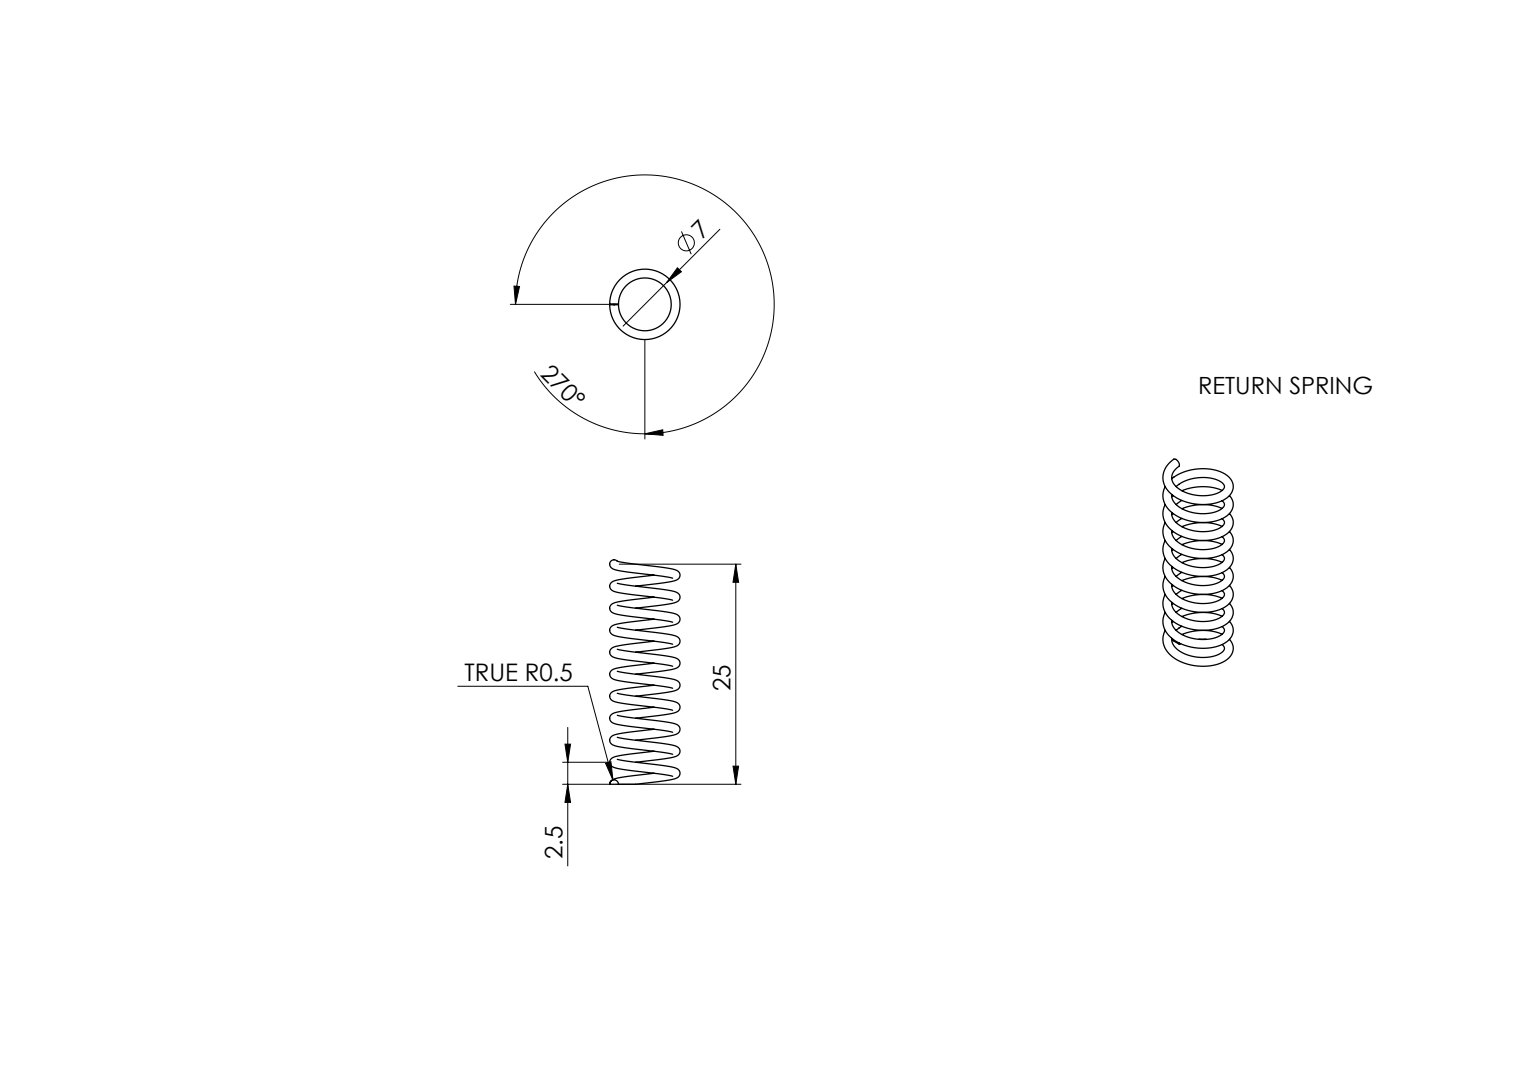
ISO-10303-21;
HEADER;
FILE_DESCRIPTION (('STEP AP214'),
    '1' );
FILE_NAME ('Return Spring.step',
    '2026-10-25T16:39:07',
    ( '' ),
    ( '' ),
    'SwSTEP 2.0',
    'SolidWorks 2026',
    '' );
FILE_SCHEMA (( 'AUTOMOTIVE_DESIGN' ));
ENDSEC;

DATA;
#1=CARTESIAN_POINT ( 'NONE',  ( 1.444289557195957086, 32.75319992234354061, -4.262301884875733471 ) ) ;
#6=CARTESIAN_POINT ( 'NONE',  ( 3.518350579753631191, 24.37180007765648071, 1.080741659609802285 ) ) ;
#9=CARTESIAN_POINT ( 'NONE',  ( -1.336863392178478716, 22.49680007765647360, 4.297206761780677731 ) ) ;
#14=CARTESIAN_POINT ( 'NONE',  ( -2.115076519116362519, 25.12180007765647360, 3.012182706137107147 ) ) ;
#21=CARTESIAN_POINT ( 'NONE',  ( 3.518350579753605434, 18.12819992234353705, -1.080741659609877114 ) ) ;
#23=CARTESIAN_POINT ( 'NONE',  ( -2.798362969681365886, 35.24680007765648071, 2.102939460078824929 ) ) ;
#24=CARTESIAN_POINT ( 'NONE',  ( 0.05938372350920109732, 27.62819992234353705, -3.680117784833935701 ) ) ;
#39=CARTESIAN_POINT ( 'NONE',  ( -2.518350579753611207, 21.87819992234354416, 0.7558219633769609480 ) ) ;
#47=CARTESIAN_POINT ( 'NONE',  ( 0.05938372350927906274, 32.37180007765647360, 3.680117784833935701 ) ) ;
#58=CARTESIAN_POINT ( 'NONE',  ( 2.055738996568313048, 21.99680007765648426, 1.423772053676023441 ) ) ;
#65=CARTESIAN_POINT ( 'NONE',  ( 0.8262555684460829442, 37.75319992234354771, -2.360188852285421302 ) ) ;
#69=CARTESIAN_POINT ( 'NONE',  ( 4.518350579753633411, 31.87180007765647716, 1.405661355842698468 ) ) ;
#87=CARTESIAN_POINT ( 'NONE',  ( 4.499999999999999112, 18.25319992234354771, 0.05647727720528474687 ) ) ;
#88=CARTESIAN_POINT ( 'NONE',  ( -2.115076519116425580, 27.37819992234354771, -3.012182706137063182 ) ) ;
#90=CARTESIAN_POINT ( 'NONE',  ( -1.593127413382998459, 35.87180007765648071, -2.091722143975139669 ) ) ;
#92=CARTESIAN_POINT ( 'NONE',  ( 2.733110507866328920, 36.12819992234354771, 3.862833514489095510 ) ) ;
#96=CARTESIAN_POINT ( 'NONE',  ( 2.798362969681366330, 18.99680007765648071, -2.102939460078824929 ) ) ;
#99=CARTESIAN_POINT ( 'NONE',  ( 4.518350579753633411, 21.87180007765647360, 1.405661355842698468 ) ) ;
#106=CARTESIAN_POINT ( 'NONE',  ( -3.500000000000000444, 22.99680007765647716, 0.05647727720536892260 ) ) ;
#111=CARTESIAN_POINT ( 'NONE',  ( -3.481649420246394122, 22.12819992234353705, -1.193696214020467883 ) ) ;
#113=CARTESIAN_POINT ( 'NONE',  ( 2.211161402132902243, 37.12180007765645939, 2.942372952327172442 ) ) ;
#114=CARTESIAN_POINT ( 'NONE',  ( 1.027846397803612311, 36.25319992234354771, 3.346150245485499219 ) ) ;
#126=CARTESIAN_POINT ( 'NONE',  ( -0.05938372350921170689, 21.37819992234354416, 2.628655560595669183 ) ) ;
#134=CARTESIAN_POINT ( 'NONE',  ( -0.05938372350927861171, 36.12180007765648782, -3.680117784833935701 ) ) ;
#147=CARTESIAN_POINT ( 'NONE',  ( 1.593127413382998903, 24.62180007765647716, 2.091722143975139669 ) ) ;
#149=CARTESIAN_POINT ( 'NONE',  ( 2.115076519116362963, 23.87180007765647360, -3.012182706137107591 ) ) ;
#154=CARTESIAN_POINT ( 'NONE',  ( -0.05938372350921170689, 33.87819992234354061, 2.628655560595669183 ) ) ;
#158=CARTESIAN_POINT ( 'NONE',  ( -3.607379964056306676, 35.24680007765647360, 2.690724712371306282 ) ) ;
#173=CARTESIAN_POINT ( 'NONE',  ( 2.733110507866328920, 21.12819992234354416, 3.862833514489095510 ) ) ;
#174=CARTESIAN_POINT ( 'NONE',  ( -2.211161402132838738, 26.62819992234354416, 2.942372952327218183 ) ) ;
#176=CARTESIAN_POINT ( 'NONE',  ( -1.989345975306426206, 40.24680007765648071, 1.515154207786343799 ) ) ;
#178=CARTESIAN_POINT ( 'NONE',  ( 0.05938372350919016857, 32.62819992234354771, -4.731580009072201776 ) ) ;
#182=CARTESIAN_POINT ( 'NONE',  ( -2.798362969681365886, 30.24680007765648071, 2.102939460078824929 ) ) ;
#187=CARTESIAN_POINT ( 'NONE',  ( 4.518350579753633411, 34.37180007765647360, 1.405661355842698468 ) ) ;
#191=CARTESIAN_POINT ( 'NONE',  ( -2.115076519116362519, 27.62180007765648071, 3.012182706137107147 ) ) ;
#197=CARTESIAN_POINT ( 'NONE',  ( 2.115076519116426024, 21.12819992234353705, 3.012182706137062294 ) ) ;
#200=CARTESIAN_POINT ( 'NONE',  ( -3.481649420246369697, 37.87180007765648071, 1.193696214020542490 ) ) ;
#202=CARTESIAN_POINT ( 'NONE',  ( -0.05938372350920063936, 31.37819992234354416, 3.680117784833935701 ) ) ;
#216=CARTESIAN_POINT ( 'NONE',  ( -1.086818808809129289, 15.00000000000000533, -3.240250934315705322 ) ) ;
#219=CARTESIAN_POINT ( 'NONE',  ( 0.8262555684460829442, 20.25319992234354771, -2.360188852285421302 ) ) ;
#222=CARTESIAN_POINT ( 'NONE',  ( -1.444289557196047014, 18.49680007765647360, -4.262301884875704161 ) ) ;
#229=CARTESIAN_POINT ( 'NONE',  ( -0.05938372350927861171, 31.12180007765647005, -3.680117784833935701 ) ) ;
#239=PLANE ( 'NONE',  #7419 ) ;
#242=CARTESIAN_POINT ( 'NONE',  ( 2.518350579753628971, 21.87180007765647360, 0.7558219633769073242 ) ) ;
#245=CARTESIAN_POINT ( 'NONE',  ( 0.05938372350927906967, 19.87180007765648071, 3.680117784833935701 ) ) ;
#249=CARTESIAN_POINT ( 'NONE',  ( 0.7188294034286553114, 33.75319992234354771, 2.395093729190349130 ) ) ;
#252=CARTESIAN_POINT ( 'NONE',  ( -2.733110507866247652, 32.62180007765647360, 3.862833514489154574 ) ) ;
#272=( NAMED_UNIT ( * ) SI_UNIT ( $, .STERADIAN. ) SOLID_ANGLE_UNIT ( ) );
#274=CARTESIAN_POINT ( 'NONE',  ( 3.607379964056363075, 18.50319992234354416, 2.690724712371229010 ) ) ;
#275=CARTESIAN_POINT ( 'NONE',  ( -2.864755990943222308, 26.75319992234354771, 2.011557305968548093 ) ) ;
#277=CARTESIAN_POINT ( 'NONE',  ( 2.518350579753628971, 34.37180007765647360, 0.7558219633769073242 ) ) ;
#279=CARTESIAN_POINT ( 'NONE',  ( 2.829195390882724759, 35.37819992234354061, -3.793023760679264278 ) ) ;
#284=CARTESIAN_POINT ( 'NONE',  ( 2.864755990943265829, 31.99680007765647716, 2.011557305968487697 ) ) ;
#289=CARTESIAN_POINT ( 'NONE',  ( -2.733110507866247652, 27.62180007765647716, 3.862833514489154574 ) ) ;
#293=CARTESIAN_POINT ( 'NONE',  ( 3.518350579753631191, 24.37180007765648071, 1.080741659609802285 ) ) ;
#298=CARTESIAN_POINT ( 'NONE',  ( -1.027846397803611866, 20.00319992234354416, -3.346150245485499219 ) ) ;
#301=CARTESIAN_POINT ( 'NONE',  ( 2.055738996568313048, 16.99680007765648071, 1.423772053676023441 ) ) ;
#303=CARTESIAN_POINT ( 'NONE',  ( 2.115076519116426024, 36.12819992234355482, 3.012182706137062294 ) ) ;
#318=CARTESIAN_POINT ( 'NONE',  ( 0.8262555684460829442, 17.75319992234354061, -2.360188852285421302 ) ) ;
#322=CARTESIAN_POINT ( 'NONE',  ( -1.336863392178478716, 17.49680007765647716, 4.297206761780677731 ) ) ;
#328=CARTESIAN_POINT ( 'NONE',  ( -2.864755990943265829, 38.24680007765647360, -2.011557305968488141 ) ) ;
#341=CARTESIAN_POINT ( 'NONE',  ( 0.7188294034286049072, 26.24680007765647716, -2.395093729190366005 ) ) ;
#344=CARTESIAN_POINT ( 'NONE',  ( 3.518350579753631191, 19.37180007765648071, 1.080741659609802729 ) ) ;
#348=CARTESIAN_POINT ( 'NONE',  ( -2.864755990943222308, 16.75319992234354416, 2.011557305968548093 ) ) ;
#351=CARTESIAN_POINT ( 'NONE',  ( -1.336863392178478716, 32.49680007765647360, 4.297206761780677731 ) ) ;
#360=ORIENTED_EDGE ( 'NONE', *, *, #444, .T. ) ;
#368=CARTESIAN_POINT ( 'NONE',  ( -3.607379964056363075, 24.75319992234354416, -2.690724712371229899 ) ) ;
#369=CARTESIAN_POINT ( 'NONE',  ( 2.798362969681409851, 26.00319992234354771, 2.102939460078764977 ) ) ;
#370=CARTESIAN_POINT ( 'NONE',  ( -2.518350579753611207, 19.37819992234354771, 0.7558219633769609480 ) ) ;
#372=CARTESIAN_POINT ( 'NONE',  ( -1.444289557195956863, 31.50319992234354416, 4.262301884875733471 ) ) ;
#379=EDGE_CURVE ( 'NONE', #12310, #9517, #6444, .T. ) ;
#380=CARTESIAN_POINT ( 'NONE',  ( 3.518350579753631191, 31.87180007765647716, 1.080741659609802285 ) ) ;
#384=CARTESIAN_POINT ( 'NONE',  ( 1.444289557196047680, 32.24680007765647360, 4.262301884875704161 ) ) ;
#388=CARTESIAN_POINT ( 'NONE',  ( 3.500000000000000444, 31.74680007765647716, -0.05647727720536935281 ) ) ;
#395=CARTESIAN_POINT ( 'NONE',  ( -2.211161402132839182, 26.62819992234353705, 2.942372952327218627 ) ) ;
#398=CARTESIAN_POINT ( 'NONE',  ( 3.481649420246369697, 36.62180007765648071, -1.193696214020541824 ) ) ;
#399=CARTESIAN_POINT ( 'NONE',  ( 3.518350579753605434, 33.12819992234354771, -1.080741659609877114 ) ) ;
#415=CARTESIAN_POINT ( 'NONE',  ( -0.05938372350921170689, 23.87819992234354416, 2.628655560595669183 ) ) ;
#417=CARTESIAN_POINT ( 'NONE',  ( 3.481649420246369697, 16.62180007765648071, -1.193696214020541824 ) ) ;
#422=CARTESIAN_POINT ( 'NONE',  ( 1.027846397803542144, 38.74680007765647360, -3.346150245485522312 ) ) ;
#424=DIRECTION ( 'NONE',  ( 1.027440012549754468E-14, -0.1129545544106655003, 0.9936001553129347741 ) ) ;
#431=CARTESIAN_POINT ( 'NONE',  ( -1.593127413382998459, 25.87180007765647716, -2.091722143975139669 ) ) ;
#433=CARTESIAN_POINT ( 'NONE',  ( 2.211161402132902243, 24.62180007765647716, 2.942372952327172442 ) ) ;
#437=CARTESIAN_POINT ( 'NONE',  ( -1.027846397803611866, 22.50319992234354416, -3.346150245485499219 ) ) ;
#441=CARTESIAN_POINT ( 'NONE',  ( -3.518350579753630747, 18.12180007765648071, -1.080741659609802729 ) ) ;
#444=EDGE_CURVE ( 'NONE', #6995, #13000, #16882, .T. ) ;
#460=CARTESIAN_POINT ( 'NONE',  ( -0.05938372350918959958, 28.87819992234354416, 4.731580009072201776 ) ) ;
#461=CARTESIAN_POINT ( 'NONE',  ( -2.115076519116425580, 24.87819992234354416, -3.012182706137063182 ) ) ;
#462=CARTESIAN_POINT ( 'NONE',  ( -2.500000000000001332, 22.00319992234354771, -0.05647727720530596601 ) ) ;
#464=CARTESIAN_POINT ( 'NONE',  ( -4.481649420246366589, 17.87180007765647360, 1.518615910253458878 ) ) ;
#468=CARTESIAN_POINT ( 'NONE',  ( 2.798362969681366330, 26.49680007765648071, -2.102939460078824929 ) ) ;
#471=CARTESIAN_POINT ( 'NONE',  ( -1.336863392178478716, 32.49680007765647360, 4.297206761780677731 ) ) ;
#475=CARTESIAN_POINT ( 'NONE',  ( 2.115076519116362963, 28.87180007765647716, -3.012182706137107147 ) ) ;
#480=( NAMED_UNIT ( * ) PLANE_ANGLE_UNIT ( ) SI_UNIT ( $, .RADIAN. ) );
#482=CARTESIAN_POINT ( 'NONE',  ( 0.05938372350920109732, 30.12819992234354416, -3.680117784833935701 ) ) ;
#486=CARTESIAN_POINT ( 'NONE',  ( 1.497042530366477164, 18.87180007765648071, -2.161531897785062384 ) ) ;
#487=CARTESIAN_POINT ( 'NONE',  ( 3.673772985318163098, 18.00319992234354416, -2.599342558261029001 ) ) ;
#504=CARTESIAN_POINT ( 'NONE',  ( -2.518350579753611207, 26.87819992234354416, 0.7558219633769609480 ) ) ;
#509=CARTESIAN_POINT ( 'NONE',  ( -2.798362969681365886, 20.24680007765647716, 2.102939460078824929 ) ) ;
#525=CARTESIAN_POINT ( 'NONE',  ( 1.497042530366477164, 33.87180007765647360, -2.161531897785062384 ) ) ;
#527=CARTESIAN_POINT ( 'NONE',  ( -2.115076519116362519, 25.12180007765647005, 3.012182706137108035 ) ) ;
#532=CARTESIAN_POINT ( 'NONE',  ( 1.027846397803612311, 18.75319992234354771, 3.346150245485499219 ) ) ;
#535=CARTESIAN_POINT ( 'NONE',  ( -2.864755990943265829, 18.24680007765648071, -2.011557305968488141 ) ) ;
#539=CLOSED_SHELL ( 'NONE', ( #14555, #17882, #8237, #2719, #9820 ) ) ;
#558=CARTESIAN_POINT ( 'NONE',  ( 4.499999999999999112, 23.25319992234354416, 0.05647727720528474687 ) ) ;
#559=CARTESIAN_POINT ( 'NONE',  ( -2.115076519116425580, 37.37819992234353350, -3.012182706137063182 ) ) ;
#561=CARTESIAN_POINT ( 'NONE',  ( -2.481649420246391902, 19.62819992234354416, -0.8687765177875723666 ) ) ;
#564=CARTESIAN_POINT ( 'NONE',  ( 3.673772985318219053, 19.49680007765647005, 2.599342558260951730 ) ) ;
#569=CARTESIAN_POINT ( 'NONE',  ( -3.481649420246369697, 32.87180007765645939, 1.193696214020542490 ) ) ;
#572=CARTESIAN_POINT ( 'NONE',  ( 4.518350579753633411, 29.37180007765647716, 1.405661355842698468 ) ) ;
#582=CARTESIAN_POINT ( 'NONE',  ( -3.500000000000000444, 24.50319992234354416, -0.05647727720529563400 ) ) ;
#585=CARTESIAN_POINT ( 'NONE',  ( 2.500000000000001332, 24.24680007765647716, -0.05647727720535888202 ) ) ;
#586=CARTESIAN_POINT ( 'NONE',  ( -3.673772985318163098, 16.75319992234354416, 2.599342558261029001 ) ) ;
#602=CARTESIAN_POINT ( 'NONE',  ( -1.497042530366522461, 27.37819992234355126, -2.161531897785030409 ) ) ;
#605=CARTESIAN_POINT ( 'NONE',  ( 0.05938372350927906274, 24.87180007765647005, 3.680117784833935701 ) ) ;
#622=CARTESIAN_POINT ( 'NONE',  ( -2.518350579753628526, 28.12180007765647716, -0.7558219633769075463 ) ) ;
#624=CARTESIAN_POINT ( 'NONE',  ( 2.211161402132902243, 27.12180007765647716, 2.942372952327172442 ) ) ;
#629=CARTESIAN_POINT ( 'NONE',  ( 3.481649420246394122, 20.87819992234354416, 1.193696214020467439 ) ) ;
#633=CARTESIAN_POINT ( 'NONE',  ( 3.500000000000000444, 16.74680007765647716, -0.05647727720536935281 ) ) ;
#650=CARTESIAN_POINT ( 'NONE',  ( -4.499999999999999112, 29.50319992234354061, -0.05647727720528529505 ) ) ;
#651=CARTESIAN_POINT ( 'NONE',  ( -2.115076519116425580, 32.37819992234354771, -3.012182706137063182 ) ) ;
#652=CARTESIAN_POINT ( 'NONE',  ( -0.05938372350921170689, 23.87819992234354416, 2.628655560595669183 ) ) ;
#655=CARTESIAN_POINT ( 'NONE',  ( -1.444289557196047014, 15.99680007765647716, -4.262301884875704161 ) ) ;
#659=CARTESIAN_POINT ( 'NONE',  ( 3.518350579753631191, 36.87180007765645939, 1.080741659609802285 ) ) ;
#672=CARTESIAN_POINT ( 'NONE',  ( -1.027846397803611866, 30.00319992234354416, -3.346150245485499219 ) ) ;
#675=CARTESIAN_POINT ( 'NONE',  ( 2.481649420246374138, 19.12180007765648071, -0.8687765177876252132 ) ) ;
#677=CARTESIAN_POINT ( 'NONE',  ( -2.829195390882724315, 21.62819992234354416, 3.793023760679264722 ) ) ;
#683=CARTESIAN_POINT ( 'NONE',  ( -4.499999999999999112, 37.99680007765646650, 0.05647727720537927543 ) ) ;
#696=CARTESIAN_POINT ( 'NONE',  ( 0.7188294034286553114, 26.25319992234354416, 2.395093729190349130 ) ) ;
#698=CARTESIAN_POINT ( 'NONE',  ( 1.135272562821090458, 19.74680007765648071, 3.311245368580554072 ) ) ;
#711=CARTESIAN_POINT ( 'NONE',  ( 1.497042530366477164, 28.87180007765648426, -2.161531897785062384 ) ) ;
#713=CARTESIAN_POINT ( 'NONE',  ( 1.027846397803542144, 31.24680007765647716, -3.346150245485522312 ) ) ;
#722=CARTESIAN_POINT ( 'NONE',  ( -1.336863392178478716, 39.99680007765647360, 4.297206761780677731 ) ) ;
#743=CARTESIAN_POINT ( 'NONE',  ( 3.673772985318163098, 25.50319992234354416, -2.599342558261029001 ) ) ;
#744=CARTESIAN_POINT ( 'NONE',  ( -2.211161402132838738, 39.12819992234354771, 2.942372952327218183 ) ) ;
#745=CARTESIAN_POINT ( 'NONE',  ( 1.593127413382953383, 17.87819992234354416, -2.091722143975172532 ) ) ;
#747=CARTESIAN_POINT ( 'NONE',  ( 1.444289557195957086, 37.75319992234354771, -4.262301884875733471 ) ) ;
#751=CARTESIAN_POINT ( 'NONE',  ( 3.518350579753631191, 34.37180007765648071, 1.080741659609802285 ) ) ;
#763=CARTESIAN_POINT ( 'NONE',  ( -1.027846397803611866, 25.00319992234354416, -3.346150245485499219 ) ) ;
#766=CARTESIAN_POINT ( 'NONE',  ( -2.518350579753628526, 25.62180007765648426, -0.7558219633769075463 ) ) ;
#767=CARTESIAN_POINT ( 'NONE',  ( 4.499999999999999112, 15.75319992234354416, 0.05647727720528474687 ) ) ;
#771=CARTESIAN_POINT ( 'NONE',  ( 1.027846397803542144, 16.24680007765647716, -3.346150245485522312 ) ) ;
#782=CARTESIAN_POINT ( 'NONE',  ( -2.481649420246391902, 29.62819992234354416, -0.8687765177875723666 ) ) ;
#784=CARTESIAN_POINT ( 'NONE',  ( -2.864755990943265829, 25.74680007765647716, -2.011557305968488141 ) ) ;
#791=DIRECTION ( 'NONE',  ( -1.028113302204112171E-14, 0.1129545544106649313, -0.9936001553129349961 ) ) ;
#799=CARTESIAN_POINT ( 'NONE',  ( -1.593127413382998459, 28.37180007765648426, -2.091722143975139669 ) ) ;
#801=CARTESIAN_POINT ( 'NONE',  ( 3.481649420246370141, 26.62180007765648071, -1.193696214020541602 ) ) ;
#805=CARTESIAN_POINT ( 'NONE',  ( -3.500000000000000444, 40.00000000000000711, 3.664603343001004987E-14 ) ) ;
#808=CARTESIAN_POINT ( 'NONE',  ( -3.518350579753630747, 25.62180007765648071, -1.080741659609802729 ) ) ;
#818=EDGE_CURVE ( 'NONE', #6875, #12310, #1742, .T. ) ;
#823=CARTESIAN_POINT ( 'NONE',  ( 3.500000000000000444, 34.24680007765648071, -0.05647727720536935281 ) ) ;
#829=CARTESIAN_POINT ( 'NONE',  ( 2.733110507866328920, 33.62819992234354771, 3.862833514489095510 ) ) ;
#830=CARTESIAN_POINT ( 'NONE',  ( 3.481649420246395010, 35.87819992234354061, 1.193696214020467439 ) ) ;
#831=CARTESIAN_POINT ( 'NONE',  ( 2.055738996568281518, 25.50319992234354416, -1.423772053676066518 ) ) ;
#833=CARTESIAN_POINT ( 'NONE',  ( 1.336863392178479160, 21.24680007765647716, -4.297206761780677731 ) ) ;
#839=CARTESIAN_POINT ( 'NONE',  ( 3.500000000000000444, 36.74680007765648071, -0.05647727720536935281 ) ) ;
#852=CARTESIAN_POINT ( 'NONE',  ( -2.798362969681409851, 34.75319992234354771, -2.102939460078765421 ) ) ;
#855=CARTESIAN_POINT ( 'NONE',  ( -2.518350579753628526, 18.12180007765648071, -0.7558219633769075463 ) ) ;
#856=CARTESIAN_POINT ( 'NONE',  ( -4.481649420246396787, 17.12819992234354416, -1.518615910253363399 ) ) ;
#860=CARTESIAN_POINT ( 'NONE',  ( 1.444289557196047680, 37.24680007765646650, 4.262301884875704161 ) ) ;
#868=CARTESIAN_POINT ( 'NONE',  ( 3.500000000000000444, 19.24680007765648071, -0.05647727720536935281 ) ) ;
#873=CARTESIAN_POINT ( 'NONE',  ( 0.8262555684460829442, 25.25319992234354771, -2.360188852285421302 ) ) ;
#876=CARTESIAN_POINT ( 'NONE',  ( 2.211161402132902243, 27.12180007765647360, 2.942372952327172442 ) ) ;
#884=CARTESIAN_POINT ( 'NONE',  ( -4.499999999999999112, 22.99680007765647716, 0.05647727720537927543 ) ) ;
#893=CARTESIAN_POINT ( 'NONE',  ( 2.518350579753628971, 29.37180007765648426, 0.7558219633769073242 ) ) ;
#895=CARTESIAN_POINT ( 'NONE',  ( 2.115076519116362963, 33.87180007765648071, -3.012182706137107591 ) ) ;
#900=ORIENTED_EDGE ( 'NONE', *, *, #12146, .T. ) ;
#902=CARTESIAN_POINT ( 'NONE',  ( -2.864755990943265829, 25.74680007765647716, -2.011557305968488141 ) ) ;
#915=CARTESIAN_POINT ( 'NONE',  ( -1.027846397803541700, 29.99680007765648071, 3.346150245485522312 ) ) ;
#920=CARTESIAN_POINT ( 'NONE',  ( 4.518350579753602325, 33.12819992234354771, -1.405661355842793725 ) ) ;
#921=CARTESIAN_POINT ( 'NONE',  ( -3.500000000000000444, 37.00319992234354061, -0.05647727720529563400 ) ) ;
#922=CARTESIAN_POINT ( 'NONE',  ( -1.989345975306457071, 29.75319992234354771, -1.515154207786300944 ) ) ;
#924=CARTESIAN_POINT ( 'NONE',  ( 4.481649420246366589, 21.62180007765647716, -1.518615910253458212 ) ) ;
#929=CARTESIAN_POINT ( 'NONE',  ( -3.518350579753630747, 35.62180007765648782, -1.080741659609802729 ) ) ;
#936=PRODUCT_DEFINITION_CONTEXT ( 'detailed design', #5355, 'design' ) ;
#941=CARTESIAN_POINT ( 'NONE',  ( 3.481649420246394122, 35.87819992234353350, 1.193696214020467439 ) ) ;
#944=CARTESIAN_POINT ( 'NONE',  ( -0.8262555684461330152, 30.99680007765647716, -2.360188852285403982 ) ) ;
#946=CARTESIAN_POINT ( 'NONE',  ( -1.336863392178569088, 27.50319992234354771, -4.297206761780648421 ) ) ;
#954=CARTESIAN_POINT ( 'NONE',  ( 2.733110507866247652, 36.37180007765647360, -3.862833514489153686 ) ) ;
#963=CARTESIAN_POINT ( 'NONE',  ( -1.135272562821090014, 18.49680007765648071, -3.311245368580554072 ) ) ;
#970=CARTESIAN_POINT ( 'NONE',  ( -1.027846397803611866, 15.00319992234354594, -3.346150245485499219 ) ) ;
#972=CARTESIAN_POINT ( 'NONE',  ( 2.115076519116362963, 31.37180007765647716, -3.012182706137107147 ) ) ;
#973=CARTESIAN_POINT ( 'NONE',  ( 3.500000000000000444, 20.75319992234354416, 0.05647727720529520379 ) ) ;
#974=CARTESIAN_POINT ( 'NONE',  ( 2.798362969681409851, 18.50319992234354771, 2.102939460078764977 ) ) ;
#980=CARTESIAN_POINT ( 'NONE',  ( -2.829195390882805139, 23.37180007765647716, -3.793023760679206102 ) ) ;
#987=CARTESIAN_POINT ( 'NONE',  ( -1.989345975306426206, 40.24680007765648071, 1.515154207786343799 ) ) ;
#989=CARTESIAN_POINT ( 'NONE',  ( -2.798362969681365886, 27.74680007765648071, 2.102939460078824929 ) ) ;
#997=CARTESIAN_POINT ( 'NONE',  ( -2.798362969681365886, 27.74680007765648071, 2.102939460078824929 ) ) ;
#1009=CARTESIAN_POINT ( 'NONE',  ( -1.027846397803541700, 34.99680007765648071, 3.346150245485522312 ) ) ;
#1013=CARTESIAN_POINT ( 'NONE',  ( 2.829195390882724759, 30.37819992234354061, -3.793023760679264278 ) ) ;
#1015=CARTESIAN_POINT ( 'NONE',  ( 2.500000000000001332, 25.75319992234354771, 0.05647727720530566764 ) ) ;
#1018=CARTESIAN_POINT ( 'NONE',  ( -1.444289557196047014, 23.49680007765647716, -4.262301884875704161 ) ) ;
#1023=CARTESIAN_POINT ( 'NONE',  ( 2.864755990943265829, 34.49680007765648071, 2.011557305968487697 ) ) ;
#1033=CARTESIAN_POINT ( 'NONE',  ( -0.05938372350920063936, 33.87819992234354771, 3.680117784833935701 ) ) ;
#1034=CARTESIAN_POINT ( 'NONE',  ( -0.05938372350920064630, 21.37819992234354061, 3.680117784833935701 ) ) ;
#1036=CARTESIAN_POINT ( 'NONE',  ( 1.989345975306426206, 31.49680007765648071, -1.515154207786343799 ) ) ;
#1037=CARTESIAN_POINT ( 'NONE',  ( 4.499999999999999112, 23.25319992234354416, 0.05647727720528474687 ) ) ;
#1043=CARTESIAN_POINT ( 'NONE',  ( -4.481649420246366589, 35.37180007765647360, 1.518615910253458878 ) ) ;
#1059=CARTESIAN_POINT ( 'NONE',  ( 1.593127413382953383, 32.87819992234354771, -2.091722143975172532 ) ) ;
#1061=CARTESIAN_POINT ( 'NONE',  ( -2.798362969681365886, 32.74680007765648071, 2.102939460078824929 ) ) ;
#1062=CARTESIAN_POINT ( 'NONE',  ( -3.518350579753605434, 24.37819992234353705, 1.080741659609877781 ) ) ;
#1067=CARTESIAN_POINT ( 'NONE',  ( -3.500000000000000444, 15.00000000000001243, 3.664603343001004987E-14 ) ) ;
#1068=CARTESIAN_POINT ( 'NONE',  ( -4.481649420246366589, 22.87180007765647360, 1.518615910253458878 ) ) ;
#1076=CARTESIAN_POINT ( 'NONE',  ( -2.481649420246391902, 14.62819992234354594, -0.8687765177875723666 ) ) ;
#1085=CARTESIAN_POINT ( 'NONE',  ( -3.481649420246369697, 27.87180007765647360, 1.193696214020542490 ) ) ;
#1096=CARTESIAN_POINT ( 'NONE',  ( 2.518350579753628971, 16.87180007765648071, 0.7558219633769073242 ) ) ;
#1100=CARTESIAN_POINT ( 'NONE',  ( -2.829195390882724315, 36.62819992234354771, 3.793023760679264722 ) ) ;
#1103=CARTESIAN_POINT ( 'NONE',  ( 0.05938372350921204690, 27.62819992234354416, -2.628655560595669183 ) ) ;
#1106=CARTESIAN_POINT ( 'NONE',  ( 4.499999999999999112, 24.24680007765647716, -0.05647727720537982360 ) ) ;
#1123=CARTESIAN_POINT ( 'NONE',  ( -2.115076519116362519, 17.62180007765647716, 3.012182706137108035 ) ) ;
#1126=CARTESIAN_POINT ( 'NONE',  ( -3.518350579753605434, 34.37819992234354771, 1.080741659609877781 ) ) ;
#1127=CARTESIAN_POINT ( 'NONE',  ( -1.135272562821019626, 24.00319992234354416, 3.311245368580577164 ) ) ;
#1129=CARTESIAN_POINT ( 'NONE',  ( -0.7188294034286043521, 32.49680007765648782, 2.395093729190366005 ) ) ;
#1130=CARTESIAN_POINT ( 'NONE',  ( 4.481649420246397675, 28.37819992234355126, 1.518615910253363177 ) ) ;
#1135=CARTESIAN_POINT ( 'NONE',  ( -2.211161402132902243, 25.87180007765647360, -2.942372952327172886 ) ) ;
#1144=CARTESIAN_POINT ( 'NONE',  ( 2.798362969681366330, 16.49680007765647716, -2.102939460078824929 ) ) ;
#1148=CARTESIAN_POINT ( 'NONE',  ( 1.593127413382953383, 37.87819992234354771, -2.091722143975172532 ) ) ;
#1150=CARTESIAN_POINT ( 'NONE',  ( 2.798362969681366330, 28.99680007765647716, -2.102939460078824929 ) ) ;
#1152=CARTESIAN_POINT ( 'NONE',  ( 1.027846397803612311, 28.75319992234354416, 3.346150245485499219 ) ) ;
#1161=DIRECTION ( 'NONE',  ( 0.000000000000000000, 0.9936001553129348851, 0.1129545544106647231 ) ) ;
#1167=CARTESIAN_POINT ( 'NONE',  ( -0.7188294034286043521, 39.99680007765647360, 2.395093729190366005 ) ) ;
#1169=CARTESIAN_POINT ( 'NONE',  ( 2.115076519116362963, 36.37180007765648071, -3.012182706137107591 ) ) ;
#1171=CARTESIAN_POINT ( 'NONE',  ( -1.244399073187948845, 15.00000000000001243, -3.410710356087081063 ) ) ;
#1175=CARTESIAN_POINT ( 'NONE',  ( 2.864755990943265829, 24.49680007765647716, 2.011557305968487697 ) ) ;
#1191=CARTESIAN_POINT ( 'NONE',  ( 1.027846397803542144, 38.74680007765647360, -3.346150245485522312 ) ) ;
#1196=CARTESIAN_POINT ( 'NONE',  ( -2.733110507866328476, 32.37819992234353350, -3.862833514489096398 ) ) ;
#1199=CARTESIAN_POINT ( 'NONE',  ( -2.518350579753611207, 31.87819992234354416, 0.7558219633769609480 ) ) ;
#1202=CARTESIAN_POINT ( 'NONE',  ( -4.499999999999999112, 27.99680007765647716, 0.05647727720537927543 ) ) ;
#1218=CARTESIAN_POINT ( 'NONE',  ( 3.518350579753605434, 38.12819992234354061, -1.080741659609877114 ) ) ;
#1219=CARTESIAN_POINT ( 'NONE',  ( 2.798362969681409851, 21.00319992234354416, 2.102939460078764977 ) ) ;
#1221=CARTESIAN_POINT ( 'NONE',  ( 1.989345975306426206, 33.99680007765647360, -1.515154207786343799 ) ) ;
#1223=CARTESIAN_POINT ( 'NONE',  ( 0.05938372350919016857, 27.62819992234354416, -4.731580009072201776 ) ) ;
#1229=CARTESIAN_POINT ( 'NONE',  ( 3.481649420246369697, 21.62180007765647360, -1.193696214020541824 ) ) ;
#1238=CARTESIAN_POINT ( 'NONE',  ( 2.211161402132902243, 17.12180007765648071, 2.942372952327172442 ) ) ;
#1243=CARTESIAN_POINT ( 'NONE',  ( -0.8262555684460826111, 36.50319992234354061, 2.360188852285421302 ) ) ;
#1245=CARTESIAN_POINT ( 'NONE',  ( -3.481649420246369697, 30.37180007765647005, 1.193696214020542490 ) ) ;
#1246=CARTESIAN_POINT ( 'NONE',  ( -3.481649420246394122, 24.62819992234354061, -1.193696214020467883 ) ) ;
#1261=CARTESIAN_POINT ( 'NONE',  ( 2.055738996568281518, 15.50319992234354949, -1.423772053676066518 ) ) ;
#1263=CARTESIAN_POINT ( 'NONE',  ( -1.027846397803541700, 39.99680007765648071, 3.346150245485522312 ) ) ;
#1265=CARTESIAN_POINT ( 'NONE',  ( -1.089585269739795192, 15.00000000000000533, -3.377979775708401355 ) ) ;
#1269=CARTESIAN_POINT ( 'NONE',  ( -3.481649420246369697, 35.37180007765648071, 1.193696214020542490 ) ) ;
#1283=CARTESIAN_POINT ( 'NONE',  ( -3.518350579753630747, 38.12180007765648071, -1.080741659609802729 ) ) ;
#1288=CARTESIAN_POINT ( 'NONE',  ( 1.336863392178479160, 16.24680007765647716, -4.297206761780677731 ) ) ;
#1290=CARTESIAN_POINT ( 'NONE',  ( -2.518350579753611207, 39.37819992234354771, 0.7558219633769609480 ) ) ;
#1294=CARTESIAN_POINT ( 'NONE',  ( -4.499999999999999112, 22.99680007765647716, 0.05647727720537927543 ) ) ;
#1309=FILL_AREA_STYLE_COLOUR ( '', #16948 ) ;
#1310=CARTESIAN_POINT ( 'NONE',  ( 2.733110507866328920, 18.62819992234354771, 3.862833514489095510 ) ) ;
#1311=CARTESIAN_POINT ( 'NONE',  ( -2.115076519116425580, 22.37819992234354061, -3.012182706137063182 ) ) ;
#1313=CARTESIAN_POINT ( 'NONE',  ( -0.8262555684461330152, 28.49680007765648071, -2.360188852285403982 ) ) ;
#1314=CARTESIAN_POINT ( 'NONE',  ( -4.499999999999999112, 27.00319992234355126, -0.05647727720528529505 ) ) ;
#1318=CARTESIAN_POINT ( 'NONE',  ( -3.518350579753630747, 23.12180007765647716, -1.080741659609802729 ) ) ;
#1328=CARTESIAN_POINT ( 'NONE',  ( -3.481649420246369697, 22.87180007765647360, 1.193696214020542490 ) ) ;
#1333=CARTESIAN_POINT ( 'NONE',  ( 0.05938372350921204690, 37.62819992234354771, -2.628655560595669183 ) ) ;
#1335=CARTESIAN_POINT ( 'NONE',  ( 2.115076519116362963, 28.87180007765647716, -3.012182706137107147 ) ) ;
#1336=CARTESIAN_POINT ( 'NONE',  ( -3.518350579753605434, 26.87819992234354416, 1.080741659609877781 ) ) ;
#1344=CARTESIAN_POINT ( 'NONE',  ( -2.013855872281842707, 15.00000000000000533, -2.423565815785008404 ) ) ;
#1347=CARTESIAN_POINT ( 'NONE',  ( 1.593127413382953383, 15.37819992234354594, -2.091722143975172532 ) ) ;
#1350=CARTESIAN_POINT ( 'NONE',  ( -3.481649420246370141, 37.87180007765647360, 1.193696214020542268 ) ) ;
#1355=CARTESIAN_POINT ( 'NONE',  ( -1.135272562821090014, 33.49680007765648071, -3.311245368580554072 ) ) ;
#1367=CARTESIAN_POINT ( 'NONE',  ( 1.135272562821090458, 39.74680007765648071, 3.311245368580554072 ) ) ;
#1371=CARTESIAN_POINT ( 'NONE',  ( -0.05938372350928957516, 16.12180007765647716, -4.731580009072201776 ) ) ;
#1374=CARTESIAN_POINT ( 'NONE',  ( -2.518350579753611207, 36.87819992234354061, 0.7558219633769609480 ) ) ;
#1378=CARTESIAN_POINT ( 'NONE',  ( 4.499999999999999112, 34.24680007765646650, -0.05647727720537982360 ) ) ;
#1396=CARTESIAN_POINT ( 'NONE',  ( 4.518350579753602325, 15.62819992234354238, -1.405661355842793725 ) ) ;
#1397=CARTESIAN_POINT ( 'NONE',  ( -2.211161402132838738, 16.62819992234354416, 2.942372952327218183 ) ) ;
#1399=CARTESIAN_POINT ( 'NONE',  ( -1.497042530366477164, 35.12180007765647360, 2.161531897785062384 ) ) ;
#1400=CARTESIAN_POINT ( 'NONE',  ( -3.607379964056363075, 37.25319992234354061, -2.690724712371229899 ) ) ;
#1408=CARTESIAN_POINT ( 'NONE',  ( 3.518350579753631191, 21.87180007765647360, 1.080741659609802285 ) ) ;
#1411=CARTESIAN_POINT ( 'NONE',  ( -4.518350579753632523, 25.62180007765648426, -1.405661355842698468 ) ) ;
#1417=CARTESIAN_POINT ( 'NONE',  ( 3.500000000000000444, 21.74680007765647716, -0.05647727720536935281 ) ) ;
#1424=CARTESIAN_POINT ( 'NONE',  ( 0.05938372350920109732, 17.62819992234354771, -3.680117784833935701 ) ) ;
#1427=CARTESIAN_POINT ( 'NONE',  ( -2.518350579753628526, 15.62180007765648071, -0.7558219633769075463 ) ) ;
#1428=CARTESIAN_POINT ( 'NONE',  ( 2.115076519116426024, 23.62819992234354416, 3.012182706137062294 ) ) ;
#1438=CARTESIAN_POINT ( 'NONE',  ( -1.074071013978619593, 15.00000000000066258, -3.257214625843751321 ) ) ;
#1440=CARTESIAN_POINT ( 'NONE',  ( -2.518350579753611207, 19.37819992234354771, 0.7558219633769609480 ) ) ;
#1442=CARTESIAN_POINT ( 'NONE',  ( -0.05938372350927861865, 36.12180007765648071, -3.680117784833935701 ) ) ;
#1448=CARTESIAN_POINT ( 'NONE',  ( -2.115076519116362519, 30.12180007765647360, 3.012182706137107147 ) ) ;
#1461=CARTESIAN_POINT ( 'NONE',  ( -3.500000000000000444, 40.49680007765648071, 0.05647727720536892260 ) ) ;
#1467=CARTESIAN_POINT ( 'NONE',  ( -2.055738996568281518, 34.25319992234354061, 1.423772053676066962 ) ) ;
#1471=CARTESIAN_POINT ( 'NONE',  ( -2.733110507866247652, 30.12180007765647716, 3.862833514489154574 ) ) ;
#1484=CARTESIAN_POINT ( 'NONE',  ( -1.444289557195956863, 21.50319992234354771, 4.262301884875733471 ) ) ;
#1485=CARTESIAN_POINT ( 'NONE',  ( -2.864755990943222308, 29.25319992234354416, 2.011557305968548093 ) ) ;
#1487=CARTESIAN_POINT ( 'NONE',  ( -2.055738996568313048, 38.24680007765647360, -1.423772053676023441 ) ) ;
#1488=CARTESIAN_POINT ( 'NONE',  ( 0.05938372350919016857, 35.12819992234354771, -4.731580009072201776 ) ) ;
#1493=CARTESIAN_POINT ( 'NONE',  ( -3.518350579753630747, 20.62180007765646650, -1.080741659609802729 ) ) ;
#1496=CARTESIAN_POINT ( 'NONE',  ( 4.518350579753633411, 24.37180007765647005, 1.405661355842698468 ) ) ;
#1501=CARTESIAN_POINT ( 'NONE',  ( -3.500000000000000444, 25.49680007765647716, 0.05647727720536892260 ) ) ;
#1508=CARTESIAN_POINT ( 'NONE',  ( 3.481649420246394122, 20.87819992234354416, 1.193696214020467439 ) ) ;
#1511=CARTESIAN_POINT ( 'NONE',  ( -0.7188294034286043521, 17.49680007765647716, 2.395093729190366005 ) ) ;
#1513=CARTESIAN_POINT ( 'NONE',  ( -2.115076519116425580, 32.37819992234354771, -3.012182706137062738 ) ) ;
#1528=CARTESIAN_POINT ( 'NONE',  ( -0.8262555684460826111, 16.50319992234354416, 2.360188852285421302 ) ) ;
#1530=CARTESIAN_POINT ( 'NONE',  ( 2.115076519116362963, 18.87180007765648071, -3.012182706137107147 ) ) ;
#1536=CARTESIAN_POINT ( 'NONE',  ( 1.135272562821090458, 29.74680007765647716, 3.311245368580554072 ) ) ;
#1541=( GEOMETRIC_REPRESENTATION_CONTEXT ( 3 ) GLOBAL_UNCERTAINTY_ASSIGNED_CONTEXT ( ( #5473 ) ) GLOBAL_UNIT_ASSIGNED_CONTEXT ( ( #13339, #1764, #272 ) ) REPRESENTATION_CONTEXT ( 'NONE', 'WORKASPACE' ) );
#1547=CARTESIAN_POINT ( 'NONE',  ( -1.593127413382998459, 20.87180007765648426, -2.091722143975139669 ) ) ;
#1549=CARTESIAN_POINT ( 'NONE',  ( 3.500000000000000444, 21.74680007765647716, -0.05647727720536935281 ) ) ;
#1552=CARTESIAN_POINT ( 'NONE',  ( 0.8262555684460829442, 32.75319992234354061, -2.360188852285421302 ) ) ;
#1557=CARTESIAN_POINT ( 'NONE',  ( -2.829195390882805139, 30.87180007765647716, -3.793023760679206102 ) ) ;
#1568=CARTESIAN_POINT ( 'NONE',  ( -4.518350579753602325, 16.87819992234354416, 1.405661355842794391 ) ) ;
#1574=CARTESIAN_POINT ( 'NONE',  ( -4.499999999999999112, 19.50319992234354416, -0.05647727720528529505 ) ) ;
#1575=CARTESIAN_POINT ( 'NONE',  ( 2.798362969681409851, 28.50319992234354416, 2.102939460078764977 ) ) ;
#1577=CARTESIAN_POINT ( 'NONE',  ( -0.8262555684461330152, 35.99680007765648071, -2.360188852285403982 ) ) ;
#1580=CARTESIAN_POINT ( 'NONE',  ( 4.481649420246397675, 35.87819992234354771, 1.518615910253363177 ) ) ;
#1585=CARTESIAN_POINT ( 'NONE',  ( 2.115076519116362963, 26.37180007765648071, -3.012182706137107147 ) ) ;
#1589=CARTESIAN_POINT ( 'NONE',  ( -0.05938372350928957516, 33.62180007765647360, -4.731580009072201776 ) ) ;
#1593=CARTESIAN_POINT ( 'NONE',  ( 1.135272562821090458, 27.24680007765648071, 3.311245368580554072 ) ) ;
#1598=CARTESIAN_POINT ( 'NONE',  ( -2.115076519116425580, 19.87819992234354416, -3.012182706137062738 ) ) ;
#1600=CARTESIAN_POINT ( 'NONE',  ( -2.211161402132902243, 38.37180007765648071, -2.942372952327172886 ) ) ;
#1601=CARTESIAN_POINT ( 'NONE',  ( -2.211161402132839182, 31.62819992234354416, 2.942372952327218627 ) ) ;
#1616=CARTESIAN_POINT ( 'NONE',  ( 1.989345975306457071, 18.50319992234354416, 1.515154207786300500 ) ) ;
#1623=CARTESIAN_POINT ( 'NONE',  ( 2.115076519116362963, 36.37180007765648782, -3.012182706137107147 ) ) ;
#1635=CARTESIAN_POINT ( 'NONE',  ( 0.05938372350926800214, 19.87180007765648426, 2.628655560595669183 ) ) ;
#1637=CARTESIAN_POINT ( 'NONE',  ( -2.864755990943265829, 25.74680007765647716, -2.011557305968488141 ) ) ;
#1641=CARTESIAN_POINT ( 'NONE',  ( -1.593127413382952939, 34.12819992234354771, 2.091722143975172532 ) ) ;
#1645=CARTESIAN_POINT ( 'NONE',  ( 3.607379964056306676, 36.49680007765646650, -2.690724712371305838 ) ) ;
#1663=CARTESIAN_POINT ( 'NONE',  ( -4.499999999999999112, 14.50319992234354594, -0.05647727720528529505 ) ) ;
#1664=CARTESIAN_POINT ( 'NONE',  ( 3.500000000000000444, 25.75319992234354771, 0.05647727720529520379 ) ) ;
#1666=CARTESIAN_POINT ( 'NONE',  ( -2.500000000000001332, 14.50319992234354771, -0.05647727720530596601 ) ) ;
#1668=CARTESIAN_POINT ( 'NONE',  ( 3.673772985318163098, 35.50319992234354771, -2.599342558261029001 ) ) ;
#1674=CARTESIAN_POINT ( 'NONE',  ( -1.135272562821090014, 33.49680007765648071, -3.311245368580554072 ) ) ;
#1679=CARTESIAN_POINT ( 'NONE',  ( -4.481649420246366589, 30.37180007765647716, 1.518615910253458878 ) ) ;
#1683=CARTESIAN_POINT ( 'NONE',  ( 2.864755990943265829, 21.99680007765647716, 2.011557305968487697 ) ) ;
#1689=CARTESIAN_POINT ( 'NONE',  ( 2.864755990943222308, 18.00319992234354771, -2.011557305968548093 ) ) ;
#1692=CARTESIAN_POINT ( 'NONE',  ( 1.593127413382998903, 17.12180007765648426, 2.091722143975139669 ) ) ;
#1694=CARTESIAN_POINT ( 'NONE',  ( 2.115076519116426024, 33.62819992234353350, 3.012182706137062294 ) ) ;
#1711=CARTESIAN_POINT ( 'NONE',  ( -2.055738996568281518, 16.75319992234354416, 1.423772053676066962 ) ) ;
#1714=CARTESIAN_POINT ( 'NONE',  ( -4.518350579753632523, 15.62180007765647360, -1.405661355842698468 ) ) ;
#1719=CARTESIAN_POINT ( 'NONE',  ( 3.500000000000000444, 36.74680007765648071, -0.05647727720536935281 ) ) ;
#1732=CARTESIAN_POINT ( 'NONE',  ( 0.7188294034286049072, 21.24680007765648426, -2.395093729190366005 ) ) ;
#1735=CARTESIAN_POINT ( 'NONE',  ( 3.481649420246370141, 19.12180007765648071, -1.193696214020541602 ) ) ;
#1739=CARTESIAN_POINT ( 'NONE',  ( -2.798362969681409851, 17.25319992234354416, -2.102939460078765421 ) ) ;
#1742=B_SPLINE_CURVE_WITH_KNOTS ( 'NONE', 3,
 ( #7246, #5865, #17304, #1438, #216, #12735, #11513, #4476, #11331, #14401, #10119, #1344, #15801, #17024, #2913, #8546, #6976, #14221, #12638, #16933 ),
 .UNSPECIFIED., .F., .F.,
 ( 4, 2, 2, 2, 2, 2, 2, 2, 2, 4 ),
 ( 0.004985757390083797244, 0.005047933101378701548, 0.005110108812673605852, 0.005234460235263413592, 0.005483163080443029073, 0.005980568770802258301, 0.006975380151520719357, 0.007970191532239179547, 0.008467597222598410509, 0.008965002912957639736 ),
 .UNSPECIFIED. ) ;
#1745=CARTESIAN_POINT ( 'NONE',  ( -4.499999999999999112, 32.99680007765648071, 0.05647727720537927543 ) ) ;
#1764=( NAMED_UNIT ( * ) PLANE_ANGLE_UNIT ( ) SI_UNIT ( $, .RADIAN. ) );
#1766=CARTESIAN_POINT ( 'NONE',  ( -2.733110507866328476, 29.87819992234354416, -3.862833514489096398 ) ) ;
#1767=CARTESIAN_POINT ( 'NONE',  ( 3.481649420246395010, 30.87819992234354061, 1.193696214020467439 ) ) ;
#1769=CARTESIAN_POINT ( 'NONE',  ( 2.055738996568313048, 39.49680007765648071, 1.423772053676023441 ) ) ;
#1771=CARTESIAN_POINT ( 'NONE',  ( 0.05938372350919016857, 37.62819992234354771, -4.731580009072201776 ) ) ;
#1776=CARTESIAN_POINT ( 'NONE',  ( -0.05938372350927861171, 26.12180007765647005, -3.680117784833935701 ) ) ;
#1780=CARTESIAN_POINT ( 'NONE',  ( 2.733110507866247652, 31.37180007765647716, -3.862833514489153686 ) ) ;
#1783=CARTESIAN_POINT ( 'NONE',  ( 1.027846397803542144, 31.24680007765647716, -3.346150245485522312 ) ) ;
#1788=CARTESIAN_POINT ( 'NONE',  ( 2.115076519116426024, 16.12819992234354416, 3.012182706137062294 ) ) ;
#1791=CARTESIAN_POINT ( 'NONE',  ( -1.593127413382998459, 15.87180007765648071, -2.091722143975139669 ) ) ;
#1792=CARTESIAN_POINT ( 'NONE',  ( 3.481649420246394122, 35.87819992234353350, 1.193696214020467439 ) ) ;
#1807=CARTESIAN_POINT ( 'NONE',  ( -0.05938372350921170689, 18.87819992234354416, 2.628655560595669183 ) ) ;
#1815=CARTESIAN_POINT ( 'NONE',  ( 2.864755990943265829, 36.99680007765648071, 2.011557305968487697 ) ) ;
#1826=CARTESIAN_POINT ( 'NONE',  ( 1.497042530366477164, 21.37180007765648071, -2.161531897785062384 ) ) ;
#1828=CARTESIAN_POINT ( 'NONE',  ( -3.518350579753630303, 23.12180007765647716, -1.080741659609802952 ) ) ;
#1833=CARTESIAN_POINT ( 'NONE',  ( -2.798362969681409851, 22.25319992234354416, -2.102939460078765421 ) ) ;
#1836=CARTESIAN_POINT ( 'NONE',  ( 4.481649420246366589, 39.12180007765647360, -1.518615910253458212 ) ) ;
#1860=CARTESIAN_POINT ( 'NONE',  ( 4.518350579753602325, 28.12819992234354416, -1.405661355842793725 ) ) ;
#1861=CARTESIAN_POINT ( 'NONE',  ( 3.500000000000000444, 28.25319992234354416, 0.05647727720529520379 ) ) ;
#1862=CARTESIAN_POINT ( 'NONE',  ( -0.05938372350921170689, 21.37819992234354416, 2.628655560595669183 ) ) ;
#1865=CARTESIAN_POINT ( 'NONE',  ( -0.05938372350928957516, 18.62180007765647716, -4.731580009072201776 ) ) ;
#1871=CARTESIAN_POINT ( 'NONE',  ( 1.135272562821090458, 29.74680007765647716, 3.311245368580554072 ) ) ;
#1875=CARTESIAN_POINT ( 'NONE',  ( -4.518350579753632523, 33.12180007765647360, -1.405661355842698468 ) ) ;
#1878=CARTESIAN_POINT ( 'NONE',  ( 0.05938372350927906274, 29.87180007765648071, 3.680117784833935701 ) ) ;
#1886=CARTESIAN_POINT ( 'NONE',  ( 2.798362969681409851, 28.50319992234354416, 2.102939460078764977 ) ) ;
#1889=CARTESIAN_POINT ( 'NONE',  ( -1.989345975306426206, 20.24680007765648071, 1.515154207786343799 ) ) ;
#1890=CARTESIAN_POINT ( 'NONE',  ( -1.027846397803611866, 32.50319992234354771, -3.346150245485499219 ) ) ;
#1907=CARTESIAN_POINT ( 'NONE',  ( -2.518350579753611207, 29.37819992234355126, 0.7558219633769609480 ) ) ;
#1909=CARTESIAN_POINT ( 'NONE',  ( -3.500000000000000444, 17.99680007765647716, 0.05647727720536892260 ) ) ;
#1915=CARTESIAN_POINT ( 'NONE',  ( 2.798362969681366330, 36.49680007765648071, -2.102939460078824929 ) ) ;
#1929=CARTESIAN_POINT ( 'NONE',  ( 2.481649420246374138, 34.12180007765647360, -0.8687765177876252132 ) ) ;
#1931=CARTESIAN_POINT ( 'NONE',  ( 0.05938372350927906967, 24.87180007765647360, 3.680117784833935701 ) ) ;
#1936=CARTESIAN_POINT ( 'NONE',  ( 3.518350579753605434, 15.62819992234354416, -1.080741659609877114 ) ) ;
#1939=CARTESIAN_POINT ( 'NONE',  ( -3.481649420246369697, 20.37180007765647716, 1.193696214020542490 ) ) ;
#1956=CARTESIAN_POINT ( 'NONE',  ( 3.673772985318163098, 23.00319992234354416, -2.599342558261029001 ) ) ;
#1957=CARTESIAN_POINT ( 'NONE',  ( 2.798362969681409851, 36.00319992234354771, 2.102939460078764977 ) ) ;
#1958=CARTESIAN_POINT ( 'NONE',  ( 2.518350579753611207, 18.12819992234354416, -0.7558219633769606149 ) ) ;
#1960=CARTESIAN_POINT ( 'NONE',  ( -2.733110507866247652, 17.62180007765648071, 3.862833514489154574 ) ) ;
#1965=CARTESIAN_POINT ( 'NONE',  ( 2.115076519116362963, 31.37180007765647716, -3.012182706137107147 ) ) ;
#1969=CARTESIAN_POINT ( 'NONE',  ( 1.336863392178479160, 33.74680007765647360, -4.297206761780677731 ) ) ;
#1973=CARTESIAN_POINT ( 'NONE',  ( -0.05938372350927861171, 33.62180007765648071, -3.680117784833935701 ) ) ;
#1977=CARTESIAN_POINT ( 'NONE',  ( 1.135272562821020070, 25.25319992234354416, -3.311245368580577164 ) ) ;
#1980=CARTESIAN_POINT ( 'NONE',  ( 1.989345975306426206, 21.49680007765648071, -1.515154207786343799 ) ) ;
#1982=CARTESIAN_POINT ( 'NONE',  ( -4.518350579753602325, 19.37819992234354061, 1.405661355842794391 ) ) ;
#1997=CARTESIAN_POINT ( 'NONE',  ( -1.989345975306457071, 24.75319992234354416, -1.515154207786300944 ) ) ;
#2001=CARTESIAN_POINT ( 'NONE',  ( 3.518350579753631191, 24.37180007765648071, 1.080741659609802285 ) ) ;
#2016=CARTESIAN_POINT ( 'NONE',  ( -2.518350579753628526, 30.62180007765647716, -0.7558219633769075463 ) ) ;
#2018=CARTESIAN_POINT ( 'NONE',  ( -2.864755990943265829, 30.74680007765647716, -2.011557305968488141 ) ) ;
#2024=CARTESIAN_POINT ( 'NONE',  ( 1.135272562821020070, 20.25319992234354416, -3.311245368580577164 ) ) ;
#2028=CARTESIAN_POINT ( 'NONE',  ( 0.05938372350929014415, 39.87180007765647360, 4.731580009072201776 ) ) ;
#2046=CARTESIAN_POINT ( 'NONE',  ( 3.673772985318163098, 28.00319992234354771, -2.599342558261029001 ) ) ;
#2048=CARTESIAN_POINT ( 'NONE',  ( -2.055738996568281518, 21.75319992234354416, 1.423772053676066962 ) ) ;
#2051=CARTESIAN_POINT ( 'NONE',  ( 4.518350579753602325, 38.12819992234354061, -1.405661355842793725 ) ) ;
#2057=CARTESIAN_POINT ( 'NONE',  ( -3.500000000000000444, 37.99680007765647360, 0.05647727720536892260 ) ) ;
#2061=PRODUCT_DEFINITION_SHAPE ( 'NONE', 'NONE',  #6725 ) ;
#2070=CARTESIAN_POINT ( 'NONE',  ( 3.481649420246394122, 25.87819992234354771, 1.193696214020467439 ) ) ;
#2073=CARTESIAN_POINT ( 'NONE',  ( 1.989345975306426206, 23.99680007765648071, -1.515154207786343799 ) ) ;
#2074=CARTESIAN_POINT ( 'NONE',  ( -0.05938372350918959958, 21.37819992234354416, 4.731580009072201776 ) ) ;
#2079=CARTESIAN_POINT ( 'NONE',  ( -1.336863392178478716, 37.49680007765647360, 4.297206761780677731 ) ) ;
#2092=CARTESIAN_POINT ( 'NONE',  ( -2.500000000000001332, 29.50319992234354771, -0.05647727720530596601 ) ) ;
#2094=CARTESIAN_POINT ( 'NONE',  ( -1.135272562821090014, 20.99680007765647716, -3.311245368580554072 ) ) ;
#2111=CARTESIAN_POINT ( 'NONE',  ( -0.05938372350926768989, 28.62180007765647716, -2.628655560595669183 ) ) ;
#2113=CARTESIAN_POINT ( 'NONE',  ( 3.518350579753631191, 29.37180007765647360, 1.080741659609802729 ) ) ;
#2118=CARTESIAN_POINT ( 'NONE',  ( -0.05938372350920063936, 21.37819992234353705, 3.680117784833935701 ) ) ;
#2121=CARTESIAN_POINT ( 'NONE',  ( 0.05938372350927906274, 19.87180007765648426, 3.680117784833935701 ) ) ;
#2138=CARTESIAN_POINT ( 'NONE',  ( -4.481649420246396787, 27.12819992234355126, -1.518615910253363399 ) ) ;
#2139=CARTESIAN_POINT ( 'NONE',  ( -2.864755990943222308, 39.25319992234354771, 2.011557305968548093 ) ) ;
#2140=CARTESIAN_POINT ( 'NONE',  ( -0.05938372350921170689, 18.87819992234354416, 2.628655560595669183 ) ) ;
#2143=CARTESIAN_POINT ( 'NONE',  ( -4.518350579753632523, 20.62180007765647716, -1.405661355842698468 ) ) ;
#2147=CARTESIAN_POINT ( 'NONE',  ( 2.115076519116362963, 38.87180007765645939, -3.012182706137107147 ) ) ;
#2162=CARTESIAN_POINT ( 'NONE',  ( 3.481649420246394122, 30.87819992234353350, 1.193696214020467439 ) ) ;
#2165=CARTESIAN_POINT ( 'NONE',  ( -2.055738996568313048, 20.74680007765648071, -1.423772053676023441 ) ) ;
#2167=CARTESIAN_POINT ( 'NONE',  ( -1.336863392178569088, 20.00319992234354416, -4.297206761780648421 ) ) ;
#2172=CARTESIAN_POINT ( 'NONE',  ( 1.135272562821090458, 17.24680007765647716, 3.311245368580554072 ) ) ;
#2185=CARTESIAN_POINT ( 'NONE',  ( -2.481649420246391902, 32.12819992234354771, -0.8687765177875723666 ) ) ;
#2188=CARTESIAN_POINT ( 'NONE',  ( -3.481649420246369697, 25.37180007765648071, 1.193696214020542490 ) ) ;
#2203=CARTESIAN_POINT ( 'NONE',  ( -1.989345975306426206, 27.74680007765648071, 1.515154207786343799 ) ) ;
#2205=CARTESIAN_POINT ( 'NONE',  ( 2.211161402132902243, 29.62180007765647716, 2.942372952327172442 ) ) ;
#2213=CARTESIAN_POINT ( 'NONE',  ( -3.518350579753630747, 15.62180007765647538, -1.080741659609802729 ) ) ;
#2230=CARTESIAN_POINT ( 'NONE',  ( 2.829195390882724759, 32.87819992234354771, -3.793023760679264278 ) ) ;
#2231=CARTESIAN_POINT ( 'NONE',  ( -2.115076519116425580, 34.87819992234354771, -3.012182706137063182 ) ) ;
#2232=CARTESIAN_POINT ( 'NONE',  ( 0.7188294034286553114, 18.75319992234354416, 2.395093729190349130 ) ) ;
#2234=CARTESIAN_POINT ( 'NONE',  ( 3.673772985318163098, 38.00319992234354061, -2.599342558261029001 ) ) ;
#2239=CARTESIAN_POINT ( 'NONE',  ( -3.481649420246369697, 35.37180007765648071, 1.193696214020542490 ) ) ;
#2253=CARTESIAN_POINT ( 'NONE',  ( -3.500000000000000444, 32.00319992234354771, -0.05647727720529563400 ) ) ;
#2256=CARTESIAN_POINT ( 'NONE',  ( -2.518350579753628526, 20.62180007765647716, -0.7558219633769075463 ) ) ;
#2257=CARTESIAN_POINT ( 'NONE',  ( -1.336863392178569088, 17.50319992234354771, -4.297206761780648421 ) ) ;
#2263=CARTESIAN_POINT ( 'NONE',  ( -3.673772985318219053, 38.24680007765647360, -2.599342558260952174 ) ) ;
#2273=CARTESIAN_POINT ( 'NONE',  ( 2.481649420246391902, 28.37819992234355126, 0.8687765177875720335 ) ) ;
#2275=CARTESIAN_POINT ( 'NONE',  ( -2.798362969681365886, 22.74680007765648071, 2.102939460078824929 ) ) ;
#2282=CARTESIAN_POINT ( 'NONE',  ( -2.733110507866247652, 20.12180007765647716, 3.862833514489154574 ) ) ;
#2290=CARTESIAN_POINT ( 'NONE',  ( 0.7188294034286049072, 31.24680007765648071, -2.395093729190366005 ) ) ;
#2292=CARTESIAN_POINT ( 'NONE',  ( 2.115076519116362963, 26.37180007765648071, -3.012182706137107591 ) ) ;
#2297=CARTESIAN_POINT ( 'NONE',  ( 2.798362969681366330, 23.99680007765647716, -2.102939460078824929 ) ) ;
#2311=CARTESIAN_POINT ( 'NONE',  ( -3.500000000000000444, 32.99680007765648071, 0.05647727720536892260 ) ) ;
#2318=CARTESIAN_POINT ( 'NONE',  ( 4.481649420246397675, 30.87819992234354061, 1.518615910253363177 ) ) ;
#2319=CARTESIAN_POINT ( 'NONE',  ( 0.05938372350920110426, 35.12819992234354771, -3.680117784833935701 ) ) ;
#2320=CARTESIAN_POINT ( 'NONE',  ( -1.593127413382952939, 29.12819992234354416, 2.091722143975172532 ) ) ;
#2323=CARTESIAN_POINT ( 'NONE',  ( -3.673772985318219053, 28.24680007765647360, -2.599342558260952174 ) ) ;
#2344=CARTESIAN_POINT ( 'NONE',  ( 2.115076519116426024, 33.62819992234353350, 3.012182706137062294 ) ) ;
#2348=CARTESIAN_POINT ( 'NONE',  ( -0.05938372350926768989, 28.62180007765647716, -2.628655560595669183 ) ) ;
#2349=CARTESIAN_POINT ( 'NONE',  ( -4.481649420246396787, 19.62819992234354416, -1.518615910253363399 ) ) ;
#2354=CARTESIAN_POINT ( 'NONE',  ( -1.027846397803541700, 17.49680007765647716, 3.346150245485522312 ) ) ;
#2361=CARTESIAN_POINT ( 'NONE',  ( -3.481649420246369697, 17.87180007765648071, 1.193696214020542490 ) ) ;
#2365=CARTESIAN_POINT ( 'NONE',  ( -3.481649420246394122, 14.62819992234354061, -1.193696214020467883 ) ) ;
#2366=( NAMED_UNIT ( * ) PLANE_ANGLE_UNIT ( ) SI_UNIT ( $, .RADIAN. ) );
#2368=CARTESIAN_POINT ( 'NONE',  ( -2.211161402132902243, 28.37180007765647716, -2.942372952327172886 ) ) ;
#2376=CARTESIAN_POINT ( 'NONE',  ( 2.829195390882805583, 24.62180007765647716, 3.793023760679204770 ) ) ;
#2382=CARTESIAN_POINT ( 'NONE',  ( -1.593127413382998459, 35.87180007765648071, -2.091722143975139669 ) ) ;
#2385=CARTESIAN_POINT ( 'NONE',  ( 1.135272562821090458, 32.24680007765648071, 3.311245368580554072 ) ) ;
#2392=CARTESIAN_POINT ( 'NONE',  ( 1.135272562821090458, 24.74680007765647716, 3.311245368580554072 ) ) ;
#2404=CARTESIAN_POINT ( 'NONE',  ( -3.481649420246369697, 35.37180007765648071, 1.193696214020542490 ) ) ;
#2409=CARTESIAN_POINT ( 'NONE',  ( 0.05938372350919016857, 32.62819992234354771, -4.731580009072201776 ) ) ;
#2411=CARTESIAN_POINT ( 'NONE',  ( 0.7188294034286553114, 26.25319992234354416, 2.395093729190349130 ) ) ;
#2413=CARTESIAN_POINT ( 'NONE',  ( 4.481649420246366589, 29.12180007765647005, -1.518615910253458212 ) ) ;
#2429=CARTESIAN_POINT ( 'NONE',  ( 0.05938372350927906967, 17.37180007765647360, 3.680117784833935701 ) ) ;
#2433=CARTESIAN_POINT ( 'NONE',  ( 2.211161402132839626, 35.37819992234353350, -2.942372952327218183 ) ) ;
#2434=CARTESIAN_POINT ( 'NONE',  ( 1.027846397803612311, 18.75319992234354771, 3.346150245485499219 ) ) ;
#2436=CARTESIAN_POINT ( 'NONE',  ( -0.7188294034286043521, 27.49680007765648071, 2.395093729190366005 ) ) ;
#2437=CARTESIAN_POINT ( 'NONE',  ( -1.444289557195956863, 29.00319992234354771, 4.262301884875733471 ) ) ;
#2442=CARTESIAN_POINT ( 'NONE',  ( 3.673772985318219053, 39.49680007765648071, 2.599342558260951730 ) ) ;
#2451=CARTESIAN_POINT ( 'NONE',  ( 2.115076519116362963, 18.87180007765648071, -3.012182706137107147 ) ) ;
#2457=CARTESIAN_POINT ( 'NONE',  ( 1.989345975306457071, 33.50319992234354061, 1.515154207786300500 ) ) ;
#2459=CARTESIAN_POINT ( 'NONE',  ( 0.05938372350927906274, 27.37180007765647716, 3.680117784833935701 ) ) ;
#2462=CARTESIAN_POINT ( 'NONE',  ( -2.864755990943222308, 26.75319992234354771, 2.011557305968548093 ) ) ;
#2468=CARTESIAN_POINT ( 'NONE',  ( 4.518350579753633411, 19.37180007765647716, 1.405661355842698468 ) ) ;
#2475=CARTESIAN_POINT ( 'NONE',  ( 0.7188294034286049072, 36.24680007765647360, -2.395093729190366005 ) ) ;
#2477=CARTESIAN_POINT ( 'NONE',  ( -3.518350579753630303, 35.62180007765648071, -1.080741659609802952 ) ) ;
#2480=CARTESIAN_POINT ( 'NONE',  ( -2.590630740757541073, 15.00000000000000888, -2.889634409359581380 ) ) ;
#2484=CARTESIAN_POINT ( 'NONE',  ( 3.500000000000000444, 26.74680007765648071, -0.05647727720536935281 ) ) ;
#2497=CARTESIAN_POINT ( 'NONE',  ( -1.027846397803541700, 37.49680007765647360, 3.346150245485522312 ) ) ;
#2501=CARTESIAN_POINT ( 'NONE',  ( -1.444289557195956863, 36.50319992234354061, 4.262301884875733471 ) ) ;
#2504=CARTESIAN_POINT ( 'NONE',  ( 2.518350579753611207, 30.62819992234355126, -0.7558219633769606149 ) ) ;
#2508=CARTESIAN_POINT ( 'NONE',  ( 1.444289557196047680, 24.74680007765647716, 4.262301884875704161 ) ) ;
#2523=CARTESIAN_POINT ( 'NONE',  ( -2.798362969681409851, 37.25319992234354061, -2.102939460078765421 ) ) ;
#2524=CARTESIAN_POINT ( 'NONE',  ( 1.027846397803612311, 23.75319992234354416, 3.346150245485499219 ) ) ;
#2526=CARTESIAN_POINT ( 'NONE',  ( 2.500000000000001332, 26.74680007765648071, -0.05647727720535888202 ) ) ;
#2528=CARTESIAN_POINT ( 'NONE',  ( -2.733110507866328476, 24.87819992234354771, -3.862833514489096398 ) ) ;
#2532=CARTESIAN_POINT ( 'NONE',  ( 3.481649420246369697, 24.12180007765648071, -1.193696214020541824 ) ) ;
#2540=CARTESIAN_POINT ( 'NONE',  ( -3.500000000000000444, 17.99680007765647716, 0.05647727720536892260 ) ) ;
#2546=CARTESIAN_POINT ( 'NONE',  ( 1.593127413382953383, 35.37819992234354061, -2.091722143975172532 ) ) ;
#2547=EDGE_CURVE ( 'NONE', #13037, #6995, #5736, .T. ) ;
#2549=CARTESIAN_POINT ( 'NONE',  ( 1.135272562821090458, 29.74680007765647716, 3.311245368580554072 ) ) ;
#2551=CARTESIAN_POINT ( 'NONE',  ( 3.518350579753605434, 25.62819992234353705, -1.080741659609877114 ) ) ;
#2556=CARTESIAN_POINT ( 'NONE',  ( -3.607379964056306676, 25.24680007765648071, 2.690724712371306282 ) ) ;
#2564=CARTESIAN_POINT ( 'NONE',  ( 0.05938372350926800214, 37.37180007765647360, 2.628655560595669183 ) ) ;
#2567=CARTESIAN_POINT ( 'NONE',  ( -1.135272562821090014, 35.99680007765648071, -3.311245368580554072 ) ) ;
#2570=CARTESIAN_POINT ( 'NONE',  ( -1.557381532822000203, 15.00000000000000888, -3.376484385459055826 ) ) ;
#2573=CARTESIAN_POINT ( 'NONE',  ( -2.211161402132902243, 28.37180007765647716, -2.942372952327172886 ) ) ;
#2584=CARTESIAN_POINT ( 'NONE',  ( -2.055738996568313048, 15.74680007765648071, -1.423772053676023441 ) ) ;
#2588=CARTESIAN_POINT ( 'NONE',  ( -1.444289557195956863, 31.50319992234354416, 4.262301884875733471 ) ) ;
#2591=CARTESIAN_POINT ( 'NONE',  ( -1.593127413382952939, 26.62819992234354416, 2.091722143975172532 ) ) ;
#2595=CARTESIAN_POINT ( 'NONE',  ( -1.336863392178478716, 27.49680007765647360, 4.297206761780677731 ) ) ;
#2611=CARTESIAN_POINT ( 'NONE',  ( 2.864755990943222308, 38.00319992234354061, -2.011557305968548093 ) ) ;
#2612=CARTESIAN_POINT ( 'NONE',  ( 2.115076519116425580, 18.62819992234354771, 3.012182706137062294 ) ) ;
#2615=CARTESIAN_POINT ( 'NONE',  ( 1.497042530366477164, 33.87180007765647360, -2.161531897785062384 ) ) ;
#2616=CARTESIAN_POINT ( 'NONE',  ( 3.607379964056363075, 26.00319992234354771, 2.690724712371229010 ) ) ;
#2621=CARTESIAN_POINT ( 'NONE',  ( -1.135272562821090014, 18.49680007765648071, -3.311245368580554072 ) ) ;
#2635=CARTESIAN_POINT ( 'NONE',  ( 2.500000000000001332, 35.75319992234354061, 0.05647727720530566764 ) ) ;
#2637=CARTESIAN_POINT ( 'NONE',  ( 2.211161402132902243, 34.62180007765648071, 2.942372952327172442 ) ) ;
#2638=CARTESIAN_POINT ( 'NONE',  ( -2.115076519116425580, 29.87819992234353350, -3.012182706137062738 ) ) ;
#2654=CARTESIAN_POINT ( 'NONE',  ( -1.497042530366522461, 14.87819992234354594, -2.161531897785030409 ) ) ;
#2657=CARTESIAN_POINT ( 'NONE',  ( 1.135272562821090458, 39.74680007765648071, 3.311245368580554072 ) ) ;
#2660=CARTESIAN_POINT ( 'NONE',  ( -1.139492713648220912, 15.00000000000000533, -3.396762047727180267 ) ) ;
#2664=CARTESIAN_POINT ( 'NONE',  ( -3.518350579753630747, 23.12180007765647716, -1.080741659609802729 ) ) ;
#2676=CARTESIAN_POINT ( 'NONE',  ( 3.481649420246369697, 36.62180007765648071, -1.193696214020541824 ) ) ;
#2677=ORIENTED_EDGE ( 'NONE', *, *, #5186, .T. ) ;
#2681=CARTESIAN_POINT ( 'NONE',  ( 3.673772985318219053, 16.99680007765647716, 2.599342558260951730 ) ) ;
#2684=CARTESIAN_POINT ( 'NONE',  ( 1.497042530366522461, 33.62819992234354771, 2.161531897785029965 ) ) ;
#2687=CARTESIAN_POINT ( 'NONE',  ( -1.444289557196047014, 28.49680007765648071, -4.262301884875704161 ) ) ;
#2704=CARTESIAN_POINT ( 'NONE',  ( -4.481649420246396787, 17.12819992234354416, -1.518615910253363399 ) ) ;
#2705=CARTESIAN_POINT ( 'NONE',  ( -0.05938372350920064630, 18.87819992234354771, 3.680117784833935701 ) ) ;
#2707=CARTESIAN_POINT ( 'NONE',  ( -2.481649420246374138, 30.37180007765648426, 0.8687765177876256573 ) ) ;
#2709=CARTESIAN_POINT ( 'NONE',  ( -3.607379964056363075, 24.75319992234354416, -2.690724712371229899 ) ) ;
#2714=CARTESIAN_POINT ( 'NONE',  ( 3.500000000000000444, 21.74680007765647716, -0.05647727720536935281 ) ) ;
#2719=ADVANCED_FACE ( 'NONE', ( #4664 ), #12725, .T. ) ;
#2724=CARTESIAN_POINT ( 'NONE',  ( 3.500000000000000444, 24.24680007765647716, -0.05647727720536935281 ) ) ;
#2729=CARTESIAN_POINT ( 'NONE',  ( 1.497042530366522461, 36.12819992234354771, 2.161531897785029965 ) ) ;
#2731=CARTESIAN_POINT ( 'NONE',  ( -3.500000000000000444, 30.49680007765647716, 0.05647727720536892260 ) ) ;
#2732=CARTESIAN_POINT ( 'NONE',  ( -2.864755990943222308, 29.25319992234354416, 2.011557305968548093 ) ) ;
#2743=CARTESIAN_POINT ( 'NONE',  ( -0.05938372350921170689, 16.37819992234354416, 2.628655560595669183 ) ) ;
#2753=CARTESIAN_POINT ( 'NONE',  ( 0.05938372350927906274, 29.87180007765648071, 3.680117784833935701 ) ) ;
#2766=CARTESIAN_POINT ( 'NONE',  ( 0.8262555684461332373, 17.24680007765648071, 2.360188852285403982 ) ) ;
#2771=CARTESIAN_POINT ( 'NONE',  ( -2.829195390882724315, 39.12819992234354771, 3.793023760679264722 ) ) ;
#2774=CARTESIAN_POINT ( 'NONE',  ( 0.05938372350921204690, 32.62819992234354771, -2.628655560595669183 ) ) ;
#2777=CARTESIAN_POINT ( 'NONE',  ( 2.733110507866247652, 36.37180007765647360, -3.862833514489153686 ) ) ;
#2791=CARTESIAN_POINT ( 'NONE',  ( 3.673772985318163098, 18.00319992234354416, -2.599342558261029001 ) ) ;
#2792=CARTESIAN_POINT ( 'NONE',  ( -2.115076519116425580, 17.37819992234354416, -3.012182706137063182 ) ) ;
#2794=CARTESIAN_POINT ( 'NONE',  ( 0.05938372350926800214, 37.37180007765647360, 2.628655560595669183 ) ) ;
#2795=CARTESIAN_POINT ( 'NONE',  ( -4.481649420246396787, 27.12819992234355126, -1.518615910253363399 ) ) ;
#2800=CARTESIAN_POINT ( 'NONE',  ( 2.115076519116362963, 23.87180007765647005, -3.012182706137107147 ) ) ;
#2808=CARTESIAN_POINT ( 'NONE',  ( 3.481649420246369697, 26.62180007765648071, -1.193696214020541824 ) ) ;
#2814=CARTESIAN_POINT ( 'NONE',  ( 3.500000000000000444, 20.75319992234354416, 0.05647727720529520379 ) ) ;
#2816=CARTESIAN_POINT ( 'NONE',  ( -2.115076519116362519, 37.62180007765648071, 3.012182706137107147 ) ) ;
#2818=CARTESIAN_POINT ( 'NONE',  ( 3.481649420246394122, 28.37819992234354416, 1.193696214020467439 ) ) ;
#2829=CARTESIAN_POINT ( 'NONE',  ( -0.8262555684460826111, 19.00319992234354771, 2.360188852285421302 ) ) ;
#2837=CARTESIAN_POINT ( 'NONE',  ( -2.798362969681365886, 30.24680007765648071, 2.102939460078824929 ) ) ;
#2847=CARTESIAN_POINT ( 'NONE',  ( -2.864755990943265829, 38.24680007765647360, -2.011557305968488141 ) ) ;
#2851=CARTESIAN_POINT ( 'NONE',  ( -0.7188294034286550893, 35.00319992234354771, -2.395093729190349130 ) ) ;
#2854=CARTESIAN_POINT ( 'NONE',  ( 4.481649420246366589, 36.62180007765647360, -1.518615910253458212 ) ) ;
#2874=CARTESIAN_POINT ( 'NONE',  ( -4.481649420246396787, 22.12819992234354416, -1.518615910253363399 ) ) ;
#2875=CARTESIAN_POINT ( 'NONE',  ( -2.798362969681409851, 24.75319992234354416, -2.102939460078765421 ) ) ;
#2877=CARTESIAN_POINT ( 'NONE',  ( 2.500000000000001332, 15.75319992234354594, 0.05647727720530566764 ) ) ;
#2878=CARTESIAN_POINT ( 'NONE',  ( 1.336863392178569754, 33.75319992234354771, 4.297206761780648421 ) ) ;
#2884=CARTESIAN_POINT ( 'NONE',  ( -3.481649420246369697, 20.37180007765647716, 1.193696214020542490 ) ) ;
#2887=CARTESIAN_POINT ( 'NONE',  ( -1.336863392178478716, 19.99680007765647716, 4.297206761780677731 ) ) ;
#2892=CARTESIAN_POINT ( 'NONE',  ( -2.211161402132902243, 23.37180007765647716, -2.942372952327172886 ) ) ;
#2898=CARTESIAN_POINT ( 'NONE',  ( -0.05938372350920063936, 16.37819992234354416, 3.680117784833935701 ) ) ;
#2901=CARTESIAN_POINT ( 'NONE',  ( 1.027846397803542144, 38.74680007765647360, -3.346150245485522312 ) ) ;
#2902=CARTESIAN_POINT ( 'NONE',  ( -2.798362969681409851, 34.75319992234354771, -2.102939460078765421 ) ) ;
#2913=CARTESIAN_POINT ( 'NONE',  ( -2.754179286501430735, 15.00000000000001954, -1.305413474713025490 ) ) ;
#2916=CARTESIAN_POINT ( 'NONE',  ( -1.497042530366522461, 22.37819992234354416, -2.161531897785030409 ) ) ;
#2918=CARTESIAN_POINT ( 'NONE',  ( -1.135272562821090014, 18.49680007765648071, -3.311245368580554072 ) ) ;
#2924=CARTESIAN_POINT ( 'NONE',  ( 2.211161402132902243, 34.62180007765648071, 2.942372952327172442 ) ) ;
#2928=CARTESIAN_POINT ( 'NONE',  ( 0.000000000000000000, 15.00000000000000355, 0.000000000000000000 ) ) ;
#2936=CARTESIAN_POINT ( 'NONE',  ( 1.989345975306426206, 21.49680007765648071, -1.515154207786343799 ) ) ;
#2938=CARTESIAN_POINT ( 'NONE',  ( -3.500000000000000444, 20.49680007765647716, 0.05647727720536892260 ) ) ;
#2943=CARTESIAN_POINT ( 'NONE',  ( -0.8262555684460826111, 39.00319992234355482, 2.360188852285421302 ) ) ;
#2947=CARTESIAN_POINT ( 'NONE',  ( -3.673772985318219053, 30.74680007765647716, -2.599342558260952174 ) ) ;
#2962=CARTESIAN_POINT ( 'NONE',  ( 2.829195390882724759, 20.37819992234354416, -3.793023760679264278 ) ) ;
#2963=CARTESIAN_POINT ( 'NONE',  ( 2.864755990943222308, 25.50319992234354771, -2.011557305968548093 ) ) ;
#2964=CARTESIAN_POINT ( 'NONE',  ( -2.518350579753628526, 35.62180007765647360, -0.7558219633769075463 ) ) ;
#2968=CARTESIAN_POINT ( 'NONE',  ( -2.733110507866328476, 29.87819992234354416, -3.862833514489096398 ) ) ;
#2974=CARTESIAN_POINT ( 'NONE',  ( 3.518350579753631191, 29.37180007765647005, 1.080741659609802285 ) ) ;
#2977=CARTESIAN_POINT ( 'NONE',  ( 4.481649420246366589, 31.62180007765647716, -1.518615910253458212 ) ) ;
#2981=CARTESIAN_POINT ( 'NONE',  ( 1.027846397803542144, 21.24680007765647716, -3.346150245485522312 ) ) ;
#2985=( LENGTH_UNIT ( ) NAMED_UNIT ( * ) SI_UNIT ( .MILLI., .METRE. ) );
#2988=CARTESIAN_POINT ( 'NONE',  ( -1.135272562821019626, 19.00319992234354771, 3.311245368580577164 ) ) ;
#2990=CARTESIAN_POINT ( 'NONE',  ( -3.500000000000000444, 37.99680007765647360, 0.05647727720536892260 ) ) ;
#2992=CARTESIAN_POINT ( 'NONE',  ( 2.798362969681409851, 38.50319992234354061, 2.102939460078764977 ) ) ;
#3005=CARTESIAN_POINT ( 'NONE',  ( -2.055738996568281518, 19.25319992234354416, 1.423772053676066962 ) ) ;
#3007=CARTESIAN_POINT ( 'NONE',  ( 1.135272562821090458, 17.24680007765647716, 3.311245368580554072 ) ) ;
#3015=CARTESIAN_POINT ( 'NONE',  ( 1.027846397803542144, 36.24680007765648071, -3.346150245485522312 ) ) ;
#3024=DIRECTION ( 'NONE',  ( 0.000000000000000000, -0.9936001553129347741, -0.1129545544106647093 ) ) ;
#3026=CARTESIAN_POINT ( 'NONE',  ( -0.7188294034286043521, 19.99680007765648071, 2.395093729190366005 ) ) ;
#3028=CARTESIAN_POINT ( 'NONE',  ( -3.500000000000000444, 25.49680007765647716, 0.05647727720536892260 ) ) ;
#3035=CARTESIAN_POINT ( 'NONE',  ( -1.497042530366522461, 37.37819992234354771, -2.161531897785030409 ) ) ;
#3040=CARTESIAN_POINT ( 'NONE',  ( 0.05938372350929014415, 34.87180007765647360, 4.731580009072201776 ) ) ;
#3056=CARTESIAN_POINT ( 'NONE',  ( -3.673772985318163098, 19.25319992234354416, 2.599342558261029001 ) ) ;
#3057=CARTESIAN_POINT ( 'NONE',  ( 0.05938372350920110426, 27.62819992234354061, -3.680117784833935701 ) ) ;
#3058=CARTESIAN_POINT ( 'NONE',  ( 0.05938372350921204690, 15.12819992234354771, -2.628655560595669183 ) ) ;
#3060=CARTESIAN_POINT ( 'NONE',  ( -1.336863392178569088, 35.00319992234354771, -4.297206761780648421 ) ) ;
#3065=CARTESIAN_POINT ( 'NONE',  ( -3.500000000000000444, 32.99680007765648071, 0.05647727720536892260 ) ) ;
#3068=CARTESIAN_POINT ( 'NONE',  ( 2.829195390882805583, 32.12180007765646650, 3.793023760679204770 ) ) ;
#3072=CARTESIAN_POINT ( 'NONE',  ( 3.518350579753631191, 21.87180007765647360, 1.080741659609802285 ) ) ;
#3079=CARTESIAN_POINT ( 'NONE',  ( -3.518350579753605434, 21.87819992234354771, 1.080741659609877781 ) ) ;
#3082=CARTESIAN_POINT ( 'NONE',  ( 1.027846397803542144, 36.24680007765648071, -3.346150245485522312 ) ) ;
#3083=CARTESIAN_POINT ( 'NONE',  ( -2.211161402132839182, 34.12819992234355482, 2.942372952327218627 ) ) ;
#3099=CARTESIAN_POINT ( 'NONE',  ( -2.055738996568281518, 21.75319992234354416, 1.423772053676066962 ) ) ;
#3103=CARTESIAN_POINT ( 'NONE',  ( 3.607379964056306676, 16.49680007765647716, -2.690724712371305838 ) ) ;
#3109=CARTESIAN_POINT ( 'NONE',  ( -2.115076519116362519, 35.12180007765645939, 3.012182706137107147 ) ) ;
#3118=FACE_OUTER_BOUND ( 'NONE', #16048, .T. ) ;
#3120=CARTESIAN_POINT ( 'NONE',  ( 0.05938372350926800214, 24.87180007765647716, 2.628655560595669183 ) ) ;
#3122=CARTESIAN_POINT ( 'NONE',  ( 2.211161402132902243, 19.62180007765647716, 2.942372952327172442 ) ) ;
#3126=CARTESIAN_POINT ( 'NONE',  ( 3.481649420246394122, 18.37819992234354771, 1.193696214020467439 ) ) ;
#3129=CARTESIAN_POINT ( 'NONE',  ( 4.518350579753633411, 34.37180007765647360, 1.405661355842698468 ) ) ;
#3147=CARTESIAN_POINT ( 'NONE',  ( -2.829195390882724315, 29.12819992234354416, 3.793023760679264722 ) ) ;
#3149=CARTESIAN_POINT ( 'NONE',  ( -2.115076519116425580, 29.87819992234354061, -3.012182706137063182 ) ) ;
#3151=CARTESIAN_POINT ( 'NONE',  ( -2.481649420246374138, 35.37180007765647360, 0.8687765177876256573 ) ) ;
#3153=CARTESIAN_POINT ( 'NONE',  ( -2.829195390882724315, 31.62819992234354416, 3.793023760679264722 ) ) ;
#3157=CARTESIAN_POINT ( 'NONE',  ( -1.135272562821090014, 30.99680007765647716, -3.311245368580554072 ) ) ;
#3161=CARTESIAN_POINT ( 'NONE',  ( -1.336863392178478716, 29.99680007765647716, 4.297206761780677731 ) ) ;
#3166=CARTESIAN_POINT ( 'NONE',  ( 3.518350579753631191, 31.87180007765647716, 1.080741659609802285 ) ) ;
#3171=CARTESIAN_POINT ( 'NONE',  ( -1.135272562821019626, 21.50319992234354416, 3.311245368580577164 ) ) ;
#3174=CARTESIAN_POINT ( 'NONE',  ( -2.481649420246374138, 17.87180007765647716, 0.8687765177876256573 ) ) ;
#3175=CARTESIAN_POINT ( 'NONE',  ( -3.518350579753605434, 36.87819992234354771, 1.080741659609877781 ) ) ;
#3192=CARTESIAN_POINT ( 'NONE',  ( -2.500000000000001332, 22.00319992234354771, -0.05647727720530596601 ) ) ;
#3194=CARTESIAN_POINT ( 'NONE',  ( 3.500000000000000444, 16.74680007765647716, -0.05647727720536935281 ) ) ;
#3199=CARTESIAN_POINT ( 'NONE',  ( -2.798362969681365886, 40.24680007765648071, 2.102939460078824929 ) ) ;
#3214=CARTESIAN_POINT ( 'NONE',  ( -2.518350579753628526, 23.12180007765647005, -0.7558219633769075463 ) ) ;
#3218=CARTESIAN_POINT ( 'NONE',  ( -2.115076519116362519, 22.62180007765647716, 3.012182706137108035 ) ) ;
#3222=CARTESIAN_POINT ( 'NONE',  ( 0.05938372350920109732, 20.12819992234353705, -3.680117784833935701 ) ) ;
#3225=CARTESIAN_POINT ( 'NONE',  ( -2.733110507866247652, 40.12180007765647360, 3.862833514489154574 ) ) ;
#3244=CARTESIAN_POINT ( 'NONE',  ( -1.336863392178569088, 25.00319992234354771, -4.297206761780648421 ) ) ;
#3245=CARTESIAN_POINT ( 'NONE',  ( -3.481649420246394566, 24.62819992234354061, -1.193696214020467883 ) ) ;
#3246=CARTESIAN_POINT ( 'NONE',  ( 2.055738996568281518, 20.50319992234355126, -1.423772053676066518 ) ) ;
#3248=CARTESIAN_POINT ( 'NONE',  ( -3.607379964056306676, 17.74680007765647716, 2.690724712371306282 ) ) ;
#3252=CARTESIAN_POINT ( 'NONE',  ( -2.798362969681365886, 27.74680007765648071, 2.102939460078824929 ) ) ;
#3257=CARTESIAN_POINT ( 'NONE',  ( 4.499999999999999112, 29.24680007765647716, -0.05647727720537982360 ) ) ;
#3260=CARTESIAN_POINT ( 'NONE',  ( -0.05938372350927861171, 28.62180007765648071, -3.680117784833935701 ) ) ;
#3266=CARTESIAN_POINT ( 'NONE',  ( -0.05938372350920063936, 28.87819992234353705, 3.680117784833935701 ) ) ;
#3270=CARTESIAN_POINT ( 'NONE',  ( 1.497042530366477164, 23.87180007765647716, -2.161531897785062384 ) ) ;
#3273=CARTESIAN_POINT ( 'NONE',  ( 2.864755990943222308, 33.00319992234354771, -2.011557305968548093 ) ) ;
#3287=CARTESIAN_POINT ( 'NONE',  ( -1.497042530366522461, 24.87819992234354771, -2.161531897785030409 ) ) ;
#3294=CARTESIAN_POINT ( 'NONE',  ( 0.05938372350927906274, 37.37180007765645939, 3.680117784833935701 ) ) ;
#3304=CARTESIAN_POINT ( 'NONE',  ( 2.500000000000001332, 19.24680007765648071, -0.05647727720535888202 ) ) ;
#3306=CARTESIAN_POINT ( 'NONE',  ( 1.027846397803542144, 23.74680007765647716, -3.346150245485522312 ) ) ;
#3312=CARTESIAN_POINT ( 'NONE',  ( -2.115076519116425580, 14.87819992234354594, -3.012182706137062738 ) ) ;
#3315=CARTESIAN_POINT ( 'NONE',  ( 3.518350579753631191, 19.37180007765648071, 1.080741659609802285 ) ) ;
#3337=CARTESIAN_POINT ( 'NONE',  ( 3.607379964056363075, 28.50319992234354416, 2.690724712371229010 ) ) ;
#3338=CARTESIAN_POINT ( 'NONE',  ( 3.481649420246395010, 38.37819992234354061, 1.193696214020467439 ) ) ;
#3339=CARTESIAN_POINT ( 'NONE',  ( -0.05938372350921170689, 16.37819992234354416, 2.628655560595669183 ) ) ;
#3341=CARTESIAN_POINT ( 'NONE',  ( 3.607379964056306676, 16.49680007765647716, -2.690724712371305838 ) ) ;
#3347=CARTESIAN_POINT ( 'NONE',  ( -3.518350579753630747, 28.12180007765647360, -1.080741659609802729 ) ) ;
#3350=CARTESIAN_POINT ( 'NONE',  ( -1.444289557196047014, 28.49680007765648071, -4.262301884875704161 ) ) ;
#3353=CARTESIAN_POINT ( 'NONE',  ( -3.518350579753630747, 30.62180007765647716, -1.080741659609802729 ) ) ;
#3358=( NAMED_UNIT ( * ) SI_UNIT ( $, .STERADIAN. ) SOLID_ANGLE_UNIT ( ) );
#3361=CARTESIAN_POINT ( 'NONE',  ( 3.500000000000000444, 28.25319992234354416, 0.05647727720529520379 ) ) ;
#3364=CARTESIAN_POINT ( 'NONE',  ( -0.8262555684461330152, 18.49680007765647716, -2.360188852285403982 ) ) ;
#3366=CARTESIAN_POINT ( 'NONE',  ( 1.444289557195957086, 20.25319992234354416, -4.262301884875733471 ) ) ;
#3382=CARTESIAN_POINT ( 'NONE',  ( -2.500000000000001332, 27.00319992234355126, -0.05647727720530596601 ) ) ;
#3385=CARTESIAN_POINT ( 'NONE',  ( 2.864755990943265829, 21.99680007765647716, 2.011557305968487697 ) ) ;
#3399=CARTESIAN_POINT ( 'NONE',  ( -1.497042530366477164, 30.12180007765648426, 2.161531897785062384 ) ) ;
#3402=CARTESIAN_POINT ( 'NONE',  ( 3.500000000000000444, 31.74680007765647716, -0.05647727720536935281 ) ) ;
#3407=CARTESIAN_POINT ( 'NONE',  ( 3.500000000000000444, 15.75319992234354416, 0.05647727720529520379 ) ) ;
#3410=CARTESIAN_POINT ( 'NONE',  ( -4.499999999999999112, 37.99680007765646650, 0.05647727720537927543 ) ) ;
#3429=CARTESIAN_POINT ( 'NONE',  ( -1.336863392178569088, 27.50319992234354771, -4.297206761780648421 ) ) ;
#3430=CARTESIAN_POINT ( 'NONE',  ( -1.027846397803611866, 32.50319992234354771, -3.346150245485499219 ) ) ;
#3431=CARTESIAN_POINT ( 'NONE',  ( -2.481649420246391902, 17.12819992234354416, -0.8687765177875723666 ) ) ;
#3433=CARTESIAN_POINT ( 'NONE',  ( -0.05938372350918959958, 38.87819992234354771, 4.731580009072201776 ) ) ;
#3450=CARTESIAN_POINT ( 'NONE',  ( 2.115076519116426024, 26.12819992234354771, 3.012182706137062294 ) ) ;
#3451=CARTESIAN_POINT ( 'NONE',  ( -1.055605843668875110, 15.00000000000000888, -3.337496964141338562 ) ) ;
#3453=CARTESIAN_POINT ( 'NONE',  ( 0.05938372350926800214, 22.37180007765647716, 2.628655560595669183 ) ) ;
#3455=CARTESIAN_POINT ( 'NONE',  ( 2.733110507866328920, 18.62819992234354771, 3.862833514489095510 ) ) ;
#3471=CARTESIAN_POINT ( 'NONE',  ( -2.518350579753611207, 31.87819992234354416, 0.7558219633769609480 ) ) ;
#3474=CARTESIAN_POINT ( 'NONE',  ( 1.027846397803542144, 21.24680007765647716, -3.346150245485522312 ) ) ;
#3485=CARTESIAN_POINT ( 'NONE',  ( -3.500000000000000444, 40.00000000000000711, 3.664603343001004987E-14 ) ) ;
#3486=CARTESIAN_POINT ( 'NONE',  ( 0.05938372350926800214, 27.37180007765647716, 2.628655560595669183 ) ) ;
#3488=CARTESIAN_POINT ( 'NONE',  ( 2.115076519116362963, 28.87180007765647716, -3.012182706137107591 ) ) ;
#3494=CARTESIAN_POINT ( 'NONE',  ( -3.500000000000000444, 22.00319992234354416, -0.05647727720529563400 ) ) ;
#3498=CARTESIAN_POINT ( 'NONE',  ( -4.499999999999999112, 40.49680007765648071, 0.05647727720537927543 ) ) ;
#3517=CARTESIAN_POINT ( 'NONE',  ( -3.673772985318163098, 24.25319992234354061, 2.599342558261029001 ) ) ;
#3518=CARTESIAN_POINT ( 'NONE',  ( 1.135272562821020070, 35.25319992234354771, -3.311245368580577164 ) ) ;
#3519=CARTESIAN_POINT ( 'NONE',  ( 0.8262555684460829442, 22.75319992234354771, -2.360188852285421302 ) ) ;
#3522=CARTESIAN_POINT ( 'NONE',  ( -4.499999999999999112, 15.49680007765647538, 0.05647727720537927543 ) ) ;
#3527=CARTESIAN_POINT ( 'NONE',  ( -1.135272562821090014, 38.49680007765647360, -3.311245368580554072 ) ) ;
#3542=CARTESIAN_POINT ( 'NONE',  ( 1.027846397803612311, 31.25319992234354416, 3.346150245485499219 ) ) ;
#3545=CARTESIAN_POINT ( 'NONE',  ( 2.518350579753628971, 19.37180007765648071, 0.7558219633769073242 ) ) ;
#3546=CARTESIAN_POINT ( 'NONE',  ( 1.336863392178569754, 16.25319992234354416, 4.297206761780648421 ) ) ;
#3552=CARTESIAN_POINT ( 'NONE',  ( 3.500000000000000444, 16.74680007765647716, -0.05647727720536935281 ) ) ;
#3564=CARTESIAN_POINT ( 'NONE',  ( -2.500000000000001332, 24.50319992234354771, -0.05647727720530596601 ) ) ;
#3567=CARTESIAN_POINT ( 'NONE',  ( -2.864755990943265829, 23.24680007765647716, -2.011557305968488141 ) ) ;
#3577=CARTESIAN_POINT ( 'NONE',  ( -2.481649420246374138, 27.87180007765648426, 0.8687765177876256573 ) ) ;
#3579=CARTESIAN_POINT ( 'NONE',  ( 1.027846397803542144, 26.24680007765648071, -3.346150245485522312 ) ) ;
#3586=CARTESIAN_POINT ( 'NONE',  ( 2.115076519116362963, 16.37180007765647716, -3.012182706137107147 ) ) ;
#3602=CARTESIAN_POINT ( 'NONE',  ( 4.481649420246397675, 33.37819992234354771, 1.518615910253363177 ) ) ;
#3604=CARTESIAN_POINT ( 'NONE',  ( 2.115076519116425580, 33.62819992234354061, 3.012182706137062294 ) ) ;
#3606=CARTESIAN_POINT ( 'NONE',  ( -2.055738996568281518, 19.25319992234354416, 1.423772053676066962 ) ) ;
#3609=CARTESIAN_POINT ( 'NONE',  ( 4.518350579753633411, 16.87180007765647716, 1.405661355842698468 ) ) ;
#3619=PRODUCT_DEFINITION_FORMATION_WITH_SPECIFIED_SOURCE ( 'ANY', '', #4859, .NOT_KNOWN. ) ;
#3620=CARTESIAN_POINT ( 'NONE',  ( -3.500000000000000444, 39.50319992234354061, -0.05647727720529600870 ) ) ;
#3628=CARTESIAN_POINT ( 'NONE',  ( -1.027846397803611866, 27.50319992234354771, -3.346150245485499219 ) ) ;
#3632=CARTESIAN_POINT ( 'NONE',  ( -0.8262555684461330152, 25.99680007765648071, -2.360188852285403982 ) ) ;
#3634=CARTESIAN_POINT ( 'NONE',  ( -3.500000000000000444, 39.50319992234354771, -0.05647727720529563400 ) ) ;
#3640=CARTESIAN_POINT ( 'NONE',  ( -1.135272562821090014, 15.99680007765647716, -3.311245368580554072 ) ) ;
#3650=CARTESIAN_POINT ( 'NONE',  ( 2.500000000000001332, 25.75319992234354771, 0.05647727720530566764 ) ) ;
#3652=CARTESIAN_POINT ( 'NONE',  ( -3.500000000000000444, 25.49680007765647716, 0.05647727720536892260 ) ) ;
#3662=CARTESIAN_POINT ( 'NONE',  ( 2.829195390882805583, 19.62180007765647716, 3.793023760679204770 ) ) ;
#3671=CARTESIAN_POINT ( 'NONE',  ( 2.055738996568313048, 29.49680007765648426, 1.423772053676023441 ) ) ;
#3673=CARTESIAN_POINT ( 'NONE',  ( -2.211161402132901799, 33.37180007765648071, -2.942372952327172886 ) ) ;
#3675=SHAPE_DEFINITION_REPRESENTATION ( #2061, #5199 ) ;
#3679=CARTESIAN_POINT ( 'NONE',  ( -1.135272562821090014, 23.49680007765647716, -3.311245368580554072 ) ) ;
#3690=CARTESIAN_POINT ( 'NONE',  ( 2.864755990943265829, 34.49680007765648071, 2.011557305968487697 ) ) ;
#3694=CARTESIAN_POINT ( 'NONE',  ( -3.673772985318163098, 36.75319992234353350, 2.599342558261029001 ) ) ;
#3695=CARTESIAN_POINT ( 'NONE',  ( 2.864755990943222308, 33.00319992234354771, -2.011557305968548093 ) ) ;
#3696=CARTESIAN_POINT ( 'NONE',  ( -1.989345975306457071, 27.25319992234354771, -1.515154207786300944 ) ) ;
#3698=CARTESIAN_POINT ( 'NONE',  ( 3.607379964056306676, 23.99680007765647716, -2.690724712371305838 ) ) ;
#3702=CARTESIAN_POINT ( 'NONE',  ( -2.211161402132902243, 35.87180007765648782, -2.942372952327172886 ) ) ;
#3713=CARTESIAN_POINT ( 'NONE',  ( -1.135272562821019626, 39.00319992234354061, 3.311245368580577164 ) ) ;
#3716=CARTESIAN_POINT ( 'NONE',  ( -2.500000000000001332, 30.49680007765648071, 0.05647727720535858364 ) ) ;
#3717=CARTESIAN_POINT ( 'NONE',  ( -1.336863392178569088, 15.00319992234354594, -4.297206761780648421 ) ) ;
#3722=CARTESIAN_POINT ( 'NONE',  ( -2.829195390882805139, 35.87180007765647360, -3.793023760679206102 ) ) ;
#3730=CARTESIAN_POINT ( 'NONE',  ( 2.211161402132902243, 19.62180007765647360, 2.942372952327172442 ) ) ;
#3734=CARTESIAN_POINT ( 'NONE',  ( -2.481649420246391902, 37.12819992234354771, -0.8687765177875723666 ) ) ;
#3736=CARTESIAN_POINT ( 'NONE',  ( 2.211161402132902243, 22.12180007765648071, 2.942372952327172442 ) ) ;
#3743=CARTESIAN_POINT ( 'NONE',  ( 4.499999999999999112, 26.74680007765647360, -0.05647727720537982360 ) ) ;
#3752=CARTESIAN_POINT ( 'NONE',  ( 1.989345975306426206, 33.99680007765647360, -1.515154207786343799 ) ) ;
#3754=CARTESIAN_POINT ( 'NONE',  ( -0.05938372350927861865, 26.12180007765647716, -3.680117784833935701 ) ) ;
#3762=CARTESIAN_POINT ( 'NONE',  ( -1.027846397803541700, 27.49680007765648071, 3.346150245485522312 ) ) ;
#3773=CARTESIAN_POINT ( 'NONE',  ( 1.135272562821090458, 34.74680007765648071, 3.311245368580554072 ) ) ;
#3779=CARTESIAN_POINT ( 'NONE',  ( 2.829195390882724759, 35.37819992234354061, -3.793023760679264278 ) ) ;
#3782=CARTESIAN_POINT ( 'NONE',  ( -0.8262555684460826111, 26.50319992234354771, 2.360188852285421302 ) ) ;
#3784=CARTESIAN_POINT ( 'NONE',  ( -2.733110507866247652, 25.12180007765648071, 3.862833514489154574 ) ) ;
#3796=CARTESIAN_POINT ( 'NONE',  ( -2.211161402132901799, 15.87180007765647716, -2.942372952327172886 ) ) ;
#3801=CARTESIAN_POINT ( 'NONE',  ( -0.05938372350920063936, 31.37819992234354416, 3.680117784833935701 ) ) ;
#3802=CARTESIAN_POINT ( 'NONE',  ( 2.115076519116425580, 21.12819992234354061, 3.012182706137062294 ) ) ;
#3804=CARTESIAN_POINT ( 'NONE',  ( 1.593127413382998903, 29.62180007765647716, 2.091722143975139669 ) ) ;
#3805=CARTESIAN_POINT ( 'NONE',  ( -0.05938372350918959958, 23.87819992234354416, 4.731580009072201776 ) ) ;
#3810=CARTESIAN_POINT ( 'NONE',  ( 1.336863392178479160, 36.24680007765647360, -4.297206761780677731 ) ) ;
#3820=CARTESIAN_POINT ( 'NONE',  ( 2.864755990943265829, 16.99680007765647716, 2.011557305968487697 ) ) ;
#3826=CARTESIAN_POINT ( 'NONE',  ( -1.989345975306457071, 34.75319992234354771, -1.515154207786300944 ) ) ;
#3828=CARTESIAN_POINT ( 'NONE',  ( 1.135272562821090458, 32.24680007765648071, 3.311245368580554072 ) ) ;
#3831=CARTESIAN_POINT ( 'NONE',  ( 2.864755990943222308, 23.00319992234354416, -2.011557305968548093 ) ) ;
#3839=CARTESIAN_POINT ( 'NONE',  ( -4.481649420246366589, 20.37180007765648071, 1.518615910253458878 ) ) ;
#3848=CARTESIAN_POINT ( 'NONE',  ( -0.7188294034286043521, 34.99680007765648071, 2.395093729190366005 ) ) ;
#3850=CARTESIAN_POINT ( 'NONE',  ( 3.481649420246370141, 34.12180007765648071, -1.193696214020541602 ) ) ;
#3856=CARTESIAN_POINT ( 'NONE',  ( -3.481649420246369697, 25.37180007765648071, 1.193696214020542490 ) ) ;
#3857=ORIENTED_EDGE ( 'NONE', *, *, #5186, .F. ) ;
#3869=CARTESIAN_POINT ( 'NONE',  ( -0.8262555684461330152, 18.49680007765647716, -2.360188852285403982 ) ) ;
#3874=CARTESIAN_POINT ( 'NONE',  ( -3.673772985318163098, 34.25319992234354061, 2.599342558261029001 ) ) ;
#3876=CARTESIAN_POINT ( 'NONE',  ( 1.989345975306457071, 28.50319992234355126, 1.515154207786300500 ) ) ;
#3879=CARTESIAN_POINT ( 'NONE',  ( 4.518350579753633411, 24.37180007765647005, 1.405661355842698468 ) ) ;
#3894=CARTESIAN_POINT ( 'NONE',  ( -3.500000000000000444, 15.49680007765647893, 0.05647727720536901974 ) ) ;
#3898=CARTESIAN_POINT ( 'NONE',  ( -3.481649420246394122, 37.12819992234354771, -1.193696214020467883 ) ) ;
#3899=CARTESIAN_POINT ( 'NONE',  ( 0.05938372350920110426, 20.12819992234354061, -3.680117784833935701 ) ) ;
#3901=CARTESIAN_POINT ( 'NONE',  ( -2.500000000000001332, 27.99680007765648426, 0.05647727720535858364 ) ) ;
#3902=CARTESIAN_POINT ( 'NONE',  ( 4.499999999999999112, 28.25319992234354416, 0.05647727720528474687 ) ) ;
#3906=CARTESIAN_POINT ( 'NONE',  ( 2.733110507866247652, 38.87180007765646650, -3.862833514489153686 ) ) ;
#3914=CARTESIAN_POINT ( 'NONE',  ( 3.500000000000000444, 16.74680007765647716, -0.05647727720536935281 ) ) ;
#3920=CARTESIAN_POINT ( 'NONE',  ( -0.05938372350921170689, 33.87819992234354061, 2.628655560595669183 ) ) ;
#3922=CARTESIAN_POINT ( 'NONE',  ( 2.115076519116362963, 33.87180007765648071, -3.012182706137107147 ) ) ;
#3924=CARTESIAN_POINT ( 'NONE',  ( -1.135272562821019626, 24.00319992234354416, 3.311245368580577164 ) ) ;
#3931=CARTESIAN_POINT ( 'NONE',  ( 1.336863392178479160, 23.74680007765647716, -4.297206761780677731 ) ) ;
#3938=CARTESIAN_POINT ( 'NONE',  ( 2.481649420246374138, 39.12180007765647360, -0.8687765177876252132 ) ) ;
#3940=CARTESIAN_POINT ( 'NONE',  ( 1.135272562821090458, 37.24680007765648071, 3.311245368580554072 ) ) ;
#3945=CARTESIAN_POINT ( 'NONE',  ( -2.054657775866485014, 15.00000000000001243, -3.211012929026491047 ) ) ;
#3948=CARTESIAN_POINT ( 'NONE',  ( -3.518350579753630747, 20.62180007765646650, -1.080741659609802729 ) ) ;
#3959=CARTESIAN_POINT ( 'NONE',  ( 0.7188294034286049072, 16.24680007765648071, -2.395093729190366005 ) ) ;
#3963=CARTESIAN_POINT ( 'NONE',  ( -4.481649420246396787, 34.62819992234354771, -1.518615910253363399 ) ) ;
#3965=CARTESIAN_POINT ( 'NONE',  ( 2.500000000000001332, 30.75319992234354416, 0.05647727720530566764 ) ) ;
#3969=CARTESIAN_POINT ( 'NONE',  ( -2.733110507866247652, 22.62180007765647360, 3.862833514489154574 ) ) ;
#3985=CARTESIAN_POINT ( 'NONE',  ( -2.115076519116425580, 34.87819992234354771, -3.012182706137062738 ) ) ;
#3986=CARTESIAN_POINT ( 'NONE',  ( -3.518350579753606322, 16.87819992234354061, 1.080741659609877781 ) ) ;
#3988=CARTESIAN_POINT ( 'NONE',  ( 2.500000000000001332, 31.74680007765648782, -0.05647727720535888202 ) ) ;
#3991=CARTESIAN_POINT ( 'NONE',  ( -2.829195390882724315, 24.12819992234354771, 3.793023760679264722 ) ) ;
#3997=CARTESIAN_POINT ( 'NONE',  ( -1.135272562821090014, 25.99680007765648071, -3.311245368580554072 ) ) ;
#4007=CARTESIAN_POINT ( 'NONE',  ( 1.027846397803542144, 16.24680007765647716, -3.346150245485522312 ) ) ;
#4013=CARTESIAN_POINT ( 'NONE',  ( -2.055738996568281518, 36.75319992234354771, 1.423772053676066962 ) ) ;
#4015=CARTESIAN_POINT ( 'NONE',  ( 3.500000000000000444, 34.24680007765648071, -0.05647727720536935281 ) ) ;
#4016=CARTESIAN_POINT ( 'NONE',  ( -2.211161402132839182, 29.12819992234354771, 2.942372952327218627 ) ) ;
#4027=CARTESIAN_POINT ( 'NONE',  ( 1.497042530366477164, 36.37180007765648071, -2.161531897785062384 ) ) ;
#4029=CARTESIAN_POINT ( 'NONE',  ( -2.798362969681365886, 35.24680007765648071, 2.102939460078824929 ) ) ;
#4034=CARTESIAN_POINT ( 'NONE',  ( -0.05938372350927861171, 21.12180007765648071, -3.680117784833935701 ) ) ;
#4042=CARTESIAN_POINT ( 'NONE',  ( -2.864755990943265829, 35.74680007765648071, -2.011557305968488141 ) ) ;
#4043=ORIENTED_EDGE ( 'NONE', *, *, #379, .F. ) ;
#4047=CARTESIAN_POINT ( 'NONE',  ( 1.336863392178569754, 38.75319992234354061, 4.297206761780648421 ) ) ;
#4049=CARTESIAN_POINT ( 'NONE',  ( -1.497042530366522461, 27.37819992234355126, -2.161531897785030409 ) ) ;
#4052=CARTESIAN_POINT ( 'NONE',  ( -4.518350579753632523, 28.12180007765647716, -1.405661355842698468 ) ) ;
#4072=CARTESIAN_POINT ( 'NONE',  ( 1.135272562821020070, 35.25319992234354771, -3.311245368580577164 ) ) ;
#4073=CARTESIAN_POINT ( 'NONE',  ( -1.027846397803611866, 20.00319992234354416, -3.346150245485499219 ) ) ;
#4075=CARTESIAN_POINT ( 'NONE',  ( 2.481649420246374138, 31.62180007765648426, -0.8687765177876252132 ) ) ;
#4078=CARTESIAN_POINT ( 'NONE',  ( -0.05938372350918959958, 26.37819992234355126, 4.731580009072201776 ) ) ;
#4082=CARTESIAN_POINT ( 'NONE',  ( 2.211161402132902243, 19.62180007765647360, 2.942372952327172442 ) ) ;
#4094=CARTESIAN_POINT ( 'NONE',  ( -2.798362969681365886, 25.24680007765647716, 2.102939460078824929 ) ) ;
#4100=CARTESIAN_POINT ( 'NONE',  ( -2.500000000000001332, 34.50319992234354771, -0.05647727720530596601 ) ) ;
#4102=CARTESIAN_POINT ( 'NONE',  ( 2.211161402132902243, 32.12180007765647360, 2.942372952327172442 ) ) ;
#4103=CARTESIAN_POINT ( 'NONE',  ( -2.115076519116425580, 24.87819992234354771, -3.012182706137062738 ) ) ;
#4121=CARTESIAN_POINT ( 'NONE',  ( -0.8262555684461330152, 35.99680007765648071, -2.360188852285403982 ) ) ;
#4124=CARTESIAN_POINT ( 'NONE',  ( 2.864755990943265829, 36.99680007765648071, 2.011557305968487697 ) ) ;
#4130=CARTESIAN_POINT ( 'NONE',  ( 3.481649420246369697, 34.12180007765648071, -1.193696214020541824 ) ) ;
#4141=CARTESIAN_POINT ( 'NONE',  ( 2.481649420246374138, 16.62180007765648071, -0.8687765177876252132 ) ) ;
#4147=CARTESIAN_POINT ( 'NONE',  ( -3.607379964056306676, 17.74680007765647716, 2.690724712371306282 ) ) ;
#4149=CARTESIAN_POINT ( 'NONE',  ( -3.500000000000000444, 14.50319992234354416, -0.05647727720529563400 ) ) ;
#4152=CARTESIAN_POINT ( 'NONE',  ( 2.829195390882805583, 34.62180007765646650, 3.793023760679204770 ) ) ;
#4170=CARTESIAN_POINT ( 'NONE',  ( -1.336863392178569088, 17.50319992234354771, -4.297206761780648421 ) ) ;
#4171=CARTESIAN_POINT ( 'NONE',  ( -1.135272562821019626, 19.00319992234354771, 3.311245368580577164 ) ) ;
#4173=CARTESIAN_POINT ( 'NONE',  ( 1.593127413382998903, 34.62180007765648071, 2.091722143975139669 ) ) ;
#4175=CARTESIAN_POINT ( 'NONE',  ( 4.518350579753602325, 23.12819992234354416, -1.405661355842793725 ) ) ;
#4179=CARTESIAN_POINT ( 'NONE',  ( -2.211161402132902243, 23.37180007765647716, -2.942372952327172886 ) ) ;
#4188=CARTESIAN_POINT ( 'NONE',  ( -1.135272562821090014, 20.99680007765647716, -3.311245368580554072 ) ) ;
#4194=CARTESIAN_POINT ( 'NONE',  ( 3.518350579753605434, 15.62819992234354416, -1.080741659609877114 ) ) ;
#4196=CARTESIAN_POINT ( 'NONE',  ( -2.864755990943265829, 33.24680007765648071, -2.011557305968488141 ) ) ;
#4197=CARTESIAN_POINT ( 'NONE',  ( -0.05938372350920063936, 26.37819992234354061, 3.680117784833935701 ) ) ;
#4210=CARTESIAN_POINT ( 'NONE',  ( 2.500000000000001332, 39.24680007765647360, -0.05647727720535888202 ) ) ;
#4212=CARTESIAN_POINT ( 'NONE',  ( 3.518350579753631191, 39.37180007765646650, 1.080741659609802729 ) ) ;
#4219=CARTESIAN_POINT ( 'NONE',  ( 1.135272562821090458, 34.74680007765648071, 3.311245368580554072 ) ) ;
#4235=CARTESIAN_POINT ( 'NONE',  ( 0.05938372350927906274, 39.87180007765648071, 3.680117784833935701 ) ) ;
#4240=CARTESIAN_POINT ( 'NONE',  ( -1.593127413382952939, 36.62819992234354771, 2.091722143975172532 ) ) ;
#4244=CARTESIAN_POINT ( 'NONE',  ( 2.829195390882805583, 32.12180007765646650, 3.793023760679204770 ) ) ;
#4259=CARTESIAN_POINT ( 'NONE',  ( 0.05938372350919016857, 15.12819992234354594, -4.731580009072201776 ) ) ;
#4260=CARTESIAN_POINT ( 'NONE',  ( -2.211161402132838738, 24.12819992234354416, 2.942372952327218183 ) ) ;
#4262=CARTESIAN_POINT ( 'NONE',  ( -2.481649420246391902, 14.62819992234354594, -0.8687765177875723666 ) ) ;
#4263=CARTESIAN_POINT ( 'NONE',  ( 4.481649420246397675, 30.87819992234354061, 1.518615910253363177 ) ) ;
#4268=CARTESIAN_POINT ( 'NONE',  ( -3.500000000000000444, 25.49680007765647716, 0.05647727720536892260 ) ) ;
#4271=CARTESIAN_POINT ( 'NONE',  ( 4.481649420246366589, 21.62180007765647716, -1.518615910253458212 ) ) ;
#4276=CARTESIAN_POINT ( 'NONE',  ( -1.027846397803541700, 22.49680007765648071, 3.346150245485522312 ) ) ;
#4282=CARTESIAN_POINT ( 'NONE',  ( -2.798362969681409851, 22.25319992234354416, -2.102939460078765421 ) ) ;
#4284=CARTESIAN_POINT ( 'NONE',  ( 0.05938372350927906274, 39.87180007765648071, 3.680117784833935701 ) ) ;
#4285=CARTESIAN_POINT ( 'NONE',  ( -0.05938372350920063936, 33.87819992234354771, 3.680117784833935701 ) ) ;
#4297=CARTESIAN_POINT ( 'NONE',  ( 0.8262555684460829442, 22.75319992234354771, -2.360188852285421302 ) ) ;
#4299=CARTESIAN_POINT ( 'NONE',  ( 0.05938372350927906274, 17.37180007765647005, 3.680117784833935701 ) ) ;
#4304=CARTESIAN_POINT ( 'NONE',  ( 3.518350579753631191, 34.37180007765648071, 1.080741659609802285 ) ) ;
#4315=CARTESIAN_POINT ( 'NONE',  ( 0.8262555684461332373, 19.74680007765648071, 2.360188852285403982 ) ) ;
#4321=CARTESIAN_POINT ( 'NONE',  ( 1.989345975306457071, 38.50319992234354771, 1.515154207786300500 ) ) ;
#4322=( BOUNDED_CURVE ( )  B_SPLINE_CURVE ( 2, ( #3451, #17836, #13361, #9364, #15040, #13630, #6586, #7700, #11969, #17661, #16249, #5381, #18205, #9457, #12420, #1397, #5469, #3986, #5557, #11114, #13911, #2792, #14085, #11205, #7025, #5648, #6762, #8154, #15130, #16894, #12510, #2612, #2434, #2705, #4171, #16803, #8060, #13723, #18014, #16713, #5286, #18111, #4073, #3899, #9635, #8337, #15224, #9725, #973, #10941, #1219, #3802, #9814, #1034, #11030, #15313, #15410, #8252, #18284, #6856, #13996, #1311, #12689, #15495, #8423, #11291, #6943, #6674, #12596, #12328, #16624, #9546, #2524, #13816, #1127, #4260, #4532, #9903, #6008, #3245, #2875, #461, #14365, #12779, #6102, #4438, #2963, #8688, #1664, #7300, #369, #14178, #12960, #8597, #14464, #174, #275, #15574, #7213, #14561, #5919, #88, #13150, #3057, #10174, #15948, #8883, #11663, #1861, #16983, #1575, #14272, #8505, #17355, #11564, #15757, #1485, #15851, #4618, #17259, #7119, #3149, #7492, #13058, #4343, #12867, #8783, #17068, #10078, #1767, #9990, #7398, #5741, #11381, #10268, #15665, #5825, #11470, #17164, #14750, #4990, #651, #3430, #11850, #10646, #6295, #3695, #6471, #16411, #9341, #10549, #3604, #17546, #9254, #9071, #10737, #16225, #16318, #14939, #12031, #13607, #2231, #12123, #2319, #3518, #11948, #7677, #15019, #17448, #830, #1957, #7950, #9165, #4716, #14846, #14657, #8984, #7583, #921, #6388, #17817, #559, #5078, #7857, #13241, #10367, #16046, #10463, #6201, #3338, #4815, #11754, #13430, #17642, #13514, #744, #2139, #17724, #7770 ),
 .UNSPECIFIED., .F., .F. ) 
 B_SPLINE_CURVE_WITH_KNOTS ( ( 3, 2, 2, 2, 2, 2, 2, 2, 2, 2, 2, 2, 2, 2, 2, 2, 2, 2, 2, 2, 2, 2, 2, 2, 2, 2, 2, 2, 2, 2, 2, 2, 2, 2, 2, 2, 2, 2, 2, 2, 2, 2, 2, 2, 2, 2, 2, 2, 2, 2, 2, 2, 2, 2, 2, 2, 2, 2, 2, 2, 2, 2, 2, 2, 2, 2, 2, 2, 2, 2, 2, 2, 2, 2, 2, 2, 2, 2, 2, 2, 2, 2, 2, 2, 2, 2, 2, 2, 2, 2, 2, 2, 2, 2, 2, 2, 2, 2, 2, 3 ),
 ( 0.01986568351594109050, 0.02000000000000000042, 0.02999999999999999889, 0.04000000000000000083, 0.05000000000000000278, 0.05999999999999999778, 0.07000000000000000666, 0.08000000000000000167, 0.08999999999999999667, 0.1000000000000000056, 0.1100000000000000006, 0.1199999999999999956, 0.1300000000000000044, 0.1400000000000000133, 0.1499999999999999944, 0.1600000000000000033, 0.1699999999999999845, 0.1799999999999999933, 0.1900000000000000022, 0.2000000000000000111, 0.2099999999999999922, 0.2200000000000000289, 0.2300000000000000100, 0.2399999999999999911, 0.2500000000000000000, 0.2600000000000000089, 0.2700000000000000178, 0.2800000000000000266, 0.2899999999999999800, 0.2999999999999999889, 0.3099999999999999978, 0.3200000000000000067, 0.3300000000000000155, 0.3400000000000000244, 0.3499999999999999778, 0.3599999999999999867, 0.3699999999999999956, 0.3800000000000000044, 0.3900000000000000133, 0.4000000000000000222, 0.4099999999999999756, 0.4199999999999999845, 0.4299999999999999933, 0.4400000000000000022, 0.4500000000000000111, 0.4600000000000000200, 0.4699999999999999734, 0.4799999999999999822, 0.4899999999999999911, 0.5000000000000000000, 0.5100000000000000089, 0.5200000000000000178, 0.5300000000000000266, 0.5400000000000000355, 0.5500000000000000444, 0.5600000000000000533, 0.5699999999999999512, 0.5799999999999999600, 0.5899999999999999689, 0.5999999999999999778, 0.6099999999999999867, 0.6199999999999999956, 0.6300000000000000044, 0.6400000000000000133, 0.6500000000000000222, 0.6600000000000000311, 0.6700000000000000400, 0.6800000000000000488, 0.6899999999999999467, 0.6999999999999999556, 0.7099999999999999645, 0.7199999999999999734, 0.7299999999999999822, 0.7399999999999999911, 0.7500000000000000000, 0.7600000000000000089, 0.7700000000000000178, 0.7800000000000000266, 0.7900000000000000355, 0.8000000000000000444, 0.8100000000000000533, 0.8199999999999999512, 0.8299999999999999600, 0.8399999999999999689, 0.8499999999999999778, 0.8599999999999999867, 0.8699999999999999956, 0.8800000000000000044, 0.8900000000000000133, 0.9000000000000000222, 0.9100000000000000311, 0.9200000000000000400, 0.9300000000000000488, 0.9399999999999999467, 0.9499999999999999556, 0.9599999999999999645, 0.9699999999999999734, 0.9799999999999999822, 0.9899999999999999911, 1.000000000000000000 ),
 .UNSPECIFIED. ) 
 CURVE ( )  GEOMETRIC_REPRESENTATION_ITEM ( )  RATIONAL_B_SPLINE_CURVE ( ( 0.9987028763776494289, 0.9993426083351170108, 1.000000000000000000, 0.9510565162951535312, 1.000000000000000000, 0.9510565162951535312, 1.000000000000000000, 0.9510565162951535312, 1.000000000000000000, 0.9510565162951535312, 1.000000000000000000, 0.9510565162951535312, 1.000000000000000000, 0.9510565162951535312, 1.000000000000000000, 0.9510565162951535312, 1.000000000000000000, 0.9510565162951535312, 1.000000000000000000, 0.9510565162951535312, 1.000000000000000000, 0.9510565162951535312, 1.000000000000000000, 0.9510565162951535312, 1.000000000000000000, 0.9510565162951535312, 1.000000000000000000, 0.9510565162951535312, 1.000000000000000000, 0.9510565162951535312, 1.000000000000000000, 0.9510565162951535312, 1.000000000000000000, 0.9510565162951535312, 1.000000000000000000, 0.9510565162951535312, 1.000000000000000000, 0.9510565162951535312, 1.000000000000000000, 0.9510565162951535312, 1.000000000000000000, 0.9510565162951535312, 1.000000000000000000, 0.9510565162951535312, 1.000000000000000000, 0.9510565162951535312, 1.000000000000000000, 0.9510565162951535312, 1.000000000000000000, 0.9510565162951535312, 1.000000000000000000, 0.9510565162951535312, 1.000000000000000000, 0.9510565162951535312, 1.000000000000000000, 0.9510565162951535312, 1.000000000000000000, 0.9510565162951535312, 1.000000000000000000, 0.9510565162951535312, 1.000000000000000000, 0.9510565162951535312, 1.000000000000000000, 0.9510565162951535312, 1.000000000000000000, 0.9510565162951535312, 1.000000000000000000, 0.9510565162951535312, 1.000000000000000000, 0.9510565162951535312, 1.000000000000000000, 0.9510565162951535312, 1.000000000000000000, 0.9510565162951535312, 1.000000000000000000, 0.9510565162951535312, 1.000000000000000000, 0.9510565162951535312, 1.000000000000000000, 0.9510565162951535312, 1.000000000000000000, 0.9510565162951535312, 1.000000000000000000, 0.9510565162951535312, 1.000000000000000000, 0.9510565162951535312, 1.000000000000000000, 0.9510565162951535312, 1.000000000000000000, 0.9510565162951535312, 1.000000000000000000, 0.9510565162951535312, 1.000000000000000000, 0.9510565162951535312, 1.000000000000000000, 0.9510565162951535312, 1.000000000000000000, 0.9510565162951535312, 1.000000000000000000, 0.9510565162951535312, 1.000000000000000000, 0.9510565162951535312, 1.000000000000000000, 0.9510565162951535312, 1.000000000000000000, 0.9510565162951535312, 1.000000000000000000, 0.9510565162951535312, 1.000000000000000000, 0.9510565162951535312, 1.000000000000000000, 0.9510565162951535312, 1.000000000000000000, 0.9510565162951535312, 1.000000000000000000, 0.9510565162951535312, 1.000000000000000000, 0.9510565162951535312, 1.000000000000000000, 0.9510565162951535312, 1.000000000000000000, 0.9510565162951535312, 1.000000000000000000, 0.9510565162951535312, 1.000000000000000000, 0.9510565162951535312, 1.000000000000000000, 0.9510565162951535312, 1.000000000000000000, 0.9510565162951535312, 1.000000000000000000, 0.9510565162951535312, 1.000000000000000000, 0.9510565162951535312, 1.000000000000000000, 0.9510565162951535312, 1.000000000000000000, 0.9510565162951535312, 1.000000000000000000, 0.9510565162951535312, 1.000000000000000000, 0.9510565162951535312, 1.000000000000000000, 0.9510565162951535312, 1.000000000000000000, 0.9510565162951535312, 1.000000000000000000, 0.9510565162951535312, 1.000000000000000000, 0.9510565162951535312, 1.000000000000000000, 0.9510565162951535312, 1.000000000000000000, 0.9510565162951535312, 1.000000000000000000, 0.9510565162951535312, 1.000000000000000000, 0.9510565162951535312, 1.000000000000000000, 0.9510565162951535312, 1.000000000000000000, 0.9510565162951535312, 1.000000000000000000, 0.9510565162951535312, 1.000000000000000000, 0.9510565162951535312, 1.000000000000000000, 0.9510565162951535312, 1.000000000000000000, 0.9510565162951535312, 1.000000000000000000, 0.9510565162951535312, 1.000000000000000000, 0.9510565162951535312, 1.000000000000000000, 0.9510565162951535312, 1.000000000000000000, 0.9510565162951535312, 1.000000000000000000, 0.9510565162951535312, 1.000000000000000000, 0.9510565162951535312, 1.000000000000000000, 0.9510565162951535312, 1.000000000000000000, 0.9510565162951535312, 1.000000000000000000, 0.9510565162951535312, 1.000000000000000000, 0.9510565162951535312, 1.000000000000000000, 0.9510565162951535312, 1.000000000000000000, 0.9510565162951535312, 1.000000000000000000, 0.9510565162951535312, 1.000000000000000000, 0.9510565162951535312, 1.000000000000000000 ) ) 
 REPRESENTATION_ITEM ( '' )  );
#4325=CARTESIAN_POINT ( 'NONE',  ( 2.733110507866247652, 33.87180007765647360, -3.862833514489153686 ) ) ;
#4341=FILL_AREA_STYLE ('',( #1309 ) ) ;
#4342=CARTESIAN_POINT ( 'NONE',  ( -3.607379964056363075, 19.75319992234354416, -2.690724712371229899 ) ) ;
#4343=CARTESIAN_POINT ( 'NONE',  ( 1.135272562821020070, 30.25319992234354416, -3.311245368580577164 ) ) ;
#4344=CARTESIAN_POINT ( 'NONE',  ( 1.593127413382998903, 37.12180007765648071, 2.091722143975139669 ) ) ;
#4346=CARTESIAN_POINT ( 'NONE',  ( 0.05938372350919016857, 30.12819992234354061, -4.731580009072201776 ) ) ;
#4351=CARTESIAN_POINT ( 'NONE',  ( 2.211161402132902243, 29.62180007765648071, 2.942372952327172442 ) ) ;
#4355=CARTESIAN_POINT ( 'NONE',  ( 4.499999999999999112, 34.24680007765646650, -0.05647727720537982360 ) ) ;
#4359=CARTESIAN_POINT ( 'NONE',  ( -3.518350579753630747, 25.62180007765648071, -1.080741659609802729 ) ) ;
#4364=CARTESIAN_POINT ( 'NONE',  ( -3.518350579753605434, 16.87819992234353705, 1.080741659609877781 ) ) ;
#4367=CARTESIAN_POINT ( 'NONE',  ( -3.500000000000000444, 40.49680007765648071, 0.05647727720536892260 ) ) ;
#4368=CARTESIAN_POINT ( 'NONE',  ( 1.135272562821020070, 37.75319992234354061, -3.311245368580577164 ) ) ;
#4386=CARTESIAN_POINT ( 'NONE',  ( 0.05938372350921204690, 22.62819992234354771, -2.628655560595669183 ) ) ;
#4389=CARTESIAN_POINT ( 'NONE',  ( 3.481649420246369697, 19.12180007765648071, -1.193696214020541824 ) ) ;
#4398=CARTESIAN_POINT ( 'NONE',  ( -1.027846397803541700, 34.99680007765648071, 3.346150245485522312 ) ) ;
#4409=CARTESIAN_POINT ( 'NONE',  ( 2.481649420246374138, 19.12180007765648071, -0.8687765177876252132 ) ) ;
#4411=CARTESIAN_POINT ( 'NONE',  ( -2.211161402132901799, 23.37180007765647716, -2.942372952327172886 ) ) ;
#4415=CARTESIAN_POINT ( 'NONE',  ( 1.593127413382953383, 35.37819992234354061, -2.091722143975172532 ) ) ;
#4419=CARTESIAN_POINT ( 'NONE',  ( -4.481649420246366589, 30.37180007765647716, 1.518615910253458878 ) ) ;
#4436=PRESENTATION_STYLE_ASSIGNMENT (( #16892 ) ) ;
#4437=CARTESIAN_POINT ( 'NONE',  ( 2.829195390882724759, 17.87819992234354416, -3.793023760679264278 ) ) ;
#4438=CARTESIAN_POINT ( 'NONE',  ( 2.211161402132839182, 25.37819992234354416, -2.942372952327217739 ) ) ;
#4439=CARTESIAN_POINT ( 'NONE',  ( -2.518350579753628526, 38.12180007765647360, -0.7558219633769075463 ) ) ;
#4441=CARTESIAN_POINT ( 'NONE',  ( -4.481649420246396787, 32.12819992234354771, -1.518615910253363399 ) ) ;
#4448=CARTESIAN_POINT ( 'NONE',  ( -2.115076519116362519, 27.62180007765648071, 3.012182706137107147 ) ) ;
#4452=CARTESIAN_POINT ( 'NONE',  ( -2.733110507866247652, 35.12180007765647360, 3.862833514489154574 ) ) ;
#4457=CARTESIAN_POINT ( 'NONE',  ( 3.481649420246369697, 21.62180007765647360, -1.193696214020541824 ) ) ;
#4462=CARTESIAN_POINT ( 'NONE',  ( 1.027846397803612311, 16.25319992234354416, 3.346150245485499219 ) ) ;
#4465=CARTESIAN_POINT ( 'NONE',  ( -1.135272562821090014, 35.99680007765648071, -3.311245368580554072 ) ) ;
#4466=CARTESIAN_POINT ( 'NONE',  ( 1.027846397803612311, 31.25319992234354416, 3.346150245485499219 ) ) ;
#4476=CARTESIAN_POINT ( 'NONE',  ( -1.252219993090138761, 15.00000000000000355, -3.080002712724053904 ) ) ;
#4480=CARTESIAN_POINT ( 'NONE',  ( 0.05938372350921204690, 20.12819992234354771, -2.628655560595669183 ) ) ;
#4483=CARTESIAN_POINT ( 'NONE',  ( 3.607379964056306676, 18.99680007765647716, -2.690724712371305838 ) ) ;
#4489=CARTESIAN_POINT ( 'NONE',  ( -2.211161402132902243, 33.37180007765648071, -2.942372952327172886 ) ) ;
#4502=CARTESIAN_POINT ( 'NONE',  ( 2.055738996568313048, 19.49680007765648071, 1.423772053676023441 ) ) ;
#4504=CARTESIAN_POINT ( 'NONE',  ( 2.211161402132902243, 22.12180007765648071, 2.942372952327172442 ) ) ;
#4509=CARTESIAN_POINT ( 'NONE',  ( -0.05938372350921170689, 38.87819992234354771, 2.628655560595669183 ) ) ;
#4512=CARTESIAN_POINT ( 'NONE',  ( 4.481649420246366589, 34.12180007765647360, -1.518615910253458212 ) ) ;
#4531=CARTESIAN_POINT ( 'NONE',  ( -1.336863392178569088, 15.00319992234354594, -4.297206761780648421 ) ) ;
#4532=CARTESIAN_POINT ( 'NONE',  ( -2.864755990943222308, 24.25319992234354416, 2.011557305968548093 ) ) ;
#4533=CARTESIAN_POINT ( 'NONE',  ( 2.500000000000001332, 36.74680007765648071, -0.05647727720535888202 ) ) ;
#4536=CARTESIAN_POINT ( 'NONE',  ( -4.518350579753602325, 34.37819992234354771, 1.405661355842794391 ) ) ;
#4541=CARTESIAN_POINT ( 'NONE',  ( 2.115076519116362963, 33.87180007765648071, -3.012182706137107147 ) ) ;
#4544=CARTESIAN_POINT ( 'NONE',  ( -4.499999999999999112, 27.99680007765647716, 0.05647727720537927543 ) ) ;
#4549=CARTESIAN_POINT ( 'NONE',  ( -2.115076519116362519, 30.12180007765647360, 3.012182706137107147 ) ) ;
#4554=CARTESIAN_POINT ( 'NONE',  ( 2.864755990943222308, 23.00319992234354416, -2.011557305968548093 ) ) ;
#4558=CARTESIAN_POINT ( 'NONE',  ( -2.798362969681365886, 40.24680007765648071, 2.102939460078824929 ) ) ;
#4560=CARTESIAN_POINT ( 'NONE',  ( 3.481649420246394122, 30.87819992234353350, 1.193696214020467439 ) ) ;
#4562=EDGE_CURVE ( 'NONE', #6875, #13000, #4322, .T. ) ;
#4573=CARTESIAN_POINT ( 'NONE',  ( -2.518350579753611207, 16.87819992234354416, 0.7558219633769609480 ) ) ;
#4579=CARTESIAN_POINT ( 'NONE',  ( 3.518350579753631191, 36.87180007765645939, 1.080741659609802285 ) ) ;
#4589=CARTESIAN_POINT ( 'NONE',  ( -2.500000000000001332, 22.99680007765648071, 0.05647727720535858364 ) ) ;
#4591=CARTESIAN_POINT ( 'NONE',  ( 3.481649420246370141, 21.62180007765647360, -1.193696214020541602 ) ) ;
#4595=CARTESIAN_POINT ( 'NONE',  ( 3.500000000000000444, 18.25319992234354771, 0.05647727720529520379 ) ) ;
#4598=CARTESIAN_POINT ( 'NONE',  ( 2.864755990943265829, 16.99680007765647716, 2.011557305968487697 ) ) ;
#4617=CARTESIAN_POINT ( 'NONE',  ( 0.05938372350919016857, 30.12819992234354061, -4.731580009072201776 ) ) ;
#4618=CARTESIAN_POINT ( 'NONE',  ( -3.500000000000000444, 29.50319992234354416, -0.05647727720529563400 ) ) ;
#4621=CARTESIAN_POINT ( 'NONE',  ( 0.05938372350921204690, 22.62819992234354771, -2.628655560595669183 ) ) ;
#4623=CARTESIAN_POINT ( 'NONE',  ( 3.607379964056363075, 31.00319992234354771, 2.690724712371229010 ) ) ;
#4628=CARTESIAN_POINT ( 'NONE',  ( -2.115076519116362519, 32.62180007765646650, 3.012182706137107147 ) ) ;
#4632=CARTESIAN_POINT ( 'NONE',  ( 1.444289557196047680, 27.24680007765647716, 4.262301884875704161 ) ) ;
#4635=CARTESIAN_POINT ( 'NONE',  ( 0.05938372350927906274, 32.37180007765647360, 3.680117784833935701 ) ) ;
#4640=CARTESIAN_POINT ( 'NONE',  ( 2.798362969681409851, 26.00319992234354771, 2.102939460078764977 ) ) ;
#4643=CARTESIAN_POINT ( 'NONE',  ( 1.135272562821090458, 39.74680007765648071, 3.311245368580554072 ) ) ;
#4644=CARTESIAN_POINT ( 'NONE',  ( 2.115076519116426024, 31.12819992234354061, 3.012182706137062294 ) ) ;
#4662=CARTESIAN_POINT ( 'NONE',  ( -2.055738996568281518, 29.25319992234355126, 1.423772053676066962 ) ) ;
#4664=FACE_OUTER_BOUND ( 'NONE', #17182, .T. ) ;
#4668=CARTESIAN_POINT ( 'NONE',  ( 3.518350579753631191, 39.37180007765646650, 1.080741659609802285 ) ) ;
#4683=CARTESIAN_POINT ( 'NONE',  ( -1.497042530366477164, 20.12180007765648071, 2.161531897785062384 ) ) ;
#4687=CARTESIAN_POINT ( 'NONE',  ( -3.518350579753630303, 18.12180007765647716, -1.080741659609802952 ) ) ;
#4691=CARTESIAN_POINT ( 'NONE',  ( 2.864755990943222308, 20.50319992234354416, -2.011557305968548093 ) ) ;
#4694=CARTESIAN_POINT ( 'NONE',  ( 2.115076519116362963, 18.87180007765648071, -3.012182706137107147 ) ) ;
#4715=CARTESIAN_POINT ( 'NONE',  ( -2.829195390882724315, 24.12819992234354771, 3.793023760679264722 ) ) ;
#4716=CARTESIAN_POINT ( 'NONE',  ( -0.05938372350920064630, 36.37819992234354771, 3.680117784833935701 ) ) ;
#4718=CARTESIAN_POINT ( 'NONE',  ( 1.593127413382953383, 22.87819992234354771, -2.091722143975172532 ) ) ;
#4720=CARTESIAN_POINT ( 'NONE',  ( 4.481649420246366589, 19.12180007765647360, -1.518615910253458212 ) ) ;
#4724=CARTESIAN_POINT ( 'NONE',  ( -2.115076519116362519, 30.12180007765647360, 3.012182706137107147 ) ) ;
#4730=CARTESIAN_POINT ( 'NONE',  ( -4.481649420246366589, 32.87180007765647360, 1.518615910253458878 ) ) ;
#4734=CARTESIAN_POINT ( 'NONE',  ( 1.027846397803542144, 33.74680007765648071, -3.346150245485522312 ) ) ;
#4740=CARTESIAN_POINT ( 'NONE',  ( -2.115076519116425580, 24.87819992234354771, -3.012182706137062738 ) ) ;
#4743=CARTESIAN_POINT ( 'NONE',  ( 0.7188294034286049072, 18.74680007765648071, -2.395093729190366005 ) ) ;
#4745=CARTESIAN_POINT ( 'NONE',  ( 4.481649420246397675, 18.37819992234354416, 1.518615910253363177 ) ) ;
#4760=CARTESIAN_POINT ( 'NONE',  ( 1.497042530366522461, 31.12819992234354416, 2.161531897785029965 ) ) ;
#4762=CARTESIAN_POINT ( 'NONE',  ( -1.135272562821090014, 23.49680007765647716, -3.311245368580554072 ) ) ;
#4766=CARTESIAN_POINT ( 'NONE',  ( 2.115076519116362963, 38.87180007765645939, -3.012182706137107147 ) ) ;
#4777=CARTESIAN_POINT ( 'NONE',  ( -2.055738996568313048, 28.24680007765648071, -1.423772053676023441 ) ) ;
#4779=CARTESIAN_POINT ( 'NONE',  ( -3.518350579753630303, 30.62180007765647716, -1.080741659609802952 ) ) ;
#4786=CARTESIAN_POINT ( 'NONE',  ( 0.05938372350920109732, 17.62819992234354771, -3.680117784833935701 ) ) ;
#4790=CARTESIAN_POINT ( 'NONE',  ( 1.135272562821090458, 17.24680007765647716, 3.311245368580554072 ) ) ;
#4814=CARTESIAN_POINT ( 'NONE',  ( -4.518350579753602325, 24.37819992234354416, 1.405661355842794391 ) ) ;
#4815=CARTESIAN_POINT ( 'NONE',  ( 2.798362969681409851, 38.50319992234354061, 2.102939460078764977 ) ) ;
#4816=CARTESIAN_POINT ( 'NONE',  ( -2.500000000000001332, 17.00319992234354416, -0.05647727720530596601 ) ) ;
#4818=CARTESIAN_POINT ( 'NONE',  ( -2.829195390882805139, 20.87180007765647716, -3.793023760679206102 ) ) ;
#4836=CARTESIAN_POINT ( 'NONE',  ( 2.115076519116426024, 28.62819992234353705, 3.012182706137062294 ) ) ;
#4839=CARTESIAN_POINT ( 'NONE',  ( 1.497042530366477164, 21.37180007765648071, -2.161531897785062384 ) ) ;
#4840=CARTESIAN_POINT ( 'NONE',  ( 3.673772985318163098, 20.50319992234354771, -2.599342558261029001 ) ) ;
#4854=CARTESIAN_POINT ( 'NONE',  ( -1.989345975306457071, 27.25319992234354771, -1.515154207786300944 ) ) ;
#4857=CARTESIAN_POINT ( 'NONE',  ( -1.135272562821090014, 25.99680007765648071, -3.311245368580554072 ) ) ;
#4859=PRODUCT ( 'Return Spring', 'Return Spring', '', ( #16294 ) ) ;
#4872=CARTESIAN_POINT ( 'NONE',  ( 2.481649420246374138, 29.12180007765648426, -0.8687765177876252132 ) ) ;
#4874=CARTESIAN_POINT ( 'NONE',  ( -3.481649420246370141, 32.87180007765647360, 1.193696214020542268 ) ) ;
#4877=CARTESIAN_POINT ( 'NONE',  ( 2.115076519116426024, 16.12819992234354416, 3.012182706137062294 ) ) ;
#4880=CARTESIAN_POINT ( 'NONE',  ( -1.027846397803541700, 17.49680007765647716, 3.346150245485522312 ) ) ;
#4898=CARTESIAN_POINT ( 'NONE',  ( -4.481649420246396787, 29.62819992234354416, -1.518615910253363399 ) ) ;
#4900=CARTESIAN_POINT ( 'NONE',  ( 1.497042530366522461, 21.12819992234354416, 2.161531897785029965 ) ) ;
#4903=CARTESIAN_POINT ( 'NONE',  ( -4.481649420246366589, 20.37180007765648071, 1.518615910253458878 ) ) ;
#4907=CARTESIAN_POINT ( 'NONE',  ( 2.864755990943265829, 39.49680007765647360, 2.011557305968487697 ) ) ;
#4922=CARTESIAN_POINT ( 'NONE',  ( 3.500000000000000444, 30.75319992234354416, 0.05647727720529520379 ) ) ;
#4925=CARTESIAN_POINT ( 'NONE',  ( -2.481649420246374138, 25.37180007765648426, 0.8687765177876256573 ) ) ;
#4926=CARTESIAN_POINT ( 'NONE',  ( 3.673772985318163098, 15.50319992234354416, -2.599342558261029001 ) ) ;
#4931=CARTESIAN_POINT ( 'NONE',  ( 1.444289557196047680, 39.74680007765648071, 4.262301884875704161 ) ) ;
#4941=CARTESIAN_POINT ( 'NONE',  ( 1.989345975306457071, 31.00319992234355126, 1.515154207786300500 ) ) ;
#4945=CARTESIAN_POINT ( 'NONE',  ( 1.027846397803542144, 23.74680007765647716, -3.346150245485522312 ) ) ;
#4960=CARTESIAN_POINT ( 'NONE',  ( -1.497042530366477164, 27.62180007765648426, 2.161531897785062384 ) ) ;
#4962=CARTESIAN_POINT ( 'NONE',  ( 2.864755990943265829, 26.99680007765648071, 2.011557305968487697 ) ) ;
#4969=CARTESIAN_POINT ( 'NONE',  ( -1.135272562821090014, 15.99680007765647716, -3.311245368580554072 ) ) ;
#4989=CARTESIAN_POINT ( 'NONE',  ( 2.733110507866328920, 36.12819992234354771, 3.862833514489095510 ) ) ;
#4990=CARTESIAN_POINT ( 'NONE',  ( -2.798362969681409851, 32.25319992234354771, -2.102939460078765421 ) ) ;
#4991=CARTESIAN_POINT ( 'NONE',  ( 2.518350579753611207, 20.62819992234354771, -0.7558219633769606149 ) ) ;
#4994=CARTESIAN_POINT ( 'NONE',  ( -3.673772985318163098, 39.25319992234354771, 2.599342558261029001 ) ) ;
#4999=CARTESIAN_POINT ( 'NONE',  ( -2.211161402132902243, 38.37180007765648071, -2.942372952327172886 ) ) ;
#5011=CARTESIAN_POINT ( 'NONE',  ( 0.05938372350920109732, 25.12819992234354416, -3.680117784833935701 ) ) ;
#5014=CARTESIAN_POINT ( 'NONE',  ( 1.593127413382998903, 22.12180007765648071, 2.091722143975139669 ) ) ;
#5016=CARTESIAN_POINT ( 'NONE',  ( 4.481649420246397675, 15.87819992234354061, 1.518615910253363177 ) ) ;
#5023=CARTESIAN_POINT ( 'NONE',  ( -2.115076519116362519, 17.62180007765647716, 3.012182706137107147 ) ) ;
#5035=CARTESIAN_POINT ( 'NONE',  ( -1.593127413382952939, 26.62819992234354416, 2.091722143975172532 ) ) ;
#5037=CARTESIAN_POINT ( 'NONE',  ( -0.05938372350927861171, 26.12180007765647005, -3.680117784833935701 ) ) ;
#5043=DIRECTION ( 'NONE',  ( 0.000000000000000000, 0.9936001553129348851, 0.1129545544106647231 ) ) ;
#5050=CARTESIAN_POINT ( 'NONE',  ( -2.500000000000001332, 32.99680007765648071, 0.05647727720535858364 ) ) ;
#5052=CARTESIAN_POINT ( 'NONE',  ( 3.518350579753631191, 31.87180007765647716, 1.080741659609802729 ) ) ;
#5057=DIRECTION ( 'NONE',  ( 1.028113302204111856E-14, -0.1129545544106654864, 0.9936001553129347741 ) ) ;
#5060=CARTESIAN_POINT ( 'NONE',  ( -3.500000000000000444, 20.49680007765647716, 0.05647727720536892260 ) ) ;
#5073=CARTESIAN_POINT ( 'NONE',  ( -2.115076519116362519, 35.12180007765645939, 3.012182706137107147 ) ) ;
#5077=CARTESIAN_POINT ( 'NONE',  ( -2.829195390882724315, 34.12819992234354771, 3.793023760679264722 ) ) ;
#5078=CARTESIAN_POINT ( 'NONE',  ( -1.027846397803611866, 37.50319992234354061, -3.346150245485499219 ) ) ;
#5079=CARTESIAN_POINT ( 'NONE',  ( 0.7188294034286553114, 28.75319992234354771, 2.395093729190349130 ) ) ;
#5081=CARTESIAN_POINT ( 'NONE',  ( 2.829195390882805583, 19.62180007765647716, 3.793023760679204770 ) ) ;
#5086=CARTESIAN_POINT ( 'NONE',  ( -2.115076519116362519, 37.62180007765648071, 3.012182706137107147 ) ) ;
#5099=CARTESIAN_POINT ( 'NONE',  ( 1.027846397803612311, 38.75319992234354061, 3.346150245485499219 ) ) ;
#5102=CARTESIAN_POINT ( 'NONE',  ( 0.05938372350926800214, 32.37180007765648782, 2.628655560595669183 ) ) ;
#5104=CARTESIAN_POINT ( 'NONE',  ( -0.05938372350920063936, 38.87819992234354771, 3.680117784833935701 ) ) ;
#5110=CARTESIAN_POINT ( 'NONE',  ( -3.607379964056306676, 40.24680007765648071, 2.690724712371306282 ) ) ;
#5118=ORIENTED_EDGE ( 'NONE', *, *, #444, .F. ) ;
#5119=CARTESIAN_POINT ( 'NONE',  ( -1.027846397803541700, 17.49680007765647716, 3.346150245485522312 ) ) ;
#5123=CARTESIAN_POINT ( 'NONE',  ( 2.518350579753611207, 35.62819992234354771, -0.7558219633769606149 ) ) ;
#5125=CARTESIAN_POINT ( 'NONE',  ( -2.115076519116362519, 22.62180007765647360, 3.012182706137107147 ) ) ;
#5133=CARTESIAN_POINT ( 'NONE',  ( 4.481649420246366589, 26.62180007765648426, -1.518615910253458212 ) ) ;
#5143=CARTESIAN_POINT ( 'NONE',  ( -0.05938372350926768989, 33.62180007765647360, -2.628655560595669183 ) ) ;
#5145=CARTESIAN_POINT ( 'NONE',  ( 1.135272562821090458, 29.74680007765647716, 3.311245368580554072 ) ) ;
#5152=CARTESIAN_POINT ( 'NONE',  ( 2.798362969681366330, 26.49680007765648071, -2.102939460078824929 ) ) ;
#5166=CARTESIAN_POINT ( 'NONE',  ( -2.211161402132902243, 33.37180007765648071, -2.942372952327172886 ) ) ;
#5170=CARTESIAN_POINT ( 'NONE',  ( 3.673772985318163098, 33.00319992234354771, -2.599342558261029001 ) ) ;
#5172=CARTESIAN_POINT ( 'NONE',  ( 1.593127413382953383, 30.37819992234354061, -2.091722143975172532 ) ) ;
#5174=CARTESIAN_POINT ( 'NONE',  ( 1.336863392178479160, 26.24680007765647716, -4.297206761780677731 ) ) ;
#5179=CARTESIAN_POINT ( 'NONE',  ( -2.115076519116362519, 40.12180007765648071, 3.012182706137107147 ) ) ;
#5186=EDGE_CURVE ( 'NONE', #13000, #6995, #14926, .T. ) ;
#5194=CARTESIAN_POINT ( 'NONE',  ( 2.115076519116426024, 36.12819992234355482, 3.012182706137062294 ) ) ;
#5198=CARTESIAN_POINT ( 'NONE',  ( -1.989345975306426206, 32.74680007765648071, 1.515154207786343799 ) ) ;
#5199=SHAPE_REPRESENTATION ( 'Return Spring', ( #16940 ), #6566 ) ;
#5200=CARTESIAN_POINT ( 'NONE',  ( 1.336863392178569754, 26.25319992234354416, 4.297206761780648421 ) ) ;
#5205=CARTESIAN_POINT ( 'NONE',  ( -3.607379964056306676, 37.74680007765647360, 2.690724712371306282 ) ) ;
#5213=CARTESIAN_POINT ( 'NONE',  ( 2.864755990943265829, 19.49680007765648071, 2.011557305968487697 ) ) ;
#5216=CARTESIAN_POINT ( 'NONE',  ( 0.05938372350920109732, 15.12819992234354238, -3.680117784833935701 ) ) ;
#5219=CARTESIAN_POINT ( 'NONE',  ( 2.798362969681366330, 31.49680007765647716, -2.102939460078824929 ) ) ;
#5220=CARTESIAN_POINT ( 'NONE',  ( 2.115076519116426024, 21.12819992234353705, 3.012182706137062294 ) ) ;
#5227=CARTESIAN_POINT ( 'NONE',  ( -0.05938372350928957516, 23.62180007765647005, -4.731580009072201776 ) ) ;
#5229=CIRCLE ( 'NONE', #8192, 0.4999999999999992784 ) ;
#5234=CARTESIAN_POINT ( 'NONE',  ( 1.593127413382998903, 34.62180007765648071, 2.091722143975139669 ) ) ;
#5236=CARTESIAN_POINT ( 'NONE',  ( -2.798362969681365886, 37.74680007765647360, 2.102939460078824929 ) ) ;
#5239=CARTESIAN_POINT ( 'NONE',  ( -2.908635224650709894, 15.00000000000001066, -2.619577396687581050 ) ) ;
#5243=CARTESIAN_POINT ( 'NONE',  ( 3.481649420246369697, 21.62180007765647360, -1.193696214020541824 ) ) ;
#5258=CARTESIAN_POINT ( 'NONE',  ( -0.7188294034286043521, 17.49680007765647716, 2.395093729190366005 ) ) ;
#5264=CARTESIAN_POINT ( 'NONE',  ( -3.607379964056363075, 37.25319992234354061, -2.690724712371229899 ) ) ;
#5266=CARTESIAN_POINT ( 'NONE',  ( -2.055738996568281518, 24.25319992234354061, 1.423772053676066962 ) ) ;
#5269=CARTESIAN_POINT ( 'NONE',  ( 4.518350579753633411, 26.87180007765647716, 1.405661355842698468 ) ) ;
#5285=CARTESIAN_POINT ( 'NONE',  ( 2.864755990943222308, 33.00319992234354771, -2.011557305968548093 ) ) ;
#5286=CARTESIAN_POINT ( 'NONE',  ( -2.798362969681409851, 19.75319992234354416, -2.102939460078765421 ) ) ;
#5290=CARTESIAN_POINT ( 'NONE',  ( 2.518350579753628971, 31.87180007765648426, 0.7558219633769073242 ) ) ;
#5291=CARTESIAN_POINT ( 'NONE',  ( 0.05938372350919016857, 25.12819992234354416, -4.731580009072201776 ) ) ;
#5296=CARTESIAN_POINT ( 'NONE',  ( -3.673772985318219053, 35.74680007765646650, -2.599342558260952174 ) ) ;
#5307=CARTESIAN_POINT ( 'NONE',  ( -2.211161402132902243, 15.87180007765647716, -2.942372952327172886 ) ) ;
#5312=CARTESIAN_POINT ( 'NONE',  ( 0.8262555684460829442, 37.75319992234354771, -2.360188852285421302 ) ) ;
#5315=CARTESIAN_POINT ( 'NONE',  ( 2.864755990943265829, 31.99680007765647716, 2.011557305968487697 ) ) ;
#5317=CARTESIAN_POINT ( 'NONE',  ( -2.864755990943222308, 24.25319992234354416, 2.011557305968548093 ) ) ;
#5322=EDGE_CURVE ( 'NONE', #9517, #6875, #13982, .T. ) ;
#5324=CARTESIAN_POINT ( 'NONE',  ( -4.518350579753632523, 23.12180007765647005, -1.405661355842698468 ) ) ;
#5332=CARTESIAN_POINT ( 'NONE',  ( -1.989345975306426206, 37.74680007765647360, 1.515154207786343799 ) ) ;
#5334=CARTESIAN_POINT ( 'NONE',  ( -1.027846397803541700, 34.99680007765648071, 3.346150245485522312 ) ) ;
#5336=CARTESIAN_POINT ( 'NONE',  ( -3.313999109161785306, 15.00000000000000888, -2.150837222270006066 ) ) ;
#5339=CARTESIAN_POINT ( 'NONE',  ( 2.211161402132902243, 27.12180007765647360, 2.942372952327172442 ) ) ;
#5351=CARTESIAN_POINT ( 'NONE',  ( -2.798362969681365886, 37.74680007765647360, 2.102939460078824929 ) ) ;
#5355=APPLICATION_CONTEXT ( 'automotive_design' ) ;
#5358=CARTESIAN_POINT ( 'NONE',  ( -4.481649420246396787, 37.12819992234354061, -1.518615910253363399 ) ) ;
#5360=CARTESIAN_POINT ( 'NONE',  ( -0.8262555684460826111, 31.50319992234354416, 2.360188852285421302 ) ) ;
#5364=CARTESIAN_POINT ( 'NONE',  ( 0.05938372350929014415, 22.37180007765647716, 4.731580009072201776 ) ) ;
#5377=CARTESIAN_POINT ( 'NONE',  ( -2.864755990943265829, 15.74680007765647716, -2.011557305968488141 ) ) ;
#5380=CARTESIAN_POINT ( 'NONE',  ( 3.481649420246394122, 33.37819992234353350, 1.193696214020467439 ) ) ;
#5381=CARTESIAN_POINT ( 'NONE',  ( 2.115076519116425580, 16.12819992234354416, 3.012182706137062294 ) ) ;
#5383=CARTESIAN_POINT ( 'NONE',  ( -0.8262555684461330152, 33.49680007765648071, -2.360188852285403982 ) ) ;
#5384=CARTESIAN_POINT ( 'NONE',  ( -2.829195390882724315, 26.62819992234354416, 3.793023760679264722 ) ) ;
#5389=CARTESIAN_POINT ( 'NONE',  ( -1.135272562821090014, 23.49680007765647716, -3.311245368580554072 ) ) ;
#5397=CARTESIAN_POINT ( 'NONE',  ( 3.518350579753631191, 16.87180007765648071, 1.080741659609802285 ) ) ;
#5404=CARTESIAN_POINT ( 'NONE',  ( -1.593127413382952939, 39.12819992234354771, 2.091722143975172532 ) ) ;
#5406=CARTESIAN_POINT ( 'NONE',  ( -2.211161402132902243, 33.37180007765648071, -2.942372952327172886 ) ) ;
#5408=CARTESIAN_POINT ( 'NONE',  ( 1.027846397803612311, 26.25319992234354771, 3.346150245485499219 ) ) ;
#5421=CARTESIAN_POINT ( 'NONE',  ( 2.055738996568313048, 36.99680007765647360, 1.423772053676023441 ) ) ;
#5424=CARTESIAN_POINT ( 'NONE',  ( 2.798362969681366330, 33.99680007765648071, -2.102939460078824929 ) ) ;
#5431=CARTESIAN_POINT ( 'NONE',  ( -2.864755990943265829, 20.74680007765647716, -2.011557305968488141 ) ) ;
#5441=CARTESIAN_POINT ( 'NONE',  ( 1.989345975306426206, 16.49680007765648071, -1.515154207786343799 ) ) ;
#5445=CARTESIAN_POINT ( 'NONE',  ( -4.518350579753632523, 18.12180007765647716, -1.405661355842698468 ) ) ;
#5447=CARTESIAN_POINT ( 'NONE',  ( 1.593127413382953383, 27.87819992234355126, -2.091722143975172532 ) ) ;
#5450=CARTESIAN_POINT ( 'NONE',  ( 4.481649420246366589, 26.62180007765648426, -1.518615910253458212 ) ) ;
#5465=CARTESIAN_POINT ( 'NONE',  ( 3.481649420246370141, 16.62180007765647716, -1.193696214020541602 ) ) ;
#5468=CARTESIAN_POINT ( 'NONE',  ( 1.027846397803612311, 33.75319992234354771, 3.346150245485499219 ) ) ;
#5469=CARTESIAN_POINT ( 'NONE',  ( -2.864755990943222308, 16.75319992234354416, 2.011557305968548093 ) ) ;
#5471=CARTESIAN_POINT ( 'NONE',  ( -1.593127413382998459, 28.37180007765648426, -2.091722143975139669 ) ) ;
#5472=CARTESIAN_POINT ( 'NONE',  ( 1.336863392178569754, 28.75319992234354771, 4.297206761780648421 ) ) ;
#5473=UNCERTAINTY_MEASURE_WITH_UNIT (LENGTH_MEASURE( 1.000000000000000082E-05 ), #13339, 'distance_accuracy_value', 'NONE');
#5480=CARTESIAN_POINT ( 'NONE',  ( -3.481649420246369697, 22.87180007765647360, 1.193696214020542490 ) ) ;
#5493=CARTESIAN_POINT ( 'NONE',  ( -0.8262555684460826111, 39.00319992234355482, 2.360188852285421302 ) ) ;
#5495=CARTESIAN_POINT ( 'NONE',  ( 3.481649420246369697, 29.12180007765647005, -1.193696214020541824 ) ) ;
#5496=CARTESIAN_POINT ( 'NONE',  ( 3.500000000000000444, 25.75319992234354771, 0.05647727720529520379 ) ) ;
#5507=CARTESIAN_POINT ( 'NONE',  ( 2.481649420246391902, 15.87819992234354771, 0.8687765177875720335 ) ) ;
#5510=CARTESIAN_POINT ( 'NONE',  ( -3.481649420246370141, 35.37180007765648071, 1.193696214020542268 ) ) ;
#5516=CARTESIAN_POINT ( 'NONE',  ( 3.481649420246369697, 29.12180007765647005, -1.193696214020541824 ) ) ;
#5529=CARTESIAN_POINT ( 'NONE',  ( 1.497042530366477164, 16.37180007765648426, -2.161531897785062384 ) ) ;
#5532=CARTESIAN_POINT ( 'NONE',  ( 4.518350579753633411, 16.87180007765647716, 1.405661355842698468 ) ) ;
#5535=CARTESIAN_POINT ( 'NONE',  ( -2.500000000000001332, 39.50319992234355482, -0.05647727720530596601 ) ) ;
#5538=CARTESIAN_POINT ( 'NONE',  ( -0.05938372350928957516, 26.12180007765648426, -4.731580009072201776 ) ) ;
#5555=SURFACE_STYLE_FILL_AREA ( #4341 ) ;
#5556=CARTESIAN_POINT ( 'NONE',  ( -2.733110507866328476, 14.87819992234354238, -3.862833514489096398 ) ) ;
#5557=CARTESIAN_POINT ( 'NONE',  ( -3.500000000000000444, 17.00319992234354416, -0.05647727720529563400 ) ) ;
#5559=CARTESIAN_POINT ( 'NONE',  ( -1.989345975306426206, 35.24680007765648071, 1.515154207786343799 ) ) ;
#5561=CARTESIAN_POINT ( 'NONE',  ( -1.444289557195956863, 26.50319992234354771, 4.262301884875733471 ) ) ;
#5566=CARTESIAN_POINT ( 'NONE',  ( 2.798362969681366330, 21.49680007765647716, -2.102939460078824929 ) ) ;
#5575=CARTESIAN_POINT ( 'NONE',  ( 2.798362969681366330, 26.49680007765648071, -2.102939460078824929 ) ) ;
#5583=CARTESIAN_POINT ( 'NONE',  ( 2.864755990943222308, 15.50319992234354416, -2.011557305968548093 ) ) ;
#5586=CARTESIAN_POINT ( 'NONE',  ( 3.518350579753631191, 34.37180007765648071, 1.080741659609802285 ) ) ;
#5588=CARTESIAN_POINT ( 'NONE',  ( 2.864755990943222308, 25.50319992234354771, -2.011557305968548093 ) ) ;
#5604=CARTESIAN_POINT ( 'NONE',  ( 0.05938372350926800214, 34.87180007765648071, 2.628655560595669183 ) ) ;
#5606=CARTESIAN_POINT ( 'NONE',  ( -3.500000000000000444, 40.49680007765648071, 0.05647727720536853402 ) ) ;
#5610=CARTESIAN_POINT ( 'NONE',  ( -3.481649420246369697, 30.37180007765647005, 1.193696214020542490 ) ) ;
#5615=FACE_OUTER_BOUND ( 'NONE', #14074, .T. ) ;
#5623=CARTESIAN_POINT ( 'NONE',  ( 2.864755990943265829, 36.99680007765648071, 2.011557305968487697 ) ) ;
#5630=CARTESIAN_POINT ( 'NONE',  ( -0.05938372350921170689, 36.37819992234354771, 2.628655560595669183 ) ) ;
#5634=CARTESIAN_POINT ( 'NONE',  ( -4.481649420246366589, 32.87180007765647360, 1.518615910253458878 ) ) ;
#5647=CARTESIAN_POINT ( 'NONE',  ( 1.336863392178569754, 16.25319992234354416, 4.297206761780648421 ) ) ;
#5648=CARTESIAN_POINT ( 'NONE',  ( 2.211161402132839182, 17.87819992234354771, -2.942372952327217739 ) ) ;
#5651=CARTESIAN_POINT ( 'NONE',  ( -0.7188294034286043521, 39.99680007765647360, 2.395093729190366005 ) ) ;
#5652=CARTESIAN_POINT ( 'NONE',  ( 4.499999999999999112, 33.25319992234354771, 0.05647727720528474687 ) ) ;
#5657=CARTESIAN_POINT ( 'NONE',  ( 2.864755990943265829, 24.49680007765647716, 2.011557305968487697 ) ) ;
#5660=CARTESIAN_POINT ( 'NONE',  ( -3.673772985318219053, 25.74680007765648426, -2.599342558260952174 ) ) ;
#5666=CARTESIAN_POINT ( 'NONE',  ( 1.135272562821090458, 24.74680007765647716, 3.311245368580554072 ) ) ;
#5672=CARTESIAN_POINT ( 'NONE',  ( 2.798362969681409851, 21.00319992234354416, 2.102939460078764977 ) ) ;
#5674=CARTESIAN_POINT ( 'NONE',  ( 0.7188294034286049072, 16.24680007765648071, -2.395093729190366005 ) ) ;
#5675=CARTESIAN_POINT ( 'NONE',  ( 3.518350579753605434, 38.12819992234354061, -1.080741659609877114 ) ) ;
#5693=CARTESIAN_POINT ( 'NONE',  ( -2.481649420246391902, 22.12819992234354771, -0.8687765177875723666 ) ) ;
#5701=CARTESIAN_POINT ( 'NONE',  ( -3.481649420246369697, 32.87180007765645939, 1.193696214020542490 ) ) ;
#5716=CARTESIAN_POINT ( 'NONE',  ( 0.05938372350926800214, 22.37180007765647716, 2.628655560595669183 ) ) ;
#5720=CARTESIAN_POINT ( 'NONE',  ( 2.518350579753611207, 38.12819992234354771, -0.7558219633769606149 ) ) ;
#5723=CARTESIAN_POINT ( 'NONE',  ( 1.336863392178479160, 36.24680007765647360, -4.297206761780677731 ) ) ;
#5736=( BOUNDED_CURVE ( )  B_SPLINE_CURVE ( 2, ( #3894, #8247, #5377, #3796, #13908, #9543, #12231, #6581, #11026, #5465, #13718, #16800, #13532, #17919, #9453, #2429, #8150, #1123, #12416, #16707, #17419, #4687, #15730, #11821, #7368, #5799, #17517, #15826, #14339, #1735, #13028, #344, #11725, #3122, #10240, #245, #5981, #6071, #8756, #12845, #2938, #15917, #11634, #8573, #17328, #14430, #14246, #8851, #10335, #4591, #1549, #7187, #11443, #4504, #17135, #15406, #13210, #3218, #14531, #16014, #10147, #1828, #6173, #4411, #7465, #9719, #3306, #149, #5890, #12930, #13124, #11539, #8948, #433, #14629, #1931, #7555, #527, #17231, #10053, #3028, #8662, #1637, #7274, #14815, #3754, #3579, #2292, #9229, #801, #9044, #16111, #4962, #624, #9136, #6537, #13669, #10525, #989, #16197, #9403, #13311, #7743, #13487, #6361, #16384, #17612, #3488, #12189, #12003, #17876, #2113, #17792, #2205, #5145, #7921, #17698, #16473, #12096, #13401, #14720, #4779, #2018, #15081, #7646, #6633, #713, #10803, #10431, #7831, #3402, #5052, #6263, #10708, #2385, #10618, #12278, #6448, #11915, #4874, #16292, #8016, #14911, #3673, #9318, #14991, #13578, #895, #5424, #3850, #13861, #6982, #16846, #9676, #18240, #8292, #5334, #14130, #4029, #5510, #16939, #2477, #11156, #15173, #2567, #1442, #8198, #1169, #16755, #6809, #7072, #18333, #4124, #12459, #3940, #10985, #17967, #15358, #5236, #1350, #16664, #9496, #10891, #18154, #13766, #9591, #12643, #8462, #15269, #16570, #11072, #4212, #12367, #8107, #2657, #13950, #1263, #9772, #18061, #6895, #5606 ),
 .UNSPECIFIED., .F., .T. ) 
 B_SPLINE_CURVE_WITH_KNOTS ( ( 3, 2, 2, 2, 2, 2, 2, 2, 2, 2, 2, 2, 2, 2, 2, 2, 2, 2, 2, 2, 2, 2, 2, 2, 2, 2, 2, 2, 2, 2, 2, 2, 2, 2, 2, 2, 2, 2, 2, 2, 2, 2, 2, 2, 2, 2, 2, 2, 2, 2, 2, 2, 2, 2, 2, 2, 2, 2, 2, 2, 2, 2, 2, 2, 2, 2, 2, 2, 2, 2, 2, 2, 2, 2, 2, 2, 2, 2, 2, 2, 2, 2, 2, 2, 2, 2, 2, 2, 2, 2, 2, 2, 2, 2, 2, 2, 2, 2, 2, 2, 3 ),
 ( 0.000000000000000000, 0.01000000000000000021, 0.02000000000000000042, 0.02999999999999999889, 0.04000000000000000083, 0.05000000000000000278, 0.05999999999999999778, 0.07000000000000000666, 0.08000000000000000167, 0.08999999999999999667, 0.1000000000000000056, 0.1100000000000000006, 0.1199999999999999956, 0.1300000000000000044, 0.1400000000000000133, 0.1499999999999999944, 0.1600000000000000033, 0.1700000000000000122, 0.1799999999999999933, 0.1900000000000000022, 0.2000000000000000111, 0.2099999999999999922, 0.2200000000000000011, 0.2300000000000000100, 0.2399999999999999911, 0.2500000000000000000, 0.2600000000000000089, 0.2700000000000000178, 0.2800000000000000266, 0.2899999999999999800, 0.2999999999999999889, 0.3099999999999999978, 0.3200000000000000067, 0.3300000000000000155, 0.3400000000000000244, 0.3499999999999999778, 0.3599999999999999867, 0.3699999999999999956, 0.3800000000000000044, 0.3900000000000000133, 0.4000000000000000222, 0.4099999999999999756, 0.4199999999999999845, 0.4299999999999999933, 0.4400000000000000022, 0.4500000000000000111, 0.4600000000000000200, 0.4699999999999999734, 0.4799999999999999822, 0.4899999999999999911, 0.5000000000000000000, 0.5100000000000000089, 0.5200000000000000178, 0.5300000000000000266, 0.5400000000000000355, 0.5500000000000000444, 0.5600000000000000533, 0.5699999999999999512, 0.5799999999999999600, 0.5899999999999999689, 0.5999999999999999778, 0.6099999999999999867, 0.6199999999999999956, 0.6300000000000000044, 0.6400000000000000133, 0.6500000000000000222, 0.6600000000000000311, 0.6700000000000000400, 0.6800000000000000488, 0.6899999999999999467, 0.6999999999999999556, 0.7099999999999999645, 0.7199999999999999734, 0.7299999999999999822, 0.7399999999999999911, 0.7500000000000000000, 0.7600000000000000089, 0.7700000000000000178, 0.7800000000000000266, 0.7900000000000000355, 0.8000000000000000444, 0.8100000000000000533, 0.8199999999999999512, 0.8299999999999999600, 0.8399999999999999689, 0.8499999999999999778, 0.8599999999999999867, 0.8699999999999999956, 0.8800000000000000044, 0.8900000000000000133, 0.9000000000000000222, 0.9100000000000000311, 0.9200000000000000400, 0.9300000000000000488, 0.9399999999999999467, 0.9499999999999999556, 0.9599999999999999645, 0.9699999999999999734, 0.9799999999999999822, 0.9899999999999999911, 1.000000000000000000 ),
 .UNSPECIFIED. ) 
 CURVE ( )  GEOMETRIC_REPRESENTATION_ITEM ( )  RATIONAL_B_SPLINE_CURVE ( ( 1.000000000000000000, 0.9510565162951535312, 1.000000000000000000, 0.9510565162951535312, 1.000000000000000000, 0.9510565162951535312, 1.000000000000000000, 0.9510565162951535312, 1.000000000000000000, 0.9510565162951535312, 1.000000000000000000, 0.9510565162951535312, 1.000000000000000000, 0.9510565162951535312, 1.000000000000000000, 0.9510565162951535312, 1.000000000000000000, 0.9510565162951535312, 1.000000000000000000, 0.9510565162951535312, 1.000000000000000000, 0.9510565162951535312, 1.000000000000000000, 0.9510565162951535312, 1.000000000000000000, 0.9510565162951535312, 1.000000000000000000, 0.9510565162951535312, 1.000000000000000000, 0.9510565162951535312, 1.000000000000000000, 0.9510565162951535312, 1.000000000000000000, 0.9510565162951535312, 1.000000000000000000, 0.9510565162951535312, 1.000000000000000000, 0.9510565162951535312, 1.000000000000000000, 0.9510565162951535312, 1.000000000000000000, 0.9510565162951535312, 1.000000000000000000, 0.9510565162951535312, 1.000000000000000000, 0.9510565162951535312, 1.000000000000000000, 0.9510565162951535312, 1.000000000000000000, 0.9510565162951535312, 1.000000000000000000, 0.9510565162951535312, 1.000000000000000000, 0.9510565162951535312, 1.000000000000000000, 0.9510565162951535312, 1.000000000000000000, 0.9510565162951535312, 1.000000000000000000, 0.9510565162951535312, 1.000000000000000000, 0.9510565162951535312, 1.000000000000000000, 0.9510565162951535312, 1.000000000000000000, 0.9510565162951535312, 1.000000000000000000, 0.9510565162951535312, 1.000000000000000000, 0.9510565162951535312, 1.000000000000000000, 0.9510565162951535312, 1.000000000000000000, 0.9510565162951535312, 1.000000000000000000, 0.9510565162951535312, 1.000000000000000000, 0.9510565162951535312, 1.000000000000000000, 0.9510565162951535312, 1.000000000000000000, 0.9510565162951535312, 1.000000000000000000, 0.9510565162951535312, 1.000000000000000000, 0.9510565162951535312, 1.000000000000000000, 0.9510565162951535312, 1.000000000000000000, 0.9510565162951535312, 1.000000000000000000, 0.9510565162951535312, 1.000000000000000000, 0.9510565162951535312, 1.000000000000000000, 0.9510565162951535312, 1.000000000000000000, 0.9510565162951535312, 1.000000000000000000, 0.9510565162951535312, 1.000000000000000000, 0.9510565162951535312, 1.000000000000000000, 0.9510565162951535312, 1.000000000000000000, 0.9510565162951535312, 1.000000000000000000, 0.9510565162951535312, 1.000000000000000000, 0.9510565162951535312, 1.000000000000000000, 0.9510565162951535312, 1.000000000000000000, 0.9510565162951535312, 1.000000000000000000, 0.9510565162951535312, 1.000000000000000000, 0.9510565162951535312, 1.000000000000000000, 0.9510565162951535312, 1.000000000000000000, 0.9510565162951535312, 1.000000000000000000, 0.9510565162951535312, 1.000000000000000000, 0.9510565162951535312, 1.000000000000000000, 0.9510565162951535312, 1.000000000000000000, 0.9510565162951535312, 1.000000000000000000, 0.9510565162951535312, 1.000000000000000000, 0.9510565162951535312, 1.000000000000000000, 0.9510565162951535312, 1.000000000000000000, 0.9510565162951535312, 1.000000000000000000, 0.9510565162951535312, 1.000000000000000000, 0.9510565162951535312, 1.000000000000000000, 0.9510565162951535312, 1.000000000000000000, 0.9510565162951535312, 1.000000000000000000, 0.9510565162951535312, 1.000000000000000000, 0.9510565162951535312, 1.000000000000000000, 0.9510565162951535312, 1.000000000000000000, 0.9510565162951535312, 1.000000000000000000, 0.9510565162951535312, 1.000000000000000000, 0.9510565162951535312, 1.000000000000000000, 0.9510565162951535312, 1.000000000000000000, 0.9510565162951535312, 1.000000000000000000, 0.9510565162951535312, 1.000000000000000000, 0.9510565162951535312, 1.000000000000000000, 0.9510565162951535312, 1.000000000000000000, 0.9510565162951535312, 1.000000000000000000, 0.9510565162951535312, 1.000000000000000000, 0.9510565162951535312, 1.000000000000000000, 0.9510565162951535312, 1.000000000000000000, 0.9510565162951535312, 1.000000000000000000, 0.9510565162951535312, 1.000000000000000000, 0.9510565162951535312, 1.000000000000000000, 0.9510565162951535312, 1.000000000000000000, 0.9510565162951535312, 1.000000000000000000, 0.9510565162951535312, 1.000000000000000000, 0.9510565162951535312, 1.000000000000000000, 0.9510565162951535312, 1.000000000000000000, 0.9510565162951535312, 1.000000000000000000, 0.9510565162951535312, 1.000000000000000000, 0.9510565162951535312, 1.000000000000000000, 0.9510565162951535312, 1.000000000000000000 ) ) 
 REPRESENTATION_ITEM ( '' )  );
#5740=CARTESIAN_POINT ( 'NONE',  ( -0.05938372350918959958, 18.87819992234354416, 4.731580009072201776 ) ) ;
#5741=CARTESIAN_POINT ( 'NONE',  ( 1.027846397803612311, 31.25319992234354416, 3.346150245485499219 ) ) ;
#5743=CARTESIAN_POINT ( 'NONE',  ( -0.05938372350926768989, 36.12180007765648071, -2.628655560595669183 ) ) ;
#5744=CARTESIAN_POINT ( 'NONE',  ( -4.481649420246396787, 37.12819992234354061, -1.518615910253363399 ) ) ;
#5750=CARTESIAN_POINT ( 'NONE',  ( -2.211161402132902243, 20.87180007765647716, -2.942372952327172886 ) ) ;
#5755=CARTESIAN_POINT ( 'NONE',  ( 3.607379964056306676, 23.99680007765647716, -2.690724712371305838 ) ) ;
#5760=CARTESIAN_POINT ( 'NONE',  ( -2.864755990943265829, 23.24680007765647716, -2.011557305968488141 ) ) ;
#5764=CARTESIAN_POINT ( 'NONE',  ( 2.211161402132839626, 15.37819992234354771, -2.942372952327218183 ) ) ;
#5766=CARTESIAN_POINT ( 'NONE',  ( 1.135272562821090458, 37.24680007765648071, 3.311245368580554072 ) ) ;
#5767=CARTESIAN_POINT ( 'NONE',  ( -0.05938372350920063936, 36.37819992234355482, 3.680117784833935701 ) ) ;
#5778=CARTESIAN_POINT ( 'NONE',  ( -2.518350579753611207, 24.37819992234354416, 0.7558219633769609480 ) ) ;
#5780=CARTESIAN_POINT ( 'NONE',  ( 1.027846397803542144, 16.24680007765647716, -3.346150245485522312 ) ) ;
#5786=CARTESIAN_POINT ( 'NONE',  ( 2.211161402132902243, 29.62180007765648071, 2.942372952327172442 ) ) ;
#5797=CARTESIAN_POINT ( 'NONE',  ( -1.989345975306426206, 25.24680007765648071, 1.515154207786343799 ) ) ;
#5799=CARTESIAN_POINT ( 'NONE',  ( -0.05938372350927861865, 18.62180007765647716, -3.680117784833935701 ) ) ;
#5805=CARTESIAN_POINT ( 'NONE',  ( -2.518350579753611207, 34.37819992234354771, 0.7558219633769609480 ) ) ;
#5809=CARTESIAN_POINT ( 'NONE',  ( -4.499999999999999112, 35.49680007765647360, 0.05647727720537927543 ) ) ;
#5824=CARTESIAN_POINT ( 'NONE',  ( 1.336863392178569754, 21.25319992234354771, 4.297206761780648421 ) ) ;
#5825=CARTESIAN_POINT ( 'NONE',  ( -2.864755990943222308, 31.75319992234354416, 2.011557305968548093 ) ) ;
#5826=CARTESIAN_POINT ( 'NONE',  ( 1.989345975306426206, 38.99680007765648071, -1.515154207786343799 ) ) ;
#5828=CARTESIAN_POINT ( 'NONE',  ( -2.829195390882724315, 34.12819992234354771, 3.793023760679264722 ) ) ;
#5831=CARTESIAN_POINT ( 'NONE',  ( -3.500000000000000444, 40.49680007765648071, 0.05647727720536853402 ) ) ;
#5833=CARTESIAN_POINT ( 'NONE',  ( 1.135272562821090458, 32.24680007765648071, 3.311245368580554072 ) ) ;
#5836=CARTESIAN_POINT ( 'NONE',  ( 0.05938372350929014415, 34.87180007765647360, 4.731580009072201776 ) ) ;
#5840=CARTESIAN_POINT ( 'NONE',  ( 0.05938372350927906274, 19.87180007765648426, 3.680117784833935701 ) ) ;
#5848=CARTESIAN_POINT ( 'NONE',  ( 1.027846397803612311, 21.25319992234354416, 3.346150245485499219 ) ) ;
#5851=CARTESIAN_POINT ( 'NONE',  ( 2.798362969681366330, 38.99680007765647360, -2.102939460078824929 ) ) ;
#5853=CARTESIAN_POINT ( 'NONE',  ( 2.798362969681409851, 33.50319992234354771, 2.102939460078764977 ) ) ;
#5865=CARTESIAN_POINT ( 'NONE',  ( -1.048844091575818815, 15.00000000000000888, -3.317259973752782809 ) ) ;
#5868=CARTESIAN_POINT ( 'NONE',  ( 1.497042530366522461, 18.62819992234354771, 2.161531897785029965 ) ) ;
#5870=CARTESIAN_POINT ( 'NONE',  ( -0.05938372350928957516, 18.62180007765647716, -4.731580009072201776 ) ) ;
#5871=MECHANICAL_DESIGN_GEOMETRIC_PRESENTATION_REPRESENTATION('',(#12384),#10906);
#5878=CARTESIAN_POINT ( 'NONE',  ( 2.864755990943265829, 29.49680007765647716, 2.011557305968487697 ) ) ;
#5888=CARTESIAN_POINT ( 'NONE',  ( 1.989345975306426206, 23.99680007765648071, -1.515154207786343799 ) ) ;
#5890=CARTESIAN_POINT ( 'NONE',  ( 2.798362969681366330, 23.99680007765647716, -2.102939460078824929 ) ) ;
#5894=CARTESIAN_POINT ( 'NONE',  ( 1.989345975306457071, 36.00319992234354771, 1.515154207786300500 ) ) ;
#5898=CARTESIAN_POINT ( 'NONE',  ( -3.673772985318219053, 33.24680007765647360, -2.599342558260952174 ) ) ;
#5918=CARTESIAN_POINT ( 'NONE',  ( -0.05938372350918959958, 21.37819992234354416, 4.731580009072201776 ) ) ;
#5919=CARTESIAN_POINT ( 'NONE',  ( -2.798362969681409851, 27.25319992234354771, -2.102939460078765421 ) ) ;
#5920=CARTESIAN_POINT ( 'NONE',  ( 2.055738996568281518, 15.50319992234354949, -1.423772053676066518 ) ) ;
#5922=CARTESIAN_POINT ( 'NONE',  ( 4.499999999999999112, 35.75319992234354061, 0.05647727720528474687 ) ) ;
#5928=CARTESIAN_POINT ( 'NONE',  ( 2.864755990943265829, 29.49680007765647716, 2.011557305968487697 ) ) ;
#5931=CARTESIAN_POINT ( 'NONE',  ( 2.829195390882805583, 29.62180007765647005, 3.793023760679204770 ) ) ;
#5935=CARTESIAN_POINT ( 'NONE',  ( 2.211161402132902243, 24.62180007765647716, 2.942372952327172442 ) ) ;
#5940=CARTESIAN_POINT ( 'NONE',  ( 1.135272562821020070, 20.25319992234354416, -3.311245368580577164 ) ) ;
#5943=CARTESIAN_POINT ( 'NONE',  ( -2.864755990943265829, 38.24680007765647360, -2.011557305968488141 ) ) ;
#5945=CARTESIAN_POINT ( 'NONE',  ( -1.135272562821019626, 36.50319992234354061, 3.311245368580577164 ) ) ;
#5957=CARTESIAN_POINT ( 'NONE',  ( -1.497042530366522461, 17.37819992234354416, -2.161531897785030409 ) ) ;
#5960=CARTESIAN_POINT ( 'NONE',  ( -2.733110507866247652, 17.62180007765648071, 3.862833514489154574 ) ) ;
#5964=CARTESIAN_POINT ( 'NONE',  ( -0.05938372350927861171, 38.62180007765648071, -3.680117784833935701 ) ) ;
#5979=CARTESIAN_POINT ( 'NONE',  ( -2.055738996568313048, 20.74680007765648071, -1.423772053676023441 ) ) ;
#5981=CARTESIAN_POINT ( 'NONE',  ( -1.027846397803541700, 19.99680007765648071, 3.346150245485522312 ) ) ;
#5986=CARTESIAN_POINT ( 'NONE',  ( -3.518350579753605434, 19.37819992234354416, 1.080741659609877781 ) ) ;
#5989=CARTESIAN_POINT ( 'NONE',  ( -4.481649420246366589, 37.87180007765647360, 1.518615910253458878 ) ) ;
#6007=CARTESIAN_POINT ( 'NONE',  ( -4.481649420246396787, 24.62819992234354416, -1.518615910253363399 ) ) ;
#6008=CARTESIAN_POINT ( 'NONE',  ( -3.500000000000000444, 24.50319992234354416, -0.05647727720529563400 ) ) ;
#6009=CARTESIAN_POINT ( 'NONE',  ( 2.481649420246391902, 20.87819992234355126, 0.8687765177875720335 ) ) ;
#6013=CARTESIAN_POINT ( 'NONE',  ( -3.673772985318163098, 31.75319992234354771, 2.599342558261029001 ) ) ;
#6019=CARTESIAN_POINT ( 'NONE',  ( 1.027846397803542144, 26.24680007765648071, -3.346150245485522312 ) ) ;
#6022=CARTESIAN_POINT ( 'NONE',  ( 2.733110507866247652, 33.87180007765647360, -3.862833514489153686 ) ) ;
#6026=CARTESIAN_POINT ( 'NONE',  ( -0.05938372350927861171, 31.12180007765647005, -3.680117784833935701 ) ) ;
#6031=CARTESIAN_POINT ( 'NONE',  ( -2.115076519116425580, 27.37819992234354771, -3.012182706137062738 ) ) ;
#6034=CARTESIAN_POINT ( 'NONE',  ( 3.500000000000000444, 36.74680007765648071, -0.05647727720536935281 ) ) ;
#6037=CARTESIAN_POINT ( 'NONE',  ( -3.500000000000000444, 34.50319992234354771, -0.05647727720529563400 ) ) ;
#6053=CARTESIAN_POINT ( 'NONE',  ( -2.500000000000001332, 17.00319992234354416, -0.05647727720530596601 ) ) ;
#6055=CARTESIAN_POINT ( 'NONE',  ( 2.864755990943265829, 16.99680007765647716, 2.011557305968487697 ) ) ;
#6059=CARTESIAN_POINT ( 'NONE',  ( 2.211161402132902243, 37.12180007765645939, 2.942372952327172442 ) ) ;
#6069=CARTESIAN_POINT ( 'NONE',  ( -0.05938372350926768989, 21.12180007765648426, -2.628655560595669183 ) ) ;
#6071=CARTESIAN_POINT ( 'NONE',  ( -2.115076519116362519, 20.12180007765647716, 3.012182706137108035 ) ) ;
#6076=CARTESIAN_POINT ( 'NONE',  ( 0.05938372350920109732, 22.62819992234354416, -3.680117784833935701 ) ) ;
#6081=CARTESIAN_POINT ( 'NONE',  ( -2.211161402132902243, 18.37180007765647005, -2.942372952327172886 ) ) ;
#6101=CARTESIAN_POINT ( 'NONE',  ( -1.336863392178569088, 22.50319992234354416, -4.297206761780648421 ) ) ;
#6102=CARTESIAN_POINT ( 'NONE',  ( 1.135272562821020070, 25.25319992234354416, -3.311245368580577164 ) ) ;
#6104=CARTESIAN_POINT ( 'NONE',  ( 2.481649420246391902, 18.37819992234354416, 0.8687765177875720335 ) ) ;
#6106=CARTESIAN_POINT ( 'NONE',  ( -4.518350579753632523, 18.12180007765647716, -1.405661355842698468 ) ) ;
#6111=CARTESIAN_POINT ( 'NONE',  ( 3.500000000000000444, 26.74680007765648071, -0.05647727720536935281 ) ) ;
#6116=CARTESIAN_POINT ( 'NONE',  ( -3.673772985318219053, 28.24680007765647360, -2.599342558260952174 ) ) ;
#6119=CARTESIAN_POINT ( 'NONE',  ( -3.518350579753630747, 28.12180007765647360, -1.080741659609802729 ) ) ;
#6125=CARTESIAN_POINT ( 'NONE',  ( 2.211161402132839626, 30.37819992234354416, -2.942372952327218183 ) ) ;
#6128=CARTESIAN_POINT ( 'NONE',  ( -1.497042530366477164, 20.12180007765648071, 2.161531897785062384 ) ) ;
#6129=CARTESIAN_POINT ( 'NONE',  ( 1.444289557195957086, 17.75319992234354061, -4.262301884875733471 ) ) ;
#6149=CARTESIAN_POINT ( 'NONE',  ( 0.8262555684460829442, 30.25319992234354771, -2.360188852285421302 ) ) ;
#6151=CARTESIAN_POINT ( 'NONE',  ( -2.864755990943265829, 20.74680007765647716, -2.011557305968488141 ) ) ;
#6156=CARTESIAN_POINT ( 'NONE',  ( 3.481649420246369697, 36.62180007765648071, -1.193696214020541824 ) ) ;
#6170=CARTESIAN_POINT ( 'NONE',  ( 2.500000000000001332, 34.24680007765648071, -0.05647727720535888202 ) ) ;
#6171=CIRCLE ( 'NONE', #15954, 0.4999999999999992784 ) ;
#6173=CARTESIAN_POINT ( 'NONE',  ( -2.864755990943265829, 23.24680007765647716, -2.011557305968488141 ) ) ;
#6178=CARTESIAN_POINT ( 'NONE',  ( -1.027846397803611866, 15.00319992234354594, -3.346150245485499219 ) ) ;
#6181=CARTESIAN_POINT ( 'NONE',  ( 3.481649420246369697, 19.12180007765648071, -1.193696214020541824 ) ) ;
#6200=CARTESIAN_POINT ( 'NONE',  ( -0.05938372350918959958, 23.87819992234354416, 4.731580009072201776 ) ) ;
#6201=CARTESIAN_POINT ( 'NONE',  ( 3.500000000000000444, 38.25319992234354061, 0.05647727720529520379 ) ) ;
#6203=CARTESIAN_POINT ( 'NONE',  ( 0.05938372350921204690, 20.12819992234354771, -2.628655560595669183 ) ) ;
#6205=CARTESIAN_POINT ( 'NONE',  ( -2.829195390882805139, 18.37180007765647360, -3.793023760679206102 ) ) ;
#6210=CARTESIAN_POINT ( 'NONE',  ( 3.500000000000000444, 31.74680007765647716, -0.05647727720536935281 ) ) ;
#6223=CARTESIAN_POINT ( 'NONE',  ( -1.135272562821019626, 26.50319992234354771, 3.311245368580577164 ) ) ;
#6226=CARTESIAN_POINT ( 'NONE',  ( 1.593127413382998903, 24.62180007765647716, 2.091722143975139669 ) ) ;
#6228=CARTESIAN_POINT ( 'NONE',  ( 0.05938372350919016857, 17.62819992234354416, -4.731580009072201776 ) ) ;
#6242=CARTESIAN_POINT ( 'NONE',  ( 0.7188294034286553114, 31.25319992234354416, 2.395093729190349130 ) ) ;
#6245=CARTESIAN_POINT ( 'NONE',  ( 3.518350579753631191, 19.37180007765648071, 1.080741659609802285 ) ) ;
#6252=FACE_OUTER_BOUND ( 'NONE', #13100, .T. ) ;
#6261=CARTESIAN_POINT ( 'NONE',  ( 0.7188294034286049072, 28.74680007765648426, -2.395093729190366005 ) ) ;
#6263=CARTESIAN_POINT ( 'NONE',  ( 2.864755990943265829, 31.99680007765647716, 2.011557305968487697 ) ) ;
#6267=CARTESIAN_POINT ( 'NONE',  ( 2.798362969681409851, 21.00319992234354416, 2.102939460078764977 ) ) ;
#6271=CARTESIAN_POINT ( 'NONE',  ( 2.211161402132902243, 17.12180007765648071, 2.942372952327172442 ) ) ;
#6293=CARTESIAN_POINT ( 'NONE',  ( -1.444289557195956863, 24.00319992234354416, 4.262301884875733471 ) ) ;
#6295=CARTESIAN_POINT ( 'NONE',  ( 2.211161402132839182, 32.87819992234354771, -2.942372952327217739 ) ) ;
#6296=CARTESIAN_POINT ( 'NONE',  ( -1.593127413382952939, 16.62819992234354061, 2.091722143975172532 ) ) ;
#6298=CARTESIAN_POINT ( 'NONE',  ( 1.336863392178479160, 18.74680007765647005, -4.297206761780677731 ) ) ;
#6305=CARTESIAN_POINT ( 'NONE',  ( 2.864755990943265829, 36.99680007765648071, 2.011557305968487697 ) ) ;
#6319=CARTESIAN_POINT ( 'NONE',  ( -3.518350579753605434, 24.37819992234353705, 1.080741659609877781 ) ) ;
#6322=CARTESIAN_POINT ( 'NONE',  ( -0.05938372350926768989, 23.62180007765648071, -2.628655560595669183 ) ) ;
#6324=CARTESIAN_POINT ( 'NONE',  ( 2.829195390882724759, 20.37819992234354416, -3.793023760679264278 ) ) ;
#6330=CARTESIAN_POINT ( 'NONE',  ( -4.518350579753632523, 35.62180007765647360, -1.405661355842698468 ) ) ;
#6341=CARTESIAN_POINT ( 'NONE',  ( 2.518350579753611207, 30.62819992234355126, -0.7558219633769606149 ) ) ;
#6344=CARTESIAN_POINT ( 'NONE',  ( -3.500000000000000444, 20.49680007765647716, 0.05647727720536892260 ) ) ;
#6359=CARTESIAN_POINT ( 'NONE',  ( 2.500000000000001332, 31.74680007765648782, -0.05647727720535888202 ) ) ;
#6361=CARTESIAN_POINT ( 'NONE',  ( -1.135272562821090014, 28.49680007765648071, -3.311245368580554072 ) ) ;
#6368=CARTESIAN_POINT ( 'NONE',  ( 1.027846397803542144, 16.24680007765647716, -3.346150245485522312 ) ) ;
#6387=CARTESIAN_POINT ( 'NONE',  ( -2.733110507866328476, 27.37819992234355126, -3.862833514489096398 ) ) ;
#6388=CARTESIAN_POINT ( 'NONE',  ( -3.481649420246394566, 37.12819992234354061, -1.193696214020467883 ) ) ;
#6389=CARTESIAN_POINT ( 'NONE',  ( 1.593127413382953383, 20.37819992234354771, -2.091722143975172532 ) ) ;
#6392=CARTESIAN_POINT ( 'NONE',  ( 4.499999999999999112, 38.25319992234354061, 0.05647727720528474687 ) ) ;
#6396=CARTESIAN_POINT ( 'NONE',  ( 2.211161402132902243, 37.12180007765645939, 2.942372952327172442 ) ) ;
#6408=CARTESIAN_POINT ( 'NONE',  ( 0.05938372350920109732, 27.62819992234353705, -3.680117784833935701 ) ) ;
#6411=CARTESIAN_POINT ( 'NONE',  ( -2.055738996568313048, 25.74680007765648426, -1.423772053676023441 ) ) ;
#6412=CARTESIAN_POINT ( 'NONE',  ( -4.499999999999999112, 19.50319992234354416, -0.05647727720528529505 ) ) ;
#6417=CARTESIAN_POINT ( 'NONE',  ( 3.607379964056306676, 36.49680007765646650, -2.690724712371305838 ) ) ;
#6427=CARTESIAN_POINT ( 'NONE',  ( -0.7188294034286550893, 25.00319992234354771, -2.395093729190349130 ) ) ;
#6428=DIRECTION ( 'NONE',  ( 1.000000000000000000, 0.000000000000000000, 0.000000000000000000 ) ) ;
#6431=CARTESIAN_POINT ( 'NONE',  ( 2.798362969681366330, 21.49680007765647716, -2.102939460078824929 ) ) ;
#6444=LINE ( 'NONE', #17694, #15383 ) ;
#6445=CARTESIAN_POINT ( 'NONE',  ( -1.593127413382998459, 30.87180007765647716, -2.091722143975139669 ) ) ;
#6448=CARTESIAN_POINT ( 'NONE',  ( -2.115076519116362519, 32.62180007765647360, 3.012182706137108035 ) ) ;
#6455=CARTESIAN_POINT ( 'NONE',  ( 3.500000000000000444, 21.74680007765647716, -0.05647727720536935281 ) ) ;
#6467=CARTESIAN_POINT ( 'NONE',  ( 3.518350579753631191, 34.37180007765648071, 1.080741659609802285 ) ) ;
#6470=CARTESIAN_POINT ( 'NONE',  ( -1.336863392178569088, 35.00319992234354771, -4.297206761780648421 ) ) ;
#6471=CARTESIAN_POINT ( 'NONE',  ( 3.518350579753606322, 33.12819992234354771, -1.080741659609876892 ) ) ;
#6472=CARTESIAN_POINT ( 'NONE',  ( 2.518350579753611207, 25.62819992234354416, -0.7558219633769606149 ) ) ;
#6474=CARTESIAN_POINT ( 'NONE',  ( 2.733110507866247652, 21.37180007765647360, -3.862833514489153686 ) ) ;
#6481=CARTESIAN_POINT ( 'NONE',  ( 0.05938372350927906274, 37.37180007765645939, 3.680117784833935701 ) ) ;
#6497=CARTESIAN_POINT ( 'NONE',  ( 0.05938372350920109732, 37.62819992234352640, -3.680117784833935701 ) ) ;
#6501=CARTESIAN_POINT ( 'NONE',  ( -1.593127413382998459, 18.37180007765648071, -2.091722143975139669 ) ) ;
#6502=CARTESIAN_POINT ( 'NONE',  ( 1.336863392178569754, 18.75319992234354416, 4.297206761780648421 ) ) ;
#6508=CARTESIAN_POINT ( 'NONE',  ( -1.444289557196047014, 38.49680007765647360, -4.262301884875704161 ) ) ;
#6519=CARTESIAN_POINT ( 'NONE',  ( 2.055738996568281518, 28.00319992234354771, -1.423772053676066518 ) ) ;
#6521=CARTESIAN_POINT ( 'NONE',  ( 3.500000000000000444, 21.74680007765647716, -0.05647727720536935281 ) ) ;
#6528=CARTESIAN_POINT ( 'NONE',  ( 4.499999999999999112, 24.24680007765647716, -0.05647727720537982360 ) ) ;
#6535=CARTESIAN_POINT ( 'NONE',  ( 1.989345975306426206, 31.49680007765648071, -1.515154207786343799 ) ) ;
#6537=CARTESIAN_POINT ( 'NONE',  ( 0.05938372350927906967, 27.37180007765647716, 3.680117784833935701 ) ) ;
#6543=CARTESIAN_POINT ( 'NONE',  ( -1.135272562821090014, 25.99680007765648071, -3.311245368580554072 ) ) ;
#6558=CARTESIAN_POINT ( 'NONE',  ( -2.798362969681365886, 30.24680007765648071, 2.102939460078824929 ) ) ;
#6562=CARTESIAN_POINT ( 'NONE',  ( -4.518350579753602325, 31.87819992234354416, 1.405661355842794391 ) ) ;
#6564=CARTESIAN_POINT ( 'NONE',  ( -1.497042530366522461, 29.87819992234354416, -2.161531897785030409 ) ) ;
#6566=( GEOMETRIC_REPRESENTATION_CONTEXT ( 3 ) GLOBAL_UNCERTAINTY_ASSIGNED_CONTEXT ( ( #9731 ) ) GLOBAL_UNIT_ASSIGNED_CONTEXT ( ( #7022, #2366, #8334 ) ) REPRESENTATION_CONTEXT ( 'NONE', 'WORKASPACE' ) );
#6567=CARTESIAN_POINT ( 'NONE',  ( 2.733110507866247652, 28.87180007765647716, -3.862833514489153686 ) ) ;
#6571=CARTESIAN_POINT ( 'NONE',  ( 3.500000000000000444, 39.24680007765647360, -0.05647727720536935281 ) ) ;
#6581=CARTESIAN_POINT ( 'NONE',  ( 2.115076519116362963, 16.37180007765647716, -3.012182706137107591 ) ) ;
#6585=CARTESIAN_POINT ( 'NONE',  ( -2.115076519116425580, 32.37819992234354771, -3.012182706137062738 ) ) ;
#6586=CARTESIAN_POINT ( 'NONE',  ( 2.864755990943222308, 15.50319992234354416, -2.011557305968548093 ) ) ;
#6588=CARTESIAN_POINT ( 'NONE',  ( -0.05938372350926768989, 31.12180007765648426, -2.628655560595669183 ) ) ;
#6591=CARTESIAN_POINT ( 'NONE',  ( -1.336863392178569088, 22.50319992234354416, -4.297206761780648421 ) ) ;
#6597=CARTESIAN_POINT ( 'NONE',  ( 4.499999999999999112, 36.74680007765647360, -0.05647727720537982360 ) ) ;
#6614=CARTESIAN_POINT ( 'NONE',  ( -2.798362969681409851, 14.75319992234354594, -2.102939460078765421 ) ) ;
#6617=CARTESIAN_POINT ( 'NONE',  ( 2.864755990943265829, 29.49680007765647716, 2.011557305968487697 ) ) ;
#6618=CARTESIAN_POINT ( 'NONE',  ( -2.798362969681409851, 19.75319992234354416, -2.102939460078765421 ) ) ;
#6624=CARTESIAN_POINT ( 'NONE',  ( -1.444289557196047014, 23.49680007765647716, -4.262301884875704161 ) ) ;
#6631=CARTESIAN_POINT ( 'NONE',  ( -2.500000000000001332, 14.50319992234354771, -0.05647727720530596601 ) ) ;
#6633=CARTESIAN_POINT ( 'NONE',  ( -0.05938372350927861865, 31.12180007765647360, -3.680117784833935701 ) ) ;
#6635=CARTESIAN_POINT ( 'NONE',  ( -3.912726941231881472, 15.00000000000000178, -0.8267756552389129432 ) ) ;
#6639=CARTESIAN_POINT ( 'NONE',  ( -2.115076519116362519, 22.62180007765647360, 3.012182706137107147 ) ) ;
#6648=CARTESIAN_POINT ( 'NONE',  ( -3.500000000000000444, 27.99680007765648071, 0.05647727720536892260 ) ) ;
#6654=CARTESIAN_POINT ( 'NONE',  ( 1.444289557195957086, 32.75319992234354061, -4.262301884875733471 ) ) ;
#6656=CARTESIAN_POINT ( 'NONE',  ( -2.481649420246391902, 27.12819992234355126, -0.8687765177875723666 ) ) ;
#6659=CARTESIAN_POINT ( 'NONE',  ( -0.05938372350928957516, 23.62180007765647005, -4.731580009072201776 ) ) ;
#6663=CARTESIAN_POINT ( 'NONE',  ( -1.027846397803541700, 39.99680007765648071, 3.346150245485522312 ) ) ;
#6673=CARTESIAN_POINT ( 'NONE',  ( -1.135272562821019626, 31.50319992234354416, 3.311245368580577164 ) ) ;
#6674=CARTESIAN_POINT ( 'NONE',  ( 3.518350579753606322, 23.12819992234354416, -1.080741659609876892 ) ) ;
#6677=CARTESIAN_POINT ( 'NONE',  ( 0.7188294034286049072, 26.24680007765647716, -2.395093729190366005 ) ) ;
#6678=CARTESIAN_POINT ( 'NONE',  ( 3.607379964056363075, 23.50319992234354416, 2.690724712371229010 ) ) ;
#6682=CARTESIAN_POINT ( 'NONE',  ( -0.05938372350928957516, 36.12180007765646650, -4.731580009072201776 ) ) ;
#6694=CARTESIAN_POINT ( 'NONE',  ( 0.7188294034286553114, 33.75319992234354771, 2.395093729190349130 ) ) ;
#6696=CARTESIAN_POINT ( 'NONE',  ( -1.027846397803541700, 29.99680007765648071, 3.346150245485522312 ) ) ;
#6697=CARTESIAN_POINT ( 'NONE',  ( 3.500000000000000444, 23.25319992234354416, 0.05647727720529520379 ) ) ;
#6705=CARTESIAN_POINT ( 'NONE',  ( 0.05938372350929014415, 22.37180007765647716, 4.731580009072201776 ) ) ;
#6714=CARTESIAN_POINT ( 'NONE',  ( 1.593127413382998903, 37.12180007765648071, 2.091722143975139669 ) ) ;
#6722=CARTESIAN_POINT ( 'NONE',  ( 3.518350579753631191, 21.87180007765647360, 1.080741659609802285 ) ) ;
#6725=PRODUCT_DEFINITION ( 'UNKNOWN', '', #3619, #936 ) ;
#6736=CARTESIAN_POINT ( 'NONE',  ( -2.518350579753628526, 18.12180007765648071, -0.7558219633769075463 ) ) ;
#6740=CARTESIAN_POINT ( 'NONE',  ( -4.499999999999999112, 32.00319992234354061, -0.05647727720528529505 ) ) ;
#6743=CARTESIAN_POINT ( 'NONE',  ( -2.055738996568281518, 26.75319992234354771, 1.423772053676066962 ) ) ;
#6746=CARTESIAN_POINT ( 'NONE',  ( -4.481649420246366589, 25.37180007765648426, 1.518615910253458878 ) ) ;
#6761=CARTESIAN_POINT ( 'NONE',  ( -1.027846397803611866, 35.00319992234354771, -3.346150245485499219 ) ) ;
#6762=CARTESIAN_POINT ( 'NONE',  ( 2.864755990943222308, 18.00319992234354771, -2.011557305968548093 ) ) ;
#6765=CARTESIAN_POINT ( 'NONE',  ( -1.593127413382998459, 33.37180007765648071, -2.091722143975139669 ) ) ;
#6766=CARTESIAN_POINT ( 'NONE',  ( 2.733110507866328920, 28.62819992234354416, 3.862833514489095510 ) ) ;
#6771=CARTESIAN_POINT ( 'NONE',  ( -2.798362969681365886, 20.24680007765647716, 2.102939460078824929 ) ) ;
#6782=CARTESIAN_POINT ( 'NONE',  ( -3.518350579753630747, 18.12180007765648071, -1.080741659609802729 ) ) ;
#6788=CARTESIAN_POINT ( 'NONE',  ( 2.481649420246391902, 35.87819992234354771, 0.8687765177875720335 ) ) ;
#6791=CARTESIAN_POINT ( 'NONE',  ( 3.500000000000000444, 29.24680007765647716, -0.05647727720536935281 ) ) ;
#6794=CARTESIAN_POINT ( 'NONE',  ( -2.798362969681409851, 29.75319992234354416, -2.102939460078765421 ) ) ;
#6807=CARTESIAN_POINT ( 'NONE',  ( -1.989345975306457071, 14.75319992234354771, -1.515154207786300944 ) ) ;
#6809=CARTESIAN_POINT ( 'NONE',  ( 3.481649420246370141, 36.62180007765648071, -1.193696214020541602 ) ) ;
#6816=CARTESIAN_POINT ( 'NONE',  ( -2.211161402132902243, 25.87180007765647360, -2.942372952327172886 ) ) ;
#6828=CARTESIAN_POINT ( 'NONE',  ( 3.518350579753631191, 36.87180007765645939, 1.080741659609802285 ) ) ;
#6832=CARTESIAN_POINT ( 'NONE',  ( 4.499999999999999112, 33.25319992234354771, 0.05647727720528474687 ) ) ;
#6835=CARTESIAN_POINT ( 'NONE',  ( -2.500000000000001332, 27.00319992234355126, -0.05647727720530596601 ) ) ;
#6838=CARTESIAN_POINT ( 'NONE',  ( 2.829195390882805583, 24.62180007765647716, 3.793023760679204770 ) ) ;
#6855=CARTESIAN_POINT ( 'NONE',  ( -3.481649420246394122, 32.12819992234353350, -1.193696214020467883 ) ) ;
#6856=CARTESIAN_POINT ( 'NONE',  ( -3.481649420246394566, 22.12819992234354061, -1.193696214020467883 ) ) ;
#6858=CARTESIAN_POINT ( 'NONE',  ( 1.497042530366477164, 26.37180007765647716, -2.161531897785062384 ) ) ;
#6859=CARTESIAN_POINT ( 'NONE',  ( -4.518350579753602325, 24.37819992234354416, 1.405661355842794391 ) ) ;
#6864=CARTESIAN_POINT ( 'NONE',  ( -1.027846397803541700, 19.99680007765648071, 3.346150245485522312 ) ) ;
#6875=VERTEX_POINT ( 'NONE', #7035 ) ;
#6877=CARTESIAN_POINT ( 'NONE',  ( -1.989345975306457071, 37.25319992234354061, -1.515154207786300944 ) ) ;
#6879=CARTESIAN_POINT ( 'NONE',  ( 1.135272562821090458, 34.74680007765648071, 3.311245368580554072 ) ) ;
#6881=CARTESIAN_POINT ( 'NONE',  ( -1.135272562821019626, 29.00319992234354416, 3.311245368580577164 ) ) ;
#6893=CARTESIAN_POINT ( 'NONE',  ( 2.481649420246374138, 36.62180007765647360, -0.8687765177876252132 ) ) ;
#6895=CARTESIAN_POINT ( 'NONE',  ( -3.481649420246370141, 40.37180007765648071, 1.193696214020542268 ) ) ;
#6900=CARTESIAN_POINT ( 'NONE',  ( -1.055605843668875110, 15.00000000000000888, -3.337496964141338562 ) ) ;
#6904=CARTESIAN_POINT ( 'NONE',  ( -2.798362969681365886, 32.74680007765648071, 2.102939460078824929 ) ) ;
#6915=CARTESIAN_POINT ( 'NONE',  ( 2.211161402132902243, 37.12180007765645939, 2.942372952327172442 ) ) ;
#6919=CARTESIAN_POINT ( 'NONE',  ( -1.444289557195956863, 39.00319992234354061, 4.262301884875733471 ) ) ;
#6921=CARTESIAN_POINT ( 'NONE',  ( -1.989345975306457071, 34.75319992234354771, -1.515154207786300944 ) ) ;
#6925=CARTESIAN_POINT ( 'NONE',  ( -4.518350579753632523, 23.12180007765647005, -1.405661355842698468 ) ) ;
#6942=CARTESIAN_POINT ( 'NONE',  ( 3.673772985318163098, 15.50319992234354416, -2.599342558261029001 ) ) ;
#6943=CARTESIAN_POINT ( 'NONE',  ( 2.864755990943222308, 23.00319992234354416, -2.011557305968548093 ) ) ;
#6945=CARTESIAN_POINT ( 'NONE',  ( -1.989345975306426206, 30.24680007765648426, 1.515154207786343799 ) ) ;
#6946=CARTESIAN_POINT ( 'NONE',  ( 4.481649420246397675, 25.87819992234355126, 1.518615910253363177 ) ) ;
#6951=CARTESIAN_POINT ( 'NONE',  ( 2.798362969681366330, 23.99680007765647716, -2.102939460078824929 ) ) ;
#6959=CARTESIAN_POINT ( 'NONE',  ( -3.500000000000000444, 20.49680007765647716, 0.05647727720536892260 ) ) ;
#6965=CARTESIAN_POINT ( 'NONE',  ( -1.593127413382952939, 34.12819992234354771, 2.091722143975172532 ) ) ;
#6967=CARTESIAN_POINT ( 'NONE',  ( -3.500000000000000444, 27.99680007765648071, 0.05647727720536892260 ) ) ;
#6968=CARTESIAN_POINT ( 'NONE',  ( 3.500000000000000444, 30.75319992234354416, 0.05647727720529520379 ) ) ;
#6976=CARTESIAN_POINT ( 'NONE',  ( -2.937035047792128761, 15.00000000000010125, -0.6671309589350113978 ) ) ;
#6979=CARTESIAN_POINT ( 'NONE',  ( 1.989345975306457071, 16.00319992234354771, 1.515154207786300500 ) ) ;
#6982=CARTESIAN_POINT ( 'NONE',  ( 3.518350579753631191, 34.37180007765648071, 1.080741659609802729 ) ) ;
#6986=CARTESIAN_POINT ( 'NONE',  ( 1.027846397803542144, 33.74680007765648071, -3.346150245485522312 ) ) ;
#6995=VERTEX_POINT ( 'NONE', #5831 ) ;
#6998=CARTESIAN_POINT ( 'NONE',  ( -1.497042530366477164, 17.62180007765648071, 2.161531897785062384 ) ) ;
#7001=CARTESIAN_POINT ( 'NONE',  ( -4.499999999999999112, 17.99680007765647005, 0.05647727720537927543 ) ) ;
#7004=CARTESIAN_POINT ( 'NONE',  ( 0.8262555684460829442, 35.25319992234354771, -2.360188852285421302 ) ) ;
#7007=CARTESIAN_POINT ( 'NONE',  ( 1.444289557196047680, 37.24680007765646650, 4.262301884875704161 ) ) ;
#7022=( LENGTH_UNIT ( ) NAMED_UNIT ( * ) SI_UNIT ( .MILLI., .METRE. ) );
#7023=CARTESIAN_POINT ( 'NONE',  ( -4.518350579753602325, 21.87819992234354416, 1.405661355842794391 ) ) ;
#7025=CARTESIAN_POINT ( 'NONE',  ( 1.135272562821020070, 17.75319992234354771, -3.311245368580577164 ) ) ;
#7027=CARTESIAN_POINT ( 'NONE',  ( -0.7188294034286043521, 37.49680007765647360, 2.395093729190366005 ) ) ;
#7030=CARTESIAN_POINT ( 'NONE',  ( -2.733110507866328476, 32.37819992234353350, -3.862833514489096398 ) ) ;
#7035=CARTESIAN_POINT ( 'NONE',  ( -1.055605843668875110, 15.00000000000000888, -3.337496964141338562 ) ) ;
#7036=CARTESIAN_POINT ( 'NONE',  ( -2.864755990943265829, 23.24680007765647716, -2.011557305968488141 ) ) ;
#7039=CARTESIAN_POINT ( 'NONE',  ( 0.05938372350929014415, 19.87180007765647716, 4.731580009072201776 ) ) ;
#7046=CARTESIAN_POINT ( 'NONE',  ( -0.05938372350927861171, 23.62180007765647005, -3.680117784833935701 ) ) ;
#7052=CARTESIAN_POINT ( 'NONE',  ( 3.500000000000000444, 23.25319992234354416, 0.05647727720529520379 ) ) ;
#7054=CARTESIAN_POINT ( 'NONE',  ( -3.518350579753630747, 38.12180007765648071, -1.080741659609802729 ) ) ;
#7055=CARTESIAN_POINT ( 'NONE',  ( -0.05938372350920063936, 23.87819992234354416, 3.680117784833935701 ) ) ;
#7070=CARTESIAN_POINT ( 'NONE',  ( -2.481649420246391902, 17.12819992234354416, -0.8687765177875723666 ) ) ;
#7072=CARTESIAN_POINT ( 'NONE',  ( 3.500000000000000444, 36.74680007765648071, -0.05647727720536935281 ) ) ;
#7078=CARTESIAN_POINT ( 'NONE',  ( 1.027846397803542144, 31.24680007765647716, -3.346150245485522312 ) ) ;
#7091=CARTESIAN_POINT ( 'NONE',  ( -1.497042530366477164, 22.62180007765647716, 2.161531897785062384 ) ) ;
#7098=CARTESIAN_POINT ( 'NONE',  ( -2.500000000000001332, 34.50319992234354771, -0.05647727720530596601 ) ) ;
#7102=CARTESIAN_POINT ( 'NONE',  ( -4.499999999999999112, 30.49680007765648071, 0.05647727720537927543 ) ) ;
#7118=CARTESIAN_POINT ( 'NONE',  ( -3.673772985318163098, 16.75319992234354416, 2.599342558261029001 ) ) ;
#7119=CARTESIAN_POINT ( 'NONE',  ( -2.798362969681409851, 29.75319992234354416, -2.102939460078765421 ) ) ;
#7121=CARTESIAN_POINT ( 'NONE',  ( 0.8262555684461332373, 39.74680007765648071, 2.360188852285403982 ) ) ;
#7123=CARTESIAN_POINT ( 'NONE',  ( 4.518350579753602325, 35.62819992234354771, -1.405661355842793725 ) ) ;
#7128=CARTESIAN_POINT ( 'NONE',  ( -2.115076519116362519, 22.62180007765647360, 3.012182706137107147 ) ) ;
#7131=CARTESIAN_POINT ( 'NONE',  ( -1.444289557196047014, 25.99680007765648071, -4.262301884875704161 ) ) ;
#7136=CARTESIAN_POINT ( 'NONE',  ( -3.481649420246369697, 20.37180007765647716, 1.193696214020542490 ) ) ;
#7143=CARTESIAN_POINT ( 'NONE',  ( 0.05938372350920109732, 20.12819992234353705, -3.680117784833935701 ) ) ;
#7145=CARTESIAN_POINT ( 'NONE',  ( 2.481649420246374138, 16.62180007765648071, -0.8687765177876252132 ) ) ;
#7146=CARTESIAN_POINT ( 'NONE',  ( -1.027846397803611866, 35.00319992234354771, -3.346150245485499219 ) ) ;
#7163=CARTESIAN_POINT ( 'NONE',  ( -2.055738996568281518, 24.25319992234354061, 1.423772053676066962 ) ) ;
#7171=CARTESIAN_POINT ( 'NONE',  ( -1.027846397803541700, 29.99680007765648071, 3.346150245485522312 ) ) ;
#7185=CARTESIAN_POINT ( 'NONE',  ( -2.518350579753628526, 20.62180007765647716, -0.7558219633769075463 ) ) ;
#7187=CARTESIAN_POINT ( 'NONE',  ( 3.518350579753631191, 21.87180007765647360, 1.080741659609802729 ) ) ;
#7191=CARTESIAN_POINT ( 'NONE',  ( -2.055738996568281518, 36.75319992234354771, 1.423772053676066962 ) ) ;
#7194=CARTESIAN_POINT ( 'NONE',  ( 1.336863392178479160, 33.74680007765647360, -4.297206761780677731 ) ) ;
#7212=CARTESIAN_POINT ( 'NONE',  ( 2.733110507866328920, 16.12819992234354416, 3.862833514489095510 ) ) ;
#7213=CARTESIAN_POINT ( 'NONE',  ( -3.500000000000000444, 27.00319992234354771, -0.05647727720529563400 ) ) ;
#7214=CARTESIAN_POINT ( 'NONE',  ( 1.497042530366477164, 38.87180007765646650, -2.161531897785062384 ) ) ;
#7216=CARTESIAN_POINT ( 'NONE',  ( 4.499999999999999112, 30.75319992234354416, 0.05647727720528474687 ) ) ;
#7220=CARTESIAN_POINT ( 'NONE',  ( -3.500000000000000444, 27.99680007765648071, 0.05647727720536892260 ) ) ;
#7223=CARTESIAN_POINT ( 'NONE',  ( 1.336863392178479160, 31.24680007765648071, -4.297206761780677731 ) ) ;
#7227=CARTESIAN_POINT ( 'NONE',  ( 0.05938372350927906274, 27.37180007765647716, 3.680117784833935701 ) ) ;
#7232=CARTESIAN_POINT ( 'NONE',  ( 2.211161402132839626, 20.37819992234354416, -2.942372952327218183 ) ) ;
#7235=CARTESIAN_POINT ( 'NONE',  ( -0.05938372350927861171, 36.12180007765648782, -3.680117784833935701 ) ) ;
#7237=CARTESIAN_POINT ( 'NONE',  ( 2.798362969681409851, 31.00319992234354416, 2.102939460078764977 ) ) ;
#7246=CARTESIAN_POINT ( 'NONE',  ( -1.055605843668875110, 15.00000000000000888, -3.337496964141338562 ) ) ;
#7249=CARTESIAN_POINT ( 'NONE',  ( -0.7188294034286550893, 20.00319992234354771, -2.395093729190349130 ) ) ;
#7251=CARTESIAN_POINT ( 'NONE',  ( 3.518350579753631191, 16.87180007765648071, 1.080741659609802285 ) ) ;
#7257=CARTESIAN_POINT ( 'NONE',  ( 2.864755990943265829, 34.49680007765648071, 2.011557305968487697 ) ) ;
#7272=CARTESIAN_POINT ( 'NONE',  ( -0.7188294034286043521, 22.49680007765648071, 2.395093729190366005 ) ) ;
#7274=CARTESIAN_POINT ( 'NONE',  ( -2.211161402132901799, 25.87180007765647360, -2.942372952327172886 ) ) ;
#7279=CARTESIAN_POINT ( 'NONE',  ( 2.500000000000001332, 33.25319992234354771, 0.05647727720530566764 ) ) ;
#7282=CARTESIAN_POINT ( 'NONE',  ( -4.518350579753632523, 30.62180007765647005, -1.405661355842698468 ) ) ;
#7299=CARTESIAN_POINT ( 'NONE',  ( 0.05938372350919016857, 20.12819992234354416, -4.731580009072201776 ) ) ;
#7300=CARTESIAN_POINT ( 'NONE',  ( 3.481649420246395010, 25.87819992234354771, 1.193696214020467439 ) ) ;
#7301=CARTESIAN_POINT ( 'NONE',  ( -2.500000000000001332, 37.99680007765646650, 0.05647727720535858364 ) ) ;
#7303=CARTESIAN_POINT ( 'NONE',  ( 2.829195390882724759, 30.37819992234354061, -3.793023760679264278 ) ) ;
#7309=CARTESIAN_POINT ( 'NONE',  ( -3.500000000000000444, 30.49680007765647716, 0.05647727720536892260 ) ) ;
#7312=CARTESIAN_POINT ( 'NONE',  ( -0.05938372350928957516, 31.12180007765647716, -4.731580009072201776 ) ) ;
#7316=CARTESIAN_POINT ( 'NONE',  ( 2.798362969681366330, 23.99680007765647716, -2.102939460078824929 ) ) ;
#7322=CARTESIAN_POINT ( 'NONE',  ( -3.518350579753605434, 19.37819992234354416, 1.080741659609877781 ) ) ;
#7327=CARTESIAN_POINT ( 'NONE',  ( 0.8262555684461332373, 17.24680007765648071, 2.360188852285403982 ) ) ;
#7329=CARTESIAN_POINT ( 'NONE',  ( -3.481649420246394122, 34.62819992234354771, -1.193696214020467883 ) ) ;
#7345=CARTESIAN_POINT ( 'NONE',  ( -1.497042530366522461, 19.87819992234354771, -2.161531897785030409 ) ) ;
#7347=CARTESIAN_POINT ( 'NONE',  ( 2.115076519116362963, 16.37180007765647716, -3.012182706137107147 ) ) ;
#7348=CARTESIAN_POINT ( 'NONE',  ( 0.05938372350929014415, 17.37180007765647716, 4.731580009072201776 ) ) ;
#7355=CARTESIAN_POINT ( 'NONE',  ( 2.211161402132902243, 39.62180007765646650, 2.942372952327172442 ) ) ;
#7366=CARTESIAN_POINT ( 'NONE',  ( -2.518350579753628526, 25.62180007765648426, -0.7558219633769075463 ) ) ;
#7368=CARTESIAN_POINT ( 'NONE',  ( -1.135272562821090014, 18.49680007765648071, -3.311245368580554072 ) ) ;
#7372=CARTESIAN_POINT ( 'NONE',  ( 1.135272562821020070, 17.75319992234354771, -3.311245368580577164 ) ) ;
#7376=CARTESIAN_POINT ( 'NONE',  ( 1.444289557196047680, 32.24680007765647360, 4.262301884875704161 ) ) ;
#7397=CARTESIAN_POINT ( 'NONE',  ( -3.673772985318163098, 26.75319992234354771, 2.599342558261029001 ) ) ;
#7398=CARTESIAN_POINT ( 'NONE',  ( 2.115076519116425580, 31.12819992234354416, 3.012182706137062294 ) ) ;
#7399=CARTESIAN_POINT ( 'NONE',  ( 1.593127413382998903, 39.62180007765647360, 2.091722143975139669 ) ) ;
#7401=CARTESIAN_POINT ( 'NONE',  ( 4.518350579753602325, 30.62819992234354416, -1.405661355842793725 ) ) ;
#7406=CARTESIAN_POINT ( 'NONE',  ( -3.481649420246369697, 30.37180007765647005, 1.193696214020542490 ) ) ;
#7410=CARTESIAN_POINT ( 'NONE',  ( 4.499999999999999112, 31.74680007765647716, -0.05647727720537982360 ) ) ;
#7413=CARTESIAN_POINT ( 'NONE',  ( -3.481649420246369697, 27.87180007765647360, 1.193696214020542490 ) ) ;
#7419=AXIS2_PLACEMENT_3D ( 'NONE', #11721, #12841, #3024 ) ;
#7420=CARTESIAN_POINT ( 'NONE',  ( 3.481649420246394122, 28.37819992234354416, 1.193696214020467439 ) ) ;
#7423=CARTESIAN_POINT ( 'NONE',  ( -2.798362969681365886, 37.74680007765647360, 2.102939460078824929 ) ) ;
#7425=CARTESIAN_POINT ( 'NONE',  ( -1.027846397803611866, 37.50319992234354061, -3.346150245485499219 ) ) ;
#7442=CARTESIAN_POINT ( 'NONE',  ( 1.497042530366522461, 21.12819992234354416, 2.161531897785029965 ) ) ;
#7445=CARTESIAN_POINT ( 'NONE',  ( -2.211161402132902243, 15.87180007765647716, -2.942372952327172886 ) ) ;
#7450=CARTESIAN_POINT ( 'NONE',  ( 1.135272562821090458, 37.24680007765648071, 3.311245368580554072 ) ) ;
#7462=CARTESIAN_POINT ( 'NONE',  ( 2.055738996568313048, 24.49680007765648426, 1.423772053676023441 ) ) ;
#7465=CARTESIAN_POINT ( 'NONE',  ( -1.135272562821090014, 23.49680007765647716, -3.311245368580554072 ) ) ;
#7470=CARTESIAN_POINT ( 'NONE',  ( 3.518350579753605434, 20.62819992234354771, -1.080741659609877114 ) ) ;
#7473=CARTESIAN_POINT ( 'NONE',  ( -2.829195390882805139, 38.37180007765647360, -3.793023760679206102 ) ) ;
#7491=CARTESIAN_POINT ( 'NONE',  ( -1.444289557195956863, 26.50319992234354771, 4.262301884875733471 ) ) ;
#7492=CARTESIAN_POINT ( 'NONE',  ( -1.027846397803611866, 30.00319992234354416, -3.346150245485499219 ) ) ;
#7493=CARTESIAN_POINT ( 'NONE',  ( -1.593127413382952939, 19.12819992234354771, 2.091722143975172532 ) ) ;
#7495=CARTESIAN_POINT ( 'NONE',  ( 2.733110507866328920, 38.62819992234354771, 3.862833514489095510 ) ) ;
#7501=CARTESIAN_POINT ( 'NONE',  ( -1.027846397803541700, 29.99680007765648071, 3.346150245485522312 ) ) ;
#7505=CARTESIAN_POINT ( 'NONE',  ( -4.518350579753632523, 30.62180007765647005, -1.405661355842698468 ) ) ;
#7511=CARTESIAN_POINT ( 'NONE',  ( 3.500000000000000444, 29.24680007765647716, -0.05647727720536935281 ) ) ;
#7517=CARTESIAN_POINT ( 'NONE',  ( -2.211161402132839182, 24.12819992234354416, 2.942372952327218627 ) ) ;
#7520=CARTESIAN_POINT ( 'NONE',  ( -0.7188294034286043521, 22.49680007765648071, 2.395093729190366005 ) ) ;
#7522=CARTESIAN_POINT ( 'NONE',  ( 3.481649420246394122, 33.37819992234353350, 1.193696214020467439 ) ) ;
#7537=CARTESIAN_POINT ( 'NONE',  ( 0.05938372350921204690, 30.12819992234354416, -2.628655560595669183 ) ) ;
#7539=CARTESIAN_POINT ( 'NONE',  ( 2.115076519116362963, 26.37180007765648071, -3.012182706137107147 ) ) ;
#7543=CARTESIAN_POINT ( 'NONE',  ( 0.05938372350927906274, 39.87180007765648071, 3.680117784833935701 ) ) ;
#7553=CARTESIAN_POINT ( 'NONE',  ( -0.05938372350926768989, 31.12180007765648426, -2.628655560595669183 ) ) ;
#7555=CARTESIAN_POINT ( 'NONE',  ( -1.027846397803541700, 24.99680007765647716, 3.346150245485522312 ) ) ;
#7559=CARTESIAN_POINT ( 'NONE',  ( 2.115076519116426024, 18.62819992234354771, 3.012182706137062294 ) ) ;
#7562=CARTESIAN_POINT ( 'NONE',  ( 3.481649420246369697, 16.62180007765648071, -1.193696214020541824 ) ) ;
#7582=CARTESIAN_POINT ( 'NONE',  ( -2.733110507866328476, 22.37819992234354416, -3.862833514489096398 ) ) ;
#7583=CARTESIAN_POINT ( 'NONE',  ( -3.518350579753606322, 36.87819992234354061, 1.080741659609877781 ) ) ;
#7584=CARTESIAN_POINT ( 'NONE',  ( -0.7188294034286550893, 22.50319992234354771, -2.395093729190349130 ) ) ;
#7586=CARTESIAN_POINT ( 'NONE',  ( -2.829195390882724315, 39.12819992234354771, 3.793023760679264722 ) ) ;
#7590=CARTESIAN_POINT ( 'NONE',  ( -1.135272562821090014, 28.49680007765648071, -3.311245368580554072 ) ) ;
#7595=CARTESIAN_POINT ( 'NONE',  ( 0.05938372350929014415, 27.37180007765647716, 4.731580009072201776 ) ) ;
#7598=CARTESIAN_POINT ( 'NONE',  ( 2.798362969681366330, 33.99680007765648071, -2.102939460078824929 ) ) ;
#7603=CARTESIAN_POINT ( 'NONE',  ( 3.518350579753605434, 25.62819992234353705, -1.080741659609877114 ) ) ;
#7607=CARTESIAN_POINT ( 'NONE',  ( -2.500000000000001332, 22.99680007765648071, 0.05647727720535858364 ) ) ;
#7608=CARTESIAN_POINT ( 'NONE',  ( 2.733110507866328920, 16.12819992234354416, 3.862833514489095510 ) ) ;
#7624=CARTESIAN_POINT ( 'NONE',  ( 0.7188294034286553114, 28.75319992234354771, 2.395093729190349130 ) ) ;
#7627=CARTESIAN_POINT ( 'NONE',  ( 2.864755990943265829, 24.49680007765647716, 2.011557305968487697 ) ) ;
#7643=CARTESIAN_POINT ( 'NONE',  ( 0.8262555684461332373, 29.74680007765648426, 2.360188852285403982 ) ) ;
#7646=CARTESIAN_POINT ( 'NONE',  ( -1.135272562821090014, 30.99680007765647716, -3.311245368580554072 ) ) ;
#7649=CARTESIAN_POINT ( 'NONE',  ( 1.135272562821020070, 15.25319992234354594, -3.311245368580577164 ) ) ;
#7652=CARTESIAN_POINT ( 'NONE',  ( -3.607379964056306676, 40.24680007765648071, 2.690724712371306282 ) ) ;
#7676=CARTESIAN_POINT ( 'NONE',  ( 4.481649420246397675, 28.37819992234355126, 1.518615910253363177 ) ) ;
#7677=CARTESIAN_POINT ( 'NONE',  ( 2.864755990943222308, 35.50319992234354771, -2.011557305968548093 ) ) ;
#7680=CARTESIAN_POINT ( 'NONE',  ( 0.7188294034286553114, 23.75319992234354771, 2.395093729190349130 ) ) ;
#7682=CARTESIAN_POINT ( 'NONE',  ( 4.481649420246397675, 38.37819992234354061, 1.518615910253363177 ) ) ;
#7687=CARTESIAN_POINT ( 'NONE',  ( 3.500000000000000444, 34.24680007765648071, -0.05647727720536935281 ) ) ;
#7699=CARTESIAN_POINT ( 'NONE',  ( 1.027846397803612311, 28.75319992234354416, 3.346150245485499219 ) ) ;
#7700=CARTESIAN_POINT ( 'NONE',  ( 3.518350579753606322, 15.62819992234354416, -1.080741659609876892 ) ) ;
#7702=CARTESIAN_POINT ( 'NONE',  ( -2.481649420246374138, 20.37180007765648426, 0.8687765177876256573 ) ) ;
#7704=CARTESIAN_POINT ( 'NONE',  ( -3.607379964056363075, 17.25319992234354416, -2.690724712371229899 ) ) ;
#7709=CARTESIAN_POINT ( 'NONE',  ( 3.607379964056306676, 38.99680007765648071, -2.690724712371305838 ) ) ;
#7720=CARTESIAN_POINT ( 'NONE',  ( 2.500000000000001332, 30.75319992234354416, 0.05647727720530566764 ) ) ;
#7722=CARTESIAN_POINT ( 'NONE',  ( 1.135272562821090458, 24.74680007765647716, 3.311245368580554072 ) ) ;
#7741=CARTESIAN_POINT ( 'NONE',  ( -2.055738996568313048, 30.74680007765648071, -1.423772053676023441 ) ) ;
#7743=CARTESIAN_POINT ( 'NONE',  ( -2.864755990943265829, 28.24680007765648071, -2.011557305968488141 ) ) ;
#7750=CARTESIAN_POINT ( 'NONE',  ( -3.607379964056306676, 37.74680007765647360, 2.690724712371306282 ) ) ;
#7769=CARTESIAN_POINT ( 'NONE',  ( 0.05938372350919016857, 22.62819992234354416, -4.731580009072201776 ) ) ;
#7770=CARTESIAN_POINT ( 'NONE',  ( -3.500000000000000444, 39.50319992234354061, -0.05647727720529600870 ) ) ;
#7771=CARTESIAN_POINT ( 'NONE',  ( -2.500000000000001332, 19.50319992234354771, -0.05647727720530596601 ) ) ;
#7773=CARTESIAN_POINT ( 'NONE',  ( -4.518350579753632523, 15.62180007765647360, -1.405661355842698468 ) ) ;
#7794=CARTESIAN_POINT ( 'NONE',  ( -2.798362969681409851, 24.75319992234354416, -2.102939460078765421 ) ) ;
#7797=CARTESIAN_POINT ( 'NONE',  ( -2.481649420246374138, 22.87180007765648071, 0.8687765177876256573 ) ) ;
#7798=CARTESIAN_POINT ( 'NONE',  ( -3.673772985318163098, 19.25319992234354416, 2.599342558261029001 ) ) ;
#7802=CARTESIAN_POINT ( 'NONE',  ( -3.518350579753630747, 15.62180007765647538, -1.080741659609802729 ) ) ;
#7813=CARTESIAN_POINT ( 'NONE',  ( -1.497042530366522461, 32.37819992234353350, -2.161531897785030409 ) ) ;
#7816=CARTESIAN_POINT ( 'NONE',  ( -3.518350579753630747, 25.62180007765648071, -1.080741659609802729 ) ) ;
#7829=CARTESIAN_POINT ( 'NONE',  ( 0.05938372350926800214, 32.37180007765648782, 2.628655560595669183 ) ) ;
#7831=CARTESIAN_POINT ( 'NONE',  ( 3.481649420246370141, 31.62180007765647005, -1.193696214020541602 ) ) ;
#7841=CARTESIAN_POINT ( 'NONE',  ( 2.733110507866247652, 38.87180007765646650, -3.862833514489153686 ) ) ;
#7856=CARTESIAN_POINT ( 'NONE',  ( -4.499999999999999112, 34.50319992234354771, -0.05647727720528529505 ) ) ;
#7857=CARTESIAN_POINT ( 'NONE',  ( 0.05938372350920110426, 37.62819992234353350, -3.680117784833935701 ) ) ;
#7858=CARTESIAN_POINT ( 'NONE',  ( -1.593127413382952939, 24.12819992234354771, 2.091722143975172532 ) ) ;
#7861=CARTESIAN_POINT ( 'NONE',  ( -3.673772985318219053, 20.74680007765647716, -2.599342558260952174 ) ) ;
#7865=CARTESIAN_POINT ( 'NONE',  ( -3.500000000000000444, 35.49680007765648071, 0.05647727720536892260 ) ) ;
#7878=CARTESIAN_POINT ( 'NONE',  ( 3.500000000000000444, 33.25319992234354771, 0.05647727720529520379 ) ) ;
#7881=CARTESIAN_POINT ( 'NONE',  ( 2.055738996568313048, 21.99680007765648426, 1.423772053676023441 ) ) ;
#7882=CARTESIAN_POINT ( 'NONE',  ( 0.05938372350919016857, 15.12819992234354594, -4.731580009072201776 ) ) ;
#7887=CARTESIAN_POINT ( 'NONE',  ( 4.499999999999999112, 39.24680007765647360, -0.05647727720537982360 ) ) ;
#7895=CARTESIAN_POINT ( 'NONE',  ( 2.115076519116362963, 16.37180007765647716, -3.012182706137107147 ) ) ;
#7900=CARTESIAN_POINT ( 'NONE',  ( -2.055738996568281518, 26.75319992234354771, 1.423772053676066962 ) ) ;
#7904=CARTESIAN_POINT ( 'NONE',  ( 3.481649420246369697, 24.12180007765648071, -1.193696214020541824 ) ) ;
#7912=CARTESIAN_POINT ( 'NONE',  ( 3.607379964056306676, 21.49680007765647360, -2.690724712371305838 ) ) ;
#7919=CARTESIAN_POINT ( 'NONE',  ( -2.481649420246374138, 30.37180007765648426, 0.8687765177876256573 ) ) ;
#7921=CARTESIAN_POINT ( 'NONE',  ( 0.05938372350927906967, 29.87180007765647716, 3.680117784833935701 ) ) ;
#7930=CARTESIAN_POINT ( 'NONE',  ( 3.500000000000000444, 24.24680007765647716, -0.05647727720536935281 ) ) ;
#7944=CARTESIAN_POINT ( 'NONE',  ( -2.864755990943265829, 33.24680007765648071, -2.011557305968488141 ) ) ;
#7947=APPLICATION_CONTEXT ( 'automotive_design' ) ;
#7949=CARTESIAN_POINT ( 'NONE',  ( 4.499999999999999112, 30.75319992234354416, 0.05647727720528474687 ) ) ;
#7950=CARTESIAN_POINT ( 'NONE',  ( 2.115076519116425580, 36.12819992234355482, 3.012182706137062294 ) ) ;
#7951=CARTESIAN_POINT ( 'NONE',  ( -2.481649420246391902, 29.62819992234354416, -0.8687765177875723666 ) ) ;
#7953=CARTESIAN_POINT ( 'NONE',  ( 3.673772985318219053, 24.49680007765648071, 2.599342558260951730 ) ) ;
#7976=CARTESIAN_POINT ( 'NONE',  ( -2.864755990943222308, 39.25319992234354771, 2.011557305968548093 ) ) ;
#7979=CARTESIAN_POINT ( 'NONE',  ( -2.518350579753628526, 30.62180007765647716, -0.7558219633769075463 ) ) ;
#7980=CARTESIAN_POINT ( 'NONE',  ( -2.733110507866328476, 19.87819992234354416, -3.862833514489096398 ) ) ;
#7984=CARTESIAN_POINT ( 'NONE',  ( -3.500000000000000444, 17.99680007765647716, 0.05647727720536892260 ) ) ;
#7996=CARTESIAN_POINT ( 'NONE',  ( -2.115076519116425580, 14.87819992234354594, -3.012182706137062738 ) ) ;
#7998=CARTESIAN_POINT ( 'NONE',  ( -0.05938372350927861171, 31.12180007765647005, -3.680117784833935701 ) ) ;
#7999=CARTESIAN_POINT ( 'NONE',  ( 2.798362969681409851, 16.00319992234354416, 2.102939460078764977 ) ) ;
#8006=CARTESIAN_POINT ( 'NONE',  ( 3.673772985318219053, 26.99680007765647716, 2.599342558260951730 ) ) ;
#8014=CARTESIAN_POINT ( 'NONE',  ( -0.7188294034286043521, 37.49680007765647360, 2.395093729190366005 ) ) ;
#8016=CARTESIAN_POINT ( 'NONE',  ( -3.518350579753630303, 33.12180007765646650, -1.080741659609802952 ) ) ;
#8023=CARTESIAN_POINT ( 'NONE',  ( 1.027846397803542144, 26.24680007765648071, -3.346150245485522312 ) ) ;
#8027=CARTESIAN_POINT ( 'NONE',  ( -4.000000000000000000, 15.00000000000000355, 4.083367561434192880E-14 ) ) ;
#8036=CARTESIAN_POINT ( 'NONE',  ( -3.500000000000000444, 35.49680007765648071, 0.05647727720536892260 ) ) ;
#8037=ORIENTED_EDGE ( 'NONE', *, *, #4562, .F. ) ;
#8040=CARTESIAN_POINT ( 'NONE',  ( -0.05938372350918959958, 36.37819992234354771, 4.731580009072201776 ) ) ;
#8042=CARTESIAN_POINT ( 'NONE',  ( -0.7188294034286550893, 30.00319992234354416, -2.395093729190349130 ) ) ;
#8044=CARTESIAN_POINT ( 'NONE',  ( 4.518350579753633411, 29.37180007765647716, 1.405661355842698468 ) ) ;
#8048=CARTESIAN_POINT ( 'NONE',  ( -2.798362969681365886, 37.74680007765647360, 2.102939460078824929 ) ) ;
#8059=CARTESIAN_POINT ( 'NONE',  ( 2.864755990943222308, 35.50319992234354771, -2.011557305968548093 ) ) ;
#8060=CARTESIAN_POINT ( 'NONE',  ( -2.864755990943222308, 19.25319992234354416, 2.011557305968548093 ) ) ;
#8062=CARTESIAN_POINT ( 'NONE',  ( -2.055738996568313048, 33.24680007765648782, -1.423772053676023441 ) ) ;
#8065=CARTESIAN_POINT ( 'NONE',  ( 1.336863392178569754, 23.75319992234354771, 4.297206761780648421 ) ) ;
#8073=CARTESIAN_POINT ( 'NONE',  ( -1.444289557196047014, 35.99680007765647360, -4.262301884875704161 ) ) ;
#8086=ORIENTED_EDGE ( 'NONE', *, *, #10080, .T. ) ;
#8087=CARTESIAN_POINT ( 'NONE',  ( 1.497042530366522461, 33.62819992234354771, 2.161531897785029965 ) ) ;
#8089=CARTESIAN_POINT ( 'NONE',  ( 1.027846397803542144, 31.24680007765647716, -3.346150245485522312 ) ) ;
#8090=CARTESIAN_POINT ( 'NONE',  ( 1.135272562821020070, 27.75319992234354416, -3.311245368580577164 ) ) ;
#8096=CARTESIAN_POINT ( 'NONE',  ( -4.518350579753632523, 20.62180007765647716, -1.405661355842698468 ) ) ;
#8105=CARTESIAN_POINT ( 'NONE',  ( 0.8262555684461332373, 39.74680007765648071, 2.360188852285403982 ) ) ;
#8107=CARTESIAN_POINT ( 'NONE',  ( 2.211161402132902243, 39.62180007765646650, 2.942372952327172442 ) ) ;
#8114=CARTESIAN_POINT ( 'NONE',  ( 3.518350579753631191, 26.87180007765647360, 1.080741659609802285 ) ) ;
#8127=CARTESIAN_POINT ( 'NONE',  ( 0.05938372350927906274, 37.37180007765645939, 3.680117784833935701 ) ) ;
#8130=CARTESIAN_POINT ( 'NONE',  ( 1.444289557195957086, 37.75319992234354771, -4.262301884875733471 ) ) ;
#8132=CARTESIAN_POINT ( 'NONE',  ( 1.989345975306457071, 31.00319992234355126, 1.515154207786300500 ) ) ;
#8136=CARTESIAN_POINT ( 'NONE',  ( -1.336863392178478716, 22.49680007765647360, 4.297206761780677731 ) ) ;
#8150=CARTESIAN_POINT ( 'NONE',  ( -1.027846397803541700, 17.49680007765647716, 3.346150245485522312 ) ) ;
#8153=CARTESIAN_POINT ( 'NONE',  ( 1.135272562821020070, 37.75319992234354061, -3.311245368580577164 ) ) ;
#8154=CARTESIAN_POINT ( 'NONE',  ( 3.518350579753606322, 18.12819992234354416, -1.080741659609876892 ) ) ;
#8156=CARTESIAN_POINT ( 'NONE',  ( 1.593127413382998903, 32.12180007765648071, 2.091722143975139669 ) ) ;
#8157=CARTESIAN_POINT ( 'NONE',  ( 4.499999999999999112, 25.75319992234354771, 0.05647727720528474687 ) ) ;
#8161=CARTESIAN_POINT ( 'NONE',  ( 0.05938372350927906274, 24.87180007765647005, 3.680117784833935701 ) ) ;
#8178=CARTESIAN_POINT ( 'NONE',  ( -0.7188294034286550893, 32.50319992234354771, -2.395093729190349130 ) ) ;
#8180=CARTESIAN_POINT ( 'NONE',  ( -3.518350579753630747, 28.12180007765647360, -1.080741659609802729 ) ) ;
#8181=CARTESIAN_POINT ( 'NONE',  ( -2.211161402132839182, 26.62819992234353705, 2.942372952327218627 ) ) ;
#8191=CARTESIAN_POINT ( 'NONE',  ( -3.500000000000000444, 15.00000000000001243, 3.664603343001004987E-14 ) ) ;
#8192=AXIS2_PLACEMENT_3D ( 'NONE', #1067, #791, #5043 ) ;
#8196=CARTESIAN_POINT ( 'NONE',  ( -2.481649420246374138, 37.87180007765647360, 0.8687765177876256573 ) ) ;
#8198=CARTESIAN_POINT ( 'NONE',  ( 1.027846397803542144, 36.24680007765648071, -3.346150245485522312 ) ) ;
#8205=CARTESIAN_POINT ( 'NONE',  ( 2.211161402132902243, 22.12180007765648071, 2.942372952327172442 ) ) ;
#8217=CARTESIAN_POINT ( 'NONE',  ( 1.593127413382998903, 17.12180007765648426, 2.091722143975139669 ) ) ;
#8222=CARTESIAN_POINT ( 'NONE',  ( 2.733110507866328920, 31.12819992234354416, 3.862833514489095510 ) ) ;
#8224=CARTESIAN_POINT ( 'NONE',  ( 2.055738996568281518, 28.00319992234354771, -1.423772053676066518 ) ) ;
#8228=CARTESIAN_POINT ( 'NONE',  ( -2.733110507866247652, 27.62180007765647716, 3.862833514489154574 ) ) ;
#8237=ADVANCED_FACE ( 'NONE', ( #6252 ), #17317, .F. ) ;
#8247=CARTESIAN_POINT ( 'NONE',  ( -3.518350579753630303, 15.62180007765647716, -1.080741659609802952 ) ) ;
#8251=CARTESIAN_POINT ( 'NONE',  ( 3.500000000000000444, 38.25319992234354061, 0.05647727720529520379 ) ) ;
#8252=CARTESIAN_POINT ( 'NONE',  ( -3.518350579753606322, 21.87819992234354771, 1.080741659609877781 ) ) ;
#8255=CARTESIAN_POINT ( 'NONE',  ( 2.055738996568313048, 26.99680007765647716, 1.423772053676023441 ) ) ;
#8256=CARTESIAN_POINT ( 'NONE',  ( 1.444289557195957086, 25.25319992234354771, -4.262301884875733471 ) ) ;
#8261=CARTESIAN_POINT ( 'NONE',  ( 3.481649420246369697, 19.12180007765648071, -1.193696214020541824 ) ) ;
#8275=CARTESIAN_POINT ( 'NONE',  ( 2.055738996568281518, 38.00319992234354061, -1.423772053676066518 ) ) ;
#8278=CARTESIAN_POINT ( 'NONE',  ( -3.481649420246369697, 32.87180007765645939, 1.193696214020542490 ) ) ;
#8280=CARTESIAN_POINT ( 'NONE',  ( 3.481649420246394122, 25.87819992234354771, 1.193696214020467439 ) ) ;
#8291=CARTESIAN_POINT ( 'NONE',  ( -0.7188294034286550893, 15.00319992234354594, -2.395093729190349130 ) ) ;
#8292=CARTESIAN_POINT ( 'NONE',  ( 0.05938372350927906967, 34.87180007765646650, 3.680117784833935701 ) ) ;
#8294=CARTESIAN_POINT ( 'NONE',  ( -1.064077915893153703, 15.00000000000000178, -3.362852706530892632 ) ) ;
#8298=CARTESIAN_POINT ( 'NONE',  ( -2.798362969681365886, 25.24680007765647716, 2.102939460078824929 ) ) ;
#8303=PLANE ( 'NONE',  #13810 ) ;
#8312=CARTESIAN_POINT ( 'NONE',  ( 1.135272562821090458, 37.24680007765648071, 3.311245368580554072 ) ) ;
#8314=CARTESIAN_POINT ( 'NONE',  ( -3.673772985318219053, 15.74680007765647716, -2.599342558260952174 ) ) ;
#8316=CARTESIAN_POINT ( 'NONE',  ( -2.055738996568281518, 39.25319992234354771, 1.423772053676066962 ) ) ;
#8319=CARTESIAN_POINT ( 'NONE',  ( 4.481649420246366589, 24.12180007765647716, -1.518615910253458212 ) ) ;
#8334=( NAMED_UNIT ( * ) SI_UNIT ( $, .STERADIAN. ) SOLID_ANGLE_UNIT ( ) );
#8336=CARTESIAN_POINT ( 'NONE',  ( 2.829195390882724759, 15.37819992234354594, -3.793023760679264278 ) ) ;
#8337=CARTESIAN_POINT ( 'NONE',  ( 2.211161402132839182, 20.37819992234354416, -2.942372952327217739 ) ) ;
#8339=CARTESIAN_POINT ( 'NONE',  ( -2.055738996568313048, 28.24680007765648071, -1.423772053676023441 ) ) ;
#8340=CARTESIAN_POINT ( 'NONE',  ( -1.336863392178569088, 25.00319992234354771, -4.297206761780648421 ) ) ;
#8346=CARTESIAN_POINT ( 'NONE',  ( 0.05938372350927906274, 19.87180007765648426, 3.680117784833935701 ) ) ;
#8356=CARTESIAN_POINT ( 'NONE',  ( -0.05938372350927861171, 26.12180007765647005, -3.680117784833935701 ) ) ;
#8362=CARTESIAN_POINT ( 'NONE',  ( -1.593127413382952939, 36.62819992234354771, 2.091722143975172532 ) ) ;
#8364=CARTESIAN_POINT ( 'NONE',  ( -3.500000000000000444, 32.99680007765648071, 0.05647727720536892260 ) ) ;
#8365=CARTESIAN_POINT ( 'NONE',  ( 3.518350579753605434, 30.62819992234353705, -1.080741659609877114 ) ) ;
#8376=CARTESIAN_POINT ( 'NONE',  ( -0.8262555684461330152, 38.49680007765647360, -2.360188852285403982 ) ) ;
#8383=CARTESIAN_POINT ( 'NONE',  ( 2.798362969681366330, 33.99680007765648071, -2.102939460078824929 ) ) ;
#8395=CARTESIAN_POINT ( 'NONE',  ( 3.500000000000000444, 36.74680007765648071, -0.05647727720536935281 ) ) ;
#8401=CARTESIAN_POINT ( 'NONE',  ( -2.829195390882805139, 18.37180007765647360, -3.793023760679206102 ) ) ;
#8404=CARTESIAN_POINT ( 'NONE',  ( 2.518350579753611207, 35.62819992234354771, -0.7558219633769606149 ) ) ;
#8408=CARTESIAN_POINT ( 'NONE',  ( 3.673772985318219053, 36.99680007765647360, 2.599342558260951730 ) ) ;
#8422=CARTESIAN_POINT ( 'NONE',  ( 4.481649420246397675, 20.87819992234354416, 1.518615910253363177 ) ) ;
#8423=CARTESIAN_POINT ( 'NONE',  ( 1.135272562821020070, 22.75319992234354416, -3.311245368580577164 ) ) ;
#8425=CARTESIAN_POINT ( 'NONE',  ( 0.8262555684461332373, 37.24680007765648071, 2.360188852285403982 ) ) ;
#8426=CARTESIAN_POINT ( 'NONE',  ( -4.518350579753602325, 36.87819992234354061, 1.405661355842794391 ) ) ;
#8430=CARTESIAN_POINT ( 'NONE',  ( -2.211161402132902243, 18.37180007765647005, -2.942372952327172886 ) ) ;
#8433=CARTESIAN_POINT ( 'NONE',  ( 3.673772985318219053, 21.99680007765647716, 2.599342558260951730 ) ) ;
#8438=CARTESIAN_POINT ( 'NONE',  ( 2.864755990943265829, 26.99680007765648071, 2.011557305968487697 ) ) ;
#8442=CARTESIAN_POINT ( 'NONE',  ( 3.518350579753605434, 20.62819992234354771, -1.080741659609877114 ) ) ;
#8444=CARTESIAN_POINT ( 'NONE',  ( -3.481649420246369697, 35.37180007765648071, 1.193696214020542490 ) ) ;
#8445=CARTESIAN_POINT ( 'NONE',  ( 2.798362969681409851, 28.50319992234354416, 2.102939460078764977 ) ) ;
#8458=CARTESIAN_POINT ( 'NONE',  ( -1.593127413382952939, 19.12819992234354771, 2.091722143975172532 ) ) ;
#8462=CARTESIAN_POINT ( 'NONE',  ( 2.115076519116362963, 38.87180007765645939, -3.012182706137107591 ) ) ;
#8466=CARTESIAN_POINT ( 'NONE',  ( -2.864755990943265829, 30.74680007765647716, -2.011557305968488141 ) ) ;
#8477=CARTESIAN_POINT ( 'NONE',  ( -2.115076519116362519, 40.12180007765648071, 3.012182706137107147 ) ) ;
#8484=CARTESIAN_POINT ( 'NONE',  ( -1.989345975306457071, 32.25319992234354061, -1.515154207786300944 ) ) ;
#8487=CARTESIAN_POINT ( 'NONE',  ( 4.518350579753633411, 36.87180007765647360, 1.405661355842698468 ) ) ;
#8504=CARTESIAN_POINT ( 'NONE',  ( 1.444289557195957086, 15.25319992234354594, -4.262301884875733471 ) ) ;
#8505=CARTESIAN_POINT ( 'NONE',  ( 1.027846397803612311, 28.75319992234354416, 3.346150245485499219 ) ) ;
#8507=CARTESIAN_POINT ( 'NONE',  ( -1.989345975306457071, 14.75319992234354771, -1.515154207786300944 ) ) ;
#8509=CARTESIAN_POINT ( 'NONE',  ( -3.607379964056363075, 34.75319992234354771, -2.690724712371229899 ) ) ;
#8516=CARTESIAN_POINT ( 'NONE',  ( -1.027846397803541700, 22.49680007765648071, 3.346150245485522312 ) ) ;
#8520=CARTESIAN_POINT ( 'NONE',  ( -1.444289557196047014, 20.99680007765647360, -4.262301884875704161 ) ) ;
#8527=CARTESIAN_POINT ( 'NONE',  ( 2.115076519116362963, 23.87180007765647005, -3.012182706137107147 ) ) ;
#8533=CARTESIAN_POINT ( 'NONE',  ( 2.798362969681409851, 18.50319992234354771, 2.102939460078764977 ) ) ;
#8535=CARTESIAN_POINT ( 'NONE',  ( 2.864755990943265829, 39.49680007765647360, 2.011557305968487697 ) ) ;
#8536=CARTESIAN_POINT ( 'NONE',  ( 1.027846397803612311, 33.75319992234354771, 3.346150245485499219 ) ) ;
#8546=CARTESIAN_POINT ( 'NONE',  ( -2.900082530493758526, 15.00000000000002309, -0.8289172060808163156 ) ) ;
#8550=CARTESIAN_POINT ( 'NONE',  ( 2.518350579753611207, 18.12819992234354416, -0.7558219633769606149 ) ) ;
#8552=CARTESIAN_POINT ( 'NONE',  ( -0.05938372350927861171, 18.62180007765647005, -3.680117784833935701 ) ) ;
#8557=CARTESIAN_POINT ( 'NONE',  ( -2.798362969681365886, 35.24680007765648071, 2.102939460078824929 ) ) ;
#8571=CARTESIAN_POINT ( 'NONE',  ( -2.055738996568313048, 23.24680007765648071, -1.423772053676023441 ) ) ;
#8573=CARTESIAN_POINT ( 'NONE',  ( -2.211161402132901799, 20.87180007765647360, -2.942372952327172886 ) ) ;
#8578=CARTESIAN_POINT ( 'NONE',  ( -3.481649420246394122, 14.62819992234354061, -1.193696214020467883 ) ) ;
#8581=CARTESIAN_POINT ( 'NONE',  ( 2.829195390882805583, 29.62180007765647005, 3.793023760679204770 ) ) ;
#8596=CARTESIAN_POINT ( 'NONE',  ( 3.607379964056363075, 21.00319992234354416, 2.690724712371229010 ) ) ;
#8597=CARTESIAN_POINT ( 'NONE',  ( -0.05938372350920064630, 26.37819992234354416, 3.680117784833935701 ) ) ;
#8598=CARTESIAN_POINT ( 'NONE',  ( 2.055738996568313048, 34.49680007765648071, 1.423772053676023441 ) ) ;
#8600=CARTESIAN_POINT ( 'NONE',  ( 2.733110507866328920, 33.62819992234354771, 3.862833514489095510 ) ) ;
#8604=CARTESIAN_POINT ( 'NONE',  ( -0.05938372350927861171, 28.62180007765648071, -3.680117784833935701 ) ) ;
#8607=CARTESIAN_POINT ( 'NONE',  ( 2.829195390882805583, 34.62180007765646650, 3.793023760679204770 ) ) ;
#8612=CARTESIAN_POINT ( 'NONE',  ( 2.211161402132902243, 27.12180007765647360, 2.942372952327172442 ) ) ;
#8619=CARTESIAN_POINT ( 'NONE',  ( -2.211161402132839182, 19.12819992234353705, 2.942372952327218627 ) ) ;
#8622=CARTESIAN_POINT ( 'NONE',  ( 3.518350579753631191, 36.87180007765645939, 1.080741659609802285 ) ) ;
#8624=CARTESIAN_POINT ( 'NONE',  ( 2.115076519116426024, 38.62819992234354771, 3.012182706137062294 ) ) ;
#8640=CARTESIAN_POINT ( 'NONE',  ( -2.481649420246391902, 19.62819992234354416, -0.8687765177875723666 ) ) ;
#8648=CARTESIAN_POINT ( 'NONE',  ( -1.135272562821090014, 30.99680007765647716, -3.311245368580554072 ) ) ;
#8660=CARTESIAN_POINT ( 'NONE',  ( 0.7188294034286049072, 18.74680007765648071, -2.395093729190366005 ) ) ;
#8662=CARTESIAN_POINT ( 'NONE',  ( -3.518350579753630303, 25.62180007765647716, -1.080741659609802952 ) ) ;
#8666=CARTESIAN_POINT ( 'NONE',  ( 1.593127413382953383, 37.87819992234354771, -2.091722143975172532 ) ) ;
#8669=CARTESIAN_POINT ( 'NONE',  ( -4.518350579753632523, 35.62180007765647360, -1.405661355842698468 ) ) ;
#8687=CARTESIAN_POINT ( 'NONE',  ( -2.733110507866328476, 19.87819992234354416, -3.862833514489096398 ) ) ;
#8688=CARTESIAN_POINT ( 'NONE',  ( 3.518350579753606322, 25.62819992234354416, -1.080741659609876892 ) ) ;
#8690=CARTESIAN_POINT ( 'NONE',  ( 0.8262555684460829442, 15.25319992234354771, -2.360188852285421302 ) ) ;
#8692=CARTESIAN_POINT ( 'NONE',  ( 3.607379964056363075, 36.00319992234354771, 2.690724712371229010 ) ) ;
#8697=CARTESIAN_POINT ( 'NONE',  ( 3.500000000000000444, 29.24680007765647716, -0.05647727720536935281 ) ) ;
#8701=CARTESIAN_POINT ( 'NONE',  ( -2.829195390882805139, 28.37180007765647716, -3.793023760679206102 ) ) ;
#8705=CARTESIAN_POINT ( 'NONE',  ( 2.864755990943265829, 24.49680007765647716, 2.011557305968487697 ) ) ;
#8712=CARTESIAN_POINT ( 'NONE',  ( -2.211161402132839182, 16.62819992234354416, 2.942372952327218627 ) ) ;
#8715=CARTESIAN_POINT ( 'NONE',  ( 2.518350579753628971, 16.87180007765648071, 0.7558219633769073242 ) ) ;
#8716=CARTESIAN_POINT ( 'NONE',  ( 3.518350579753605434, 35.62819992234353350, -1.080741659609877114 ) ) ;
#8731=CARTESIAN_POINT ( 'NONE',  ( 2.055738996568281518, 20.50319992234355126, -1.423772053676066518 ) ) ;
#8734=CARTESIAN_POINT ( 'NONE',  ( -4.499999999999999112, 39.50319992234354061, -0.05647727720528529505 ) ) ;
#8739=CARTESIAN_POINT ( 'NONE',  ( -3.481649420246369697, 37.87180007765648071, 1.193696214020542490 ) ) ;
#8754=CARTESIAN_POINT ( 'NONE',  ( 1.593127413382998903, 19.62180007765648071, 2.091722143975139669 ) ) ;
#8756=CARTESIAN_POINT ( 'NONE',  ( -2.798362969681365886, 20.24680007765647716, 2.102939460078824929 ) ) ;
#8761=CARTESIAN_POINT ( 'NONE',  ( -3.518350579753605434, 21.87819992234354771, 1.080741659609877781 ) ) ;
#8764=CARTESIAN_POINT ( 'NONE',  ( -1.336863392178478716, 34.99680007765647360, 4.297206761780677731 ) ) ;
#8782=CARTESIAN_POINT ( 'NONE',  ( 3.607379964056363075, 23.50319992234354416, 2.690724712371229010 ) ) ;
#8783=CARTESIAN_POINT ( 'NONE',  ( 2.864755990943222308, 30.50319992234354416, -2.011557305968548093 ) ) ;
#8784=CARTESIAN_POINT ( 'NONE',  ( 2.481649420246374138, 36.62180007765647360, -0.8687765177876252132 ) ) ;
#8786=CARTESIAN_POINT ( 'NONE',  ( 3.673772985318163098, 33.00319992234354771, -2.599342558261029001 ) ) ;
#8793=CARTESIAN_POINT ( 'NONE',  ( 0.05938372350927906274, 27.37180007765647716, 3.680117784833935701 ) ) ;
#8798=CARTESIAN_POINT ( 'NONE',  ( -1.444289557196047014, 30.99680007765647716, -4.262301884875704161 ) ) ;
#8802=CARTESIAN_POINT ( 'NONE',  ( -1.135272562821090014, 28.49680007765648071, -3.311245368580554072 ) ) ;
#8808=CARTESIAN_POINT ( 'NONE',  ( 3.518350579753605434, 23.12819992234354416, -1.080741659609877114 ) ) ;
#8812=CARTESIAN_POINT ( 'NONE',  ( -2.500000000000001332, 17.99680007765648071, 0.05647727720535858364 ) ) ;
#8813=CARTESIAN_POINT ( 'NONE',  ( -2.798362969681409851, 37.25319992234354061, -2.102939460078765421 ) ) ;
#8831=CARTESIAN_POINT ( 'NONE',  ( -0.8262555684460826111, 24.00319992234354416, 2.360188852285421302 ) ) ;
#8833=CARTESIAN_POINT ( 'NONE',  ( 2.211161402132902243, 17.12180007765648071, 2.942372952327172442 ) ) ;
#8839=CARTESIAN_POINT ( 'NONE',  ( -3.481649420246369697, 40.37180007765648071, 1.193696214020542490 ) ) ;
#8849=CARTESIAN_POINT ( 'NONE',  ( 1.497042530366477164, 18.87180007765648071, -2.161531897785062384 ) ) ;
#8851=CARTESIAN_POINT ( 'NONE',  ( 2.115076519116362963, 21.37180007765647716, -3.012182706137107591 ) ) ;
#8858=CARTESIAN_POINT ( 'NONE',  ( 3.500000000000000444, 20.75319992234354416, 0.05647727720529520379 ) ) ;
#8863=CARTESIAN_POINT ( 'NONE',  ( 3.518350579753631191, 16.87180007765648071, 1.080741659609802285 ) ) ;
#8882=CARTESIAN_POINT ( 'NONE',  ( 4.518350579753602325, 25.62819992234354416, -1.405661355842793725 ) ) ;
#8883=CARTESIAN_POINT ( 'NONE',  ( 2.864755990943222308, 28.00319992234354416, -2.011557305968548093 ) ) ;
#8884=CARTESIAN_POINT ( 'NONE',  ( 1.989345975306457071, 23.50319992234355126, 1.515154207786300500 ) ) ;
#8886=CARTESIAN_POINT ( 'NONE',  ( -1.336863392178478716, 17.49680007765647716, 4.297206761780677731 ) ) ;
#8891=CARTESIAN_POINT ( 'NONE',  ( 1.027846397803542144, 31.24680007765647716, -3.346150245485522312 ) ) ;
#8895=CARTESIAN_POINT ( 'NONE',  ( 0.05938372350929014415, 29.87180007765647005, 4.731580009072201776 ) ) ;
#8897=CARTESIAN_POINT ( 'NONE',  ( -1.027846397803541700, 32.49680007765648071, 3.346150245485522312 ) ) ;
#8904=CARTESIAN_POINT ( 'NONE',  ( -3.481649420246394122, 29.62819992234353350, -1.193696214020467883 ) ) ;
#8907=CARTESIAN_POINT ( 'NONE',  ( -0.7188294034286043521, 24.99680007765647716, 2.395093729190366005 ) ) ;
#8910=CARTESIAN_POINT ( 'NONE',  ( 3.500000000000000444, 33.25319992234354771, 0.05647727720529520379 ) ) ;
#8923=CARTESIAN_POINT ( 'NONE',  ( -1.497042530366522461, 29.87819992234354416, -2.161531897785030409 ) ) ;
#8946=CARTESIAN_POINT ( 'NONE',  ( 0.8262555684461332373, 24.74680007765647716, 2.360188852285403982 ) ) ;
#8948=CARTESIAN_POINT ( 'NONE',  ( 2.864755990943265829, 24.49680007765647716, 2.011557305968487697 ) ) ;
#8955=CARTESIAN_POINT ( 'NONE',  ( 0.05938372350920109732, 15.12819992234354238, -3.680117784833935701 ) ) ;
#8958=CARTESIAN_POINT ( 'NONE',  ( -2.733110507866247652, 37.62180007765646650, 3.862833514489154574 ) ) ;
#8981=SHAPE_REPRESENTATION_RELATIONSHIP ( 'NONE' , 'NONE' ,  #5199, #9153 ) ;
#8983=CARTESIAN_POINT ( 'NONE',  ( -0.05938372350918959958, 26.37819992234355126, 4.731580009072201776 ) ) ;
#8984=CARTESIAN_POINT ( 'NONE',  ( -2.864755990943222308, 36.75319992234354061, 2.011557305968548093 ) ) ;
#8985=CARTESIAN_POINT ( 'NONE',  ( -2.055738996568281518, 16.75319992234354416, 1.423772053676066962 ) ) ;
#8988=CARTESIAN_POINT ( 'NONE',  ( -4.499999999999999112, 39.50319992234354061, -0.05647727720528529505 ) ) ;
#8993=CARTESIAN_POINT ( 'NONE',  ( 0.05938372350927906274, 32.37180007765647360, 3.680117784833935701 ) ) ;
#8997=CARTESIAN_POINT ( 'NONE',  ( -4.499999999999999112, 30.49680007765648071, 0.05647727720537927543 ) ) ;
#9000=CARTESIAN_POINT ( 'NONE',  ( 1.135272562821090458, 29.74680007765647716, 3.311245368580554072 ) ) ;
#9006=CARTESIAN_POINT ( 'NONE',  ( 2.211161402132839626, 27.87819992234354061, -2.942372952327218183 ) ) ;
#9009=CARTESIAN_POINT ( 'NONE',  ( 1.593127413382998903, 19.62180007765648071, 2.091722143975139669 ) ) ;
#9010=CARTESIAN_POINT ( 'NONE',  ( 1.444289557195957086, 15.25319992234354594, -4.262301884875733471 ) ) ;
#9023=CARTESIAN_POINT ( 'NONE',  ( 1.497042530366522461, 26.12819992234354416, 2.161531897785029965 ) ) ;
#9024=CARTESIAN_POINT ( 'NONE',  ( 0.000000000000000000, 0.000000000000000000, 0.000000000000000000 ) ) ;
#9026=CARTESIAN_POINT ( 'NONE',  ( -2.211161402132902243, 20.87180007765647716, -2.942372952327172886 ) ) ;
#9042=CARTESIAN_POINT ( 'NONE',  ( -0.7188294034286043521, 32.49680007765648782, 2.395093729190366005 ) ) ;
#9044=CARTESIAN_POINT ( 'NONE',  ( 3.500000000000000444, 26.74680007765648071, -0.05647727720536935281 ) ) ;
#9049=CARTESIAN_POINT ( 'NONE',  ( -1.027846397803611866, 20.00319992234354416, -3.346150245485499219 ) ) ;
#9052=CARTESIAN_POINT ( 'NONE',  ( 3.607379964056306676, 38.99680007765648071, -2.690724712371305838 ) ) ;
#9070=CARTESIAN_POINT ( 'NONE',  ( 4.481649420246397675, 25.87819992234355126, 1.518615910253363177 ) ) ;
#9071=CARTESIAN_POINT ( 'NONE',  ( -1.135272562821019626, 34.00319992234354771, 3.311245368580577164 ) ) ;
#9072=CARTESIAN_POINT ( 'NONE',  ( 2.500000000000001332, 20.75319992234354771, 0.05647727720530566764 ) ) ;
#9074=CARTESIAN_POINT ( 'NONE',  ( -2.733110507866247652, 20.12180007765647716, 3.862833514489154574 ) ) ;
#9091=CARTESIAN_POINT ( 'NONE',  ( -0.05938372350920063936, 26.37819992234354061, 3.680117784833935701 ) ) ;
#9094=CARTESIAN_POINT ( 'NONE',  ( -2.055738996568313048, 23.24680007765648071, -1.423772053676023441 ) ) ;
#9096=CARTESIAN_POINT ( 'NONE',  ( 2.733110507866328920, 21.12819992234354416, 3.862833514489095510 ) ) ;
#9116=CARTESIAN_POINT ( 'NONE',  ( -2.481649420246391902, 24.62819992234354416, -0.8687765177875723666 ) ) ;
#9118=CARTESIAN_POINT ( 'NONE',  ( 3.481649420246369697, 21.62180007765647360, -1.193696214020541824 ) ) ;
#9132=DIRECTION ( 'NONE',  ( 0.000000000000000000, 0.9936001553129349961, 0.1129545544106631688 ) ) ;
#9133=CARTESIAN_POINT ( 'NONE',  ( -0.8262555684461330152, 28.49680007765648071, -2.360188852285403982 ) ) ;
#9136=CARTESIAN_POINT ( 'NONE',  ( 1.135272562821090458, 27.24680007765648071, 3.311245368580554072 ) ) ;
#9139=CARTESIAN_POINT ( 'NONE',  ( -2.115076519116425580, 22.37819992234353350, -3.012182706137062738 ) ) ;
#9144=CARTESIAN_POINT ( 'NONE',  ( 2.864755990943265829, 19.49680007765648071, 2.011557305968487697 ) ) ;
#9153=ADVANCED_BREP_SHAPE_REPRESENTATION ( '', ( #14305, #16940 ), #6566 ) ;
#9164=CARTESIAN_POINT ( 'NONE',  ( -4.518350579753602325, 26.87819992234354416, 1.405661355842794391 ) ) ;
#9165=CARTESIAN_POINT ( 'NONE',  ( 1.027846397803612311, 36.25319992234354771, 3.346150245485499219 ) ) ;
#9167=CARTESIAN_POINT ( 'NONE',  ( -2.518350579753611207, 16.87819992234354416, 0.7558219633769609480 ) ) ;
#9169=CARTESIAN_POINT ( 'NONE',  ( 4.499999999999999112, 19.24680007765647716, -0.05647727720537982360 ) ) ;
#9174=CARTESIAN_POINT ( 'NONE',  ( -3.481649420246369697, 40.37180007765648071, 1.193696214020542490 ) ) ;
#9186=CARTESIAN_POINT ( 'NONE',  ( 2.864755990943222308, 28.00319992234354416, -2.011557305968548093 ) ) ;
#9189=CARTESIAN_POINT ( 'NONE',  ( -0.05938372350926768989, 21.12180007765648426, -2.628655560595669183 ) ) ;
#9191=CARTESIAN_POINT ( 'NONE',  ( -1.444289557195956863, 16.50319992234354416, 4.262301884875733471 ) ) ;
#9195=CARTESIAN_POINT ( 'NONE',  ( 2.211161402132902243, 17.12180007765648071, 2.942372952327172442 ) ) ;
#9210=CARTESIAN_POINT ( 'NONE',  ( 1.497042530366522461, 28.62819992234355126, 2.161531897785029965 ) ) ;
#9213=CARTESIAN_POINT ( 'NONE',  ( -0.05938372350927861171, 23.62180007765647005, -3.680117784833935701 ) ) ;
#9227=CARTESIAN_POINT ( 'NONE',  ( 2.055738996568313048, 31.99680007765648426, 1.423772053676023441 ) ) ;
#9229=CARTESIAN_POINT ( 'NONE',  ( 2.798362969681366330, 26.49680007765648071, -2.102939460078824929 ) ) ;
#9236=CARTESIAN_POINT ( 'NONE',  ( 1.135272562821090458, 19.74680007765648071, 3.311245368580554072 ) ) ;
#9253=CARTESIAN_POINT ( 'NONE',  ( 3.673772985318163098, 35.50319992234354771, -2.599342558261029001 ) ) ;
#9254=CARTESIAN_POINT ( 'NONE',  ( -0.05938372350920064630, 33.87819992234354061, 3.680117784833935701 ) ) ;
#9255=CARTESIAN_POINT ( 'NONE',  ( 1.989345975306457071, 18.50319992234354416, 1.515154207786300500 ) ) ;
#9257=CARTESIAN_POINT ( 'NONE',  ( 4.518350579753633411, 19.37180007765647716, 1.405661355842698468 ) ) ;
#9263=CARTESIAN_POINT ( 'NONE',  ( -2.798362969681365886, 35.24680007765648071, 2.102939460078824929 ) ) ;
#9278=CARTESIAN_POINT ( 'NONE',  ( 1.135272562821020070, 27.75319992234354416, -3.311245368580577164 ) ) ;
#9281=CARTESIAN_POINT ( 'NONE',  ( -0.05938372350926768989, 18.62180007765648071, -2.628655560595669183 ) ) ;
#9282=CARTESIAN_POINT ( 'NONE',  ( -4.499999999999999112, 14.50319992234354594, -0.05647727720528529505 ) ) ;
#9286=CARTESIAN_POINT ( 'NONE',  ( -0.05938372350927861171, 16.12180007765647716, -3.680117784833935701 ) ) ;
#9293=CARTESIAN_POINT ( 'NONE',  ( -3.518350579753630747, 15.62180007765647538, -1.080741659609802729 ) ) ;
#9297=CARTESIAN_POINT ( 'NONE',  ( 0.05938372350921204690, 27.62819992234354416, -2.628655560595669183 ) ) ;
#9299=CARTESIAN_POINT ( 'NONE',  ( 3.518350579753631191, 26.87180007765647360, 1.080741659609802285 ) ) ;
#9308=CARTESIAN_POINT ( 'NONE',  ( -0.05938372350928957516, 21.12180007765647360, -4.731580009072201776 ) ) ;
#9316=CARTESIAN_POINT ( 'NONE',  ( -0.8262555684461330152, 33.49680007765648071, -2.360188852285403982 ) ) ;
#9318=CARTESIAN_POINT ( 'NONE',  ( -1.135272562821090014, 33.49680007765648071, -3.311245368580554072 ) ) ;
#9325=CARTESIAN_POINT ( 'NONE',  ( 1.027846397803542144, 23.74680007765647716, -3.346150245485522312 ) ) ;
#9336=CARTESIAN_POINT ( 'NONE',  ( 3.481649420246369697, 29.12180007765647005, -1.193696214020541824 ) ) ;
#9340=CARTESIAN_POINT ( 'NONE',  ( 4.499999999999999112, 35.75319992234354061, 0.05647727720528474687 ) ) ;
#9341=CARTESIAN_POINT ( 'NONE',  ( 3.481649420246395010, 33.37819992234354061, 1.193696214020467439 ) ) ;
#9342=CARTESIAN_POINT ( 'NONE',  ( -2.481649420246391902, 24.62819992234354416, -0.8687765177875723666 ) ) ;
#9344=CARTESIAN_POINT ( 'NONE',  ( 4.499999999999999112, 21.74680007765647360, -0.05647727720537982360 ) ) ;
#9349=CARTESIAN_POINT ( 'NONE',  ( -2.798362969681365886, 40.24680007765648071, 2.102939460078824929 ) ) ;
#9363=CARTESIAN_POINT ( 'NONE',  ( -2.211161402132839182, 39.12819992234354771, 2.942372952327218627 ) ) ;
#9364=CARTESIAN_POINT ( 'NONE',  ( 0.05938372350920110426, 15.12819992234354416, -3.680117784833935701 ) ) ;
#9366=CARTESIAN_POINT ( 'NONE',  ( -1.497042530366477164, 27.62180007765648426, 2.161531897785062384 ) ) ;
#9367=CARTESIAN_POINT ( 'NONE',  ( 3.607379964056363075, 18.50319992234354416, 2.690724712371229010 ) ) ;
#9373=CARTESIAN_POINT ( 'NONE',  ( -2.733110507866247652, 40.12180007765647360, 3.862833514489154574 ) ) ;
#9384=CARTESIAN_POINT ( 'NONE',  ( 0.8262555684460829442, 35.25319992234354771, -2.360188852285421302 ) ) ;
#9387=CARTESIAN_POINT ( 'NONE',  ( -3.500000000000000444, 22.99680007765647716, 0.05647727720536892260 ) ) ;
#9394=CARTESIAN_POINT ( 'NONE',  ( 3.673772985318219053, 24.49680007765648071, 2.599342558260951730 ) ) ;
#9401=CARTESIAN_POINT ( 'NONE',  ( -1.989345975306426206, 30.24680007765648426, 1.515154207786343799 ) ) ;
#9403=CARTESIAN_POINT ( 'NONE',  ( -3.500000000000000444, 27.99680007765648071, 0.05647727720536892260 ) ) ;
#9411=CARTESIAN_POINT ( 'NONE',  ( -2.115076519116362519, 27.62180007765648071, 3.012182706137107147 ) ) ;
#9425=CARTESIAN_POINT ( 'NONE',  ( -3.500000000000000444, 30.49680007765647716, 0.05647727720536892260 ) ) ;
#9431=CARTESIAN_POINT ( 'NONE',  ( -0.05938372350918959958, 33.87819992234354061, 4.731580009072201776 ) ) ;
#9433=CARTESIAN_POINT ( 'NONE',  ( -2.518350579753611207, 26.87819992234354416, 0.7558219633769609480 ) ) ;
#9437=CARTESIAN_POINT ( 'NONE',  ( -2.829195390882805139, 25.87180007765647716, -3.793023760679206102 ) ) ;
#9441=CARTESIAN_POINT ( 'NONE',  ( 3.518350579753631191, 39.37180007765646650, 1.080741659609802285 ) ) ;
#9453=CARTESIAN_POINT ( 'NONE',  ( 1.135272562821090458, 17.24680007765647716, 3.311245368580554072 ) ) ;
#9456=CARTESIAN_POINT ( 'NONE',  ( -1.027846397803611866, 32.50319992234354771, -3.346150245485499219 ) ) ;
#9457=CARTESIAN_POINT ( 'NONE',  ( -0.05938372350920064630, 16.37819992234354416, 3.680117784833935701 ) ) ;
#9459=CARTESIAN_POINT ( 'NONE',  ( -2.500000000000001332, 32.99680007765648071, 0.05647727720535858364 ) ) ;
#9460=CARTESIAN_POINT ( 'NONE',  ( 1.444289557195957086, 22.75319992234354061, -4.262301884875733471 ) ) ;
#9466=CARTESIAN_POINT ( 'NONE',  ( 4.518350579753633411, 36.87180007765647360, 1.405661355842698468 ) ) ;
#9477=CARTESIAN_POINT ( 'NONE',  ( 1.135272562821020070, 15.25319992234354594, -3.311245368580577164 ) ) ;
#9479=CARTESIAN_POINT ( 'NONE',  ( -2.115076519116362519, 30.12180007765647360, 3.012182706137107147 ) ) ;
#9480=CARTESIAN_POINT ( 'NONE',  ( 3.500000000000000444, 28.25319992234354416, 0.05647727720529520379 ) ) ;
#9486=CARTESIAN_POINT ( 'NONE',  ( 2.733110507866247652, 21.37180007765647360, -3.862833514489153686 ) ) ;
#9493=CARTESIAN_POINT ( 'NONE',  ( -2.518350579753628526, 38.12180007765647360, -0.7558219633769075463 ) ) ;
#9496=CARTESIAN_POINT ( 'NONE',  ( -3.518350579753630303, 38.12180007765647360, -1.080741659609802952 ) ) ;
#9503=CARTESIAN_POINT ( 'NONE',  ( -2.798362969681365886, 22.74680007765648071, 2.102939460078824929 ) ) ;
#9515=CARTESIAN_POINT ( 'NONE',  ( 2.864755990943265829, 39.49680007765647360, 2.011557305968487697 ) ) ;
#9517=VERTEX_POINT ( 'NONE', #8027 ) ;
#9520=CARTESIAN_POINT ( 'NONE',  ( 2.829195390882724759, 37.87819992234353350, -3.793023760679264278 ) ) ;
#9523=CARTESIAN_POINT ( 'NONE',  ( -2.500000000000001332, 29.50319992234354771, -0.05647727720530596601 ) ) ;
#9527=CARTESIAN_POINT ( 'NONE',  ( -3.673772985318219053, 23.24680007765647716, -2.599342558260952174 ) ) ;
#9543=CARTESIAN_POINT ( 'NONE',  ( -0.05938372350927861865, 16.12180007765647716, -3.680117784833935701 ) ) ;
#9545=CARTESIAN_POINT ( 'NONE',  ( 2.798362969681409851, 33.50319992234354771, 2.102939460078764977 ) ) ;
#9546=CARTESIAN_POINT ( 'NONE',  ( 2.115076519116425580, 23.62819992234354061, 3.012182706137062294 ) ) ;
#9548=CARTESIAN_POINT ( 'NONE',  ( 0.7188294034286049072, 28.74680007765648426, -2.395093729190366005 ) ) ;
#9550=CARTESIAN_POINT ( 'NONE',  ( -2.829195390882724315, 29.12819992234354416, 3.793023760679264722 ) ) ;
#9558=CARTESIAN_POINT ( 'NONE',  ( -2.798362969681365886, 25.24680007765647716, 2.102939460078824929 ) ) ;
#9568=CARTESIAN_POINT ( 'NONE',  ( 1.135272562821090458, 17.24680007765647716, 3.311245368580554072 ) ) ;
#9572=CARTESIAN_POINT ( 'NONE',  ( 0.7188294034286553114, 36.25319992234354771, 2.395093729190349130 ) ) ;
#9574=CARTESIAN_POINT ( 'NONE',  ( -2.115076519116362519, 27.62180007765648071, 3.012182706137107147 ) ) ;
#9575=CARTESIAN_POINT ( 'NONE',  ( 0.05938372350920109732, 25.12819992234354416, -3.680117784833935701 ) ) ;
#9581=CARTESIAN_POINT ( 'NONE',  ( 2.733110507866247652, 23.87180007765647716, -3.862833514489153686 ) ) ;
#9588=CARTESIAN_POINT ( 'NONE',  ( -2.500000000000001332, 35.49680007765647360, 0.05647727720535858364 ) ) ;
#9591=CARTESIAN_POINT ( 'NONE',  ( -0.05938372350927861865, 38.62180007765647360, -3.680117784833935701 ) ) ;
#9595=CARTESIAN_POINT ( 'NONE',  ( -1.860401164264412488, 15.00000000000001243, -3.294166817225182786 ) ) ;
#9599=CARTESIAN_POINT ( 'NONE',  ( -3.518350579753630747, 28.12180007765647360, -1.080741659609802729 ) ) ;
#9612=CARTESIAN_POINT ( 'NONE',  ( 3.500000000000000444, 39.24680007765647360, -0.05647727720536935281 ) ) ;
#9615=CARTESIAN_POINT ( 'NONE',  ( 4.518350579753602325, 38.12819992234354061, -1.405661355842793725 ) ) ;
#9617=CARTESIAN_POINT ( 'NONE',  ( -0.8262555684460826111, 24.00319992234354416, 2.360188852285421302 ) ) ;
#9620=CARTESIAN_POINT ( 'NONE',  ( 2.829195390882805583, 27.12180007765647716, 3.793023760679204770 ) ) ;
#9634=CARTESIAN_POINT ( 'NONE',  ( -0.05938372350920063936, 36.37819992234355482, 3.680117784833935701 ) ) ;
#9635=CARTESIAN_POINT ( 'NONE',  ( 1.135272562821020070, 20.25319992234354416, -3.311245368580577164 ) ) ;
#9637=CARTESIAN_POINT ( 'NONE',  ( 0.7188294034286049072, 33.74680007765648071, -2.395093729190366005 ) ) ;
#9639=CARTESIAN_POINT ( 'NONE',  ( -3.607379964056363075, 22.25319992234354416, -2.690724712371229899 ) ) ;
#9643=CARTESIAN_POINT ( 'NONE',  ( -3.518350579753630747, 18.12180007765648071, -1.080741659609802729 ) ) ;
#9656=CARTESIAN_POINT ( 'NONE',  ( -1.497042530366522461, 37.37819992234354771, -2.161531897785030409 ) ) ;
#9659=CARTESIAN_POINT ( 'NONE',  ( -2.115076519116362519, 32.62180007765646650, 3.012182706137107147 ) ) ;
#9661=CARTESIAN_POINT ( 'NONE',  ( -3.481649420246394122, 27.12819992234354771, -1.193696214020467883 ) ) ;
#9674=CARTESIAN_POINT ( 'NONE',  ( 2.500000000000001332, 36.74680007765648071, -0.05647727720535888202 ) ) ;
#9676=CARTESIAN_POINT ( 'NONE',  ( 2.211161402132902243, 34.62180007765648071, 2.942372952327172442 ) ) ;
#9681=CARTESIAN_POINT ( 'NONE',  ( -1.135272562821090014, 20.99680007765647716, -3.311245368580554072 ) ) ;
#9694=CARTESIAN_POINT ( 'NONE',  ( -2.211161402132902243, 35.87180007765648782, -2.942372952327172886 ) ) ;
#9697=CARTESIAN_POINT ( 'NONE',  ( -2.829195390882805139, 15.87180007765647716, -3.793023760679206102 ) ) ;
#9700=CARTESIAN_POINT ( 'NONE',  ( 0.05938372350921204690, 25.12819992234354416, -2.628655560595669183 ) ) ;
#9704=CARTESIAN_POINT ( 'NONE',  ( -2.829195390882805139, 28.37180007765647716, -3.793023760679206102 ) ) ;
#9719=CARTESIAN_POINT ( 'NONE',  ( -0.05938372350927861865, 23.62180007765647360, -3.680117784833935701 ) ) ;
#9724=CARTESIAN_POINT ( 'NONE',  ( -2.864755990943222308, 31.75319992234354416, 2.011557305968548093 ) ) ;
#9725=CARTESIAN_POINT ( 'NONE',  ( 3.518350579753606322, 20.62819992234354416, -1.080741659609876892 ) ) ;
#9729=CARTESIAN_POINT ( 'NONE',  ( -2.481649420246374138, 27.87180007765648426, 0.8687765177876256573 ) ) ;
#9730=CARTESIAN_POINT ( 'NONE',  ( -4.481649420246396787, 29.62819992234354416, -1.518615910253363399 ) ) ;
#9731=UNCERTAINTY_MEASURE_WITH_UNIT (LENGTH_MEASURE( 1.000000000000000082E-05 ), #7022, 'distance_accuracy_value', 'NONE');
#9735=CARTESIAN_POINT ( 'NONE',  ( -2.798362969681365886, 22.74680007765648071, 2.102939460078824929 ) ) ;
#9745=CARTESIAN_POINT ( 'NONE',  ( 2.798362969681366330, 21.49680007765647716, -2.102939460078824929 ) ) ;
#9750=CARTESIAN_POINT ( 'NONE',  ( 2.481649420246391902, 33.37819992234354771, 0.8687765177875720335 ) ) ;
#9753=CARTESIAN_POINT ( 'NONE',  ( -2.798362969681365886, 30.24680007765648071, 2.102939460078824929 ) ) ;
#9755=CARTESIAN_POINT ( 'NONE',  ( 2.211161402132839626, 30.37819992234354416, -2.942372952327218183 ) ) ;
#9770=CARTESIAN_POINT ( 'NONE',  ( -2.481649420246374138, 40.37180007765647360, 0.8687765177876256573 ) ) ;
#9772=CARTESIAN_POINT ( 'NONE',  ( -2.115076519116362519, 40.12180007765648071, 3.012182706137108035 ) ) ;
#9779=CARTESIAN_POINT ( 'NONE',  ( 2.798362969681366330, 28.99680007765647716, -2.102939460078824929 ) ) ;
#9789=CARTESIAN_POINT ( 'NONE',  ( 2.500000000000001332, 16.74680007765648071, -0.05647727720535888202 ) ) ;
#9794=CARTESIAN_POINT ( 'NONE',  ( 2.733110507866328920, 38.62819992234354771, 3.862833514489095510 ) ) ;
#9796=CARTESIAN_POINT ( 'NONE',  ( -2.500000000000001332, 32.00319992234354061, -0.05647727720530596601 ) ) ;
#9799=CARTESIAN_POINT ( 'NONE',  ( -1.336863392178478716, 29.99680007765647716, 4.297206761780677731 ) ) ;
#9813=CARTESIAN_POINT ( 'NONE',  ( -3.500000000000000444, 39.50319992234354771, -0.05647727720529563400 ) ) ;
#9814=CARTESIAN_POINT ( 'NONE',  ( 1.027846397803612311, 21.25319992234354416, 3.346150245485499219 ) ) ;
#9816=CARTESIAN_POINT ( 'NONE',  ( 0.8262555684461332373, 34.74680007765647360, 2.360188852285403982 ) ) ;
#9817=CARTESIAN_POINT ( 'NONE',  ( 4.481649420246397675, 23.37819992234354416, 1.518615910253363177 ) ) ;
#9820=ADVANCED_FACE ( 'NONE', ( #5615 ), #8303, .F. ) ;
#9823=CARTESIAN_POINT ( 'NONE',  ( 1.027846397803542144, 18.74680007765648071, -3.346150245485522312 ) ) ;
#9834=CARTESIAN_POINT ( 'NONE',  ( -2.115076519116362519, 20.12180007765648071, 3.012182706137107147 ) ) ;
#9841=CARTESIAN_POINT ( 'NONE',  ( -2.864755990943222308, 16.75319992234354416, 2.011557305968548093 ) ) ;
#9843=CARTESIAN_POINT ( 'NONE',  ( -0.05938372350927861171, 33.62180007765648071, -3.680117784833935701 ) ) ;
#9845=CARTESIAN_POINT ( 'NONE',  ( -2.211161402132839182, 24.12819992234354416, 2.942372952327218627 ) ) ;
#9857=CARTESIAN_POINT ( 'NONE',  ( 0.05938372350921204690, 17.62819992234354416, -2.628655560595669183 ) ) ;
#9865=CARTESIAN_POINT ( 'NONE',  ( -2.864755990943265829, 35.74680007765648071, -2.011557305968488141 ) ) ;
#9876=CARTESIAN_POINT ( 'NONE',  ( -0.8262555684461330152, 15.99680007765648249, -2.360188852285403982 ) ) ;
#9884=CARTESIAN_POINT ( 'NONE',  ( -1.497042530366522461, 32.37819992234353350, -2.161531897785030409 ) ) ;
#9887=CARTESIAN_POINT ( 'NONE',  ( -3.607379964056306676, 32.74680007765648071, 2.690724712371306282 ) ) ;
#9902=CARTESIAN_POINT ( 'NONE',  ( -1.336863392178569088, 20.00319992234354416, -4.297206761780648421 ) ) ;
#9903=CARTESIAN_POINT ( 'NONE',  ( -3.518350579753606322, 24.37819992234354061, 1.080741659609877781 ) ) ;
#9905=CARTESIAN_POINT ( 'NONE',  ( -0.7188294034286550893, 15.00319992234354594, -2.395093729190349130 ) ) ;
#9906=CARTESIAN_POINT ( 'NONE',  ( -3.607379964056363075, 29.75319992234354416, -2.690724712371229899 ) ) ;
#9911=CARTESIAN_POINT ( 'NONE',  ( 1.135272562821090458, 22.24680007765648071, 3.311245368580554072 ) ) ;
#9914=CARTESIAN_POINT ( 'NONE',  ( 4.481649420246366589, 24.12180007765647716, -1.518615910253458212 ) ) ;
#9919=CARTESIAN_POINT ( 'NONE',  ( -0.05938372350927861171, 21.12180007765648071, -3.680117784833935701 ) ) ;
#9925=CARTESIAN_POINT ( 'NONE',  ( -1.027846397803611866, 22.50319992234354416, -3.346150245485499219 ) ) ;
#9928=CARTESIAN_POINT ( 'NONE',  ( 2.500000000000001332, 16.74680007765648071, -0.05647727720535888202 ) ) ;
#9930=CARTESIAN_POINT ( 'NONE',  ( -1.135272562821019626, 31.50319992234354416, 3.311245368580577164 ) ) ;
#9943=CARTESIAN_POINT ( 'NONE',  ( 0.7188294034286553114, 23.75319992234354771, 2.395093729190349130 ) ) ;
#9951=CARTESIAN_POINT ( 'NONE',  ( -1.027846397803541700, 32.49680007765648071, 3.346150245485522312 ) ) ;
#9962=CARTESIAN_POINT ( 'NONE',  ( -0.8262555684461330152, 20.99680007765648071, -2.360188852285403982 ) ) ;
#9967=CARTESIAN_POINT ( 'NONE',  ( 2.481649420246391902, 38.37819992234354061, 0.8687765177875720335 ) ) ;
#9970=CARTESIAN_POINT ( 'NONE',  ( 1.336863392178479160, 31.24680007765648071, -4.297206761780677731 ) ) ;
#9989=CARTESIAN_POINT ( 'NONE',  ( -4.481649420246396787, 14.62819992234354594, -1.518615910253363399 ) ) ;
#9990=CARTESIAN_POINT ( 'NONE',  ( 2.798362969681409851, 31.00319992234354416, 2.102939460078764977 ) ) ;
#9991=CARTESIAN_POINT ( 'NONE',  ( -1.497042530366477164, 37.62180007765646650, 2.161531897785062384 ) ) ;
#9994=CARTESIAN_POINT ( 'NONE',  ( 3.673772985318163098, 30.50319992234354416, -2.599342558261029001 ) ) ;
#10000=CARTESIAN_POINT ( 'NONE',  ( -2.864755990943265829, 30.74680007765647716, -2.011557305968488141 ) ) ;
#10005=CARTESIAN_POINT ( 'NONE',  ( 3.607379964056306676, 28.99680007765648071, -2.690724712371305838 ) ) ;
#10010=CARTESIAN_POINT ( 'NONE',  ( 3.500000000000000444, 26.74680007765648071, -0.05647727720536935281 ) ) ;
#10015=CARTESIAN_POINT ( 'NONE',  ( -2.115076519116425580, 17.37819992234354771, -3.012182706137062738 ) ) ;
#10017=CARTESIAN_POINT ( 'NONE',  ( -2.500000000000001332, 15.49680007765647893, 0.05647727720535858364 ) ) ;
#10018=CARTESIAN_POINT ( 'NONE',  ( 3.481649420246394122, 38.37819992234354771, 1.193696214020467439 ) ) ;
#10025=CARTESIAN_POINT ( 'NONE',  ( -3.000000000000001332, 15.00000000000000355, 3.048632113068340848E-14 ) ) ;
#10031=CARTESIAN_POINT ( 'NONE',  ( 2.500000000000001332, 23.25319992234354771, 0.05647727720530566764 ) ) ;
#10038=CARTESIAN_POINT ( 'NONE',  ( -0.05938372350927861171, 28.62180007765648071, -3.680117784833935701 ) ) ;
#10051=CARTESIAN_POINT ( 'NONE',  ( -0.8262555684461330152, 23.49680007765647716, -2.360188852285403982 ) ) ;
#10053=CARTESIAN_POINT ( 'NONE',  ( -3.481649420246370141, 25.37180007765647716, 1.193696214020542268 ) ) ;
#10058=CARTESIAN_POINT ( 'NONE',  ( -2.481649420246391902, 37.12819992234354771, -0.8687765177875723666 ) ) ;
#10061=CARTESIAN_POINT ( 'NONE',  ( -1.444289557196047014, 35.99680007765647360, -4.262301884875704161 ) ) ;
#10077=CARTESIAN_POINT ( 'NONE',  ( -3.607379964056363075, 14.75319992234354416, -2.690724712371229899 ) ) ;
#10078=CARTESIAN_POINT ( 'NONE',  ( 3.500000000000000444, 30.75319992234354416, 0.05647727720529520379 ) ) ;
#10079=CARTESIAN_POINT ( 'NONE',  ( 1.989345975306426206, 36.49680007765648071, -1.515154207786343799 ) ) ;
#10080=EDGE_CURVE ( 'NONE', #13037, #12310, #5229, .T. ) ;
#10082=CARTESIAN_POINT ( 'NONE',  ( 4.518350579753602325, 33.12819992234354771, -1.405661355842793725 ) ) ;
#10086=CARTESIAN_POINT ( 'NONE',  ( 1.027846397803542144, 28.74680007765647716, -3.346150245485522312 ) ) ;
#10089=CARTESIAN_POINT ( 'NONE',  ( -4.518350579753632523, 28.12180007765647716, -1.405661355842698468 ) ) ;
#10093=CARTESIAN_POINT ( 'NONE',  ( -2.864755990943265829, 20.74680007765647716, -2.011557305968488141 ) ) ;
#10099=CARTESIAN_POINT ( 'NONE',  ( -1.135272562821019626, 16.50319992234354416, 3.311245368580577164 ) ) ;
#10102=CARTESIAN_POINT ( 'NONE',  ( -1.027846397803541700, 39.99680007765648071, 3.346150245485522312 ) ) ;
#10105=CARTESIAN_POINT ( 'NONE',  ( -2.798362969681409851, 32.25319992234354771, -2.102939460078765421 ) ) ;
#10119=CARTESIAN_POINT ( 'NONE',  ( -1.643582917929414133, 15.00000000000000711, -2.763362831372398798 ) ) ;
#10122=CARTESIAN_POINT ( 'NONE',  ( 0.7188294034286553114, 18.75319992234354416, 2.395093729190349130 ) ) ;
#10126=CARTESIAN_POINT ( 'NONE',  ( 4.481649420246366589, 19.12180007765647360, -1.518615910253458212 ) ) ;
#10131=CARTESIAN_POINT ( 'NONE',  ( -0.05938372350927861171, 33.62180007765648071, -3.680117784833935701 ) ) ;
#10145=CARTESIAN_POINT ( 'NONE',  ( -1.593127413382998459, 23.37180007765648071, -2.091722143975139669 ) ) ;
#10147=CARTESIAN_POINT ( 'NONE',  ( -3.500000000000000444, 22.99680007765647716, 0.05647727720536892260 ) ) ;
#10151=CARTESIAN_POINT ( 'NONE',  ( -1.593127413382952939, 39.12819992234354771, 2.091722143975172532 ) ) ;
#10155=CARTESIAN_POINT ( 'NONE',  ( -2.829195390882805139, 35.87180007765647360, -3.793023760679206102 ) ) ;
#10173=CARTESIAN_POINT ( 'NONE',  ( 1.444289557195957086, 22.75319992234354061, -4.262301884875733471 ) ) ;
#10174=CARTESIAN_POINT ( 'NONE',  ( 1.135272562821020070, 27.75319992234354416, -3.311245368580577164 ) ) ;
#10175=CARTESIAN_POINT ( 'NONE',  ( 2.481649420246374138, 39.12180007765647360, -0.8687765177876252132 ) ) ;
#10178=CARTESIAN_POINT ( 'NONE',  ( -4.499999999999999112, 37.00319992234354771, -0.05647727720528529505 ) ) ;
#10183=CARTESIAN_POINT ( 'NONE',  ( 2.798362969681366330, 33.99680007765648071, -2.102939460078824929 ) ) ;
#10186=CARTESIAN_POINT ( 'NONE',  ( 1.444289557196047680, 29.74680007765648071, 4.262301884875704161 ) ) ;
#10190=CARTESIAN_POINT ( 'NONE',  ( -2.211161402132902243, 28.37180007765647716, -2.942372952327172886 ) ) ;
#10195=CARTESIAN_POINT ( 'NONE',  ( 2.211161402132839626, 17.87819992234354771, -2.942372952327218183 ) ) ;
#10198=CARTESIAN_POINT ( 'NONE',  ( -2.055738996568313048, 15.74680007765648071, -1.423772053676023441 ) ) ;
#10199=CARTESIAN_POINT ( 'NONE',  ( -3.518350579753605434, 31.87819992234354416, 1.080741659609877781 ) ) ;
#10216=CARTESIAN_POINT ( 'NONE',  ( 1.497042530366522461, 23.62819992234354416, 2.161531897785029965 ) ) ;
#10218=CARTESIAN_POINT ( 'NONE',  ( -3.500000000000000444, 15.49680007765647893, 0.05647727720536892260 ) ) ;
#10224=CARTESIAN_POINT ( 'NONE',  ( 2.864755990943265829, 39.49680007765647360, 2.011557305968487697 ) ) ;
#10238=CARTESIAN_POINT ( 'NONE',  ( -0.05938372350926768989, 26.12180007765648426, -2.628655560595669183 ) ) ;
#10240=CARTESIAN_POINT ( 'NONE',  ( 1.135272562821090458, 19.74680007765648071, 3.311245368580554072 ) ) ;
#10245=CARTESIAN_POINT ( 'NONE',  ( -2.864755990943222308, 19.25319992234354416, 2.011557305968548093 ) ) ;
#10248=CARTESIAN_POINT ( 'NONE',  ( 0.05938372350927906274, 17.37180007765647005, 3.680117784833935701 ) ) ;
#10267=CARTESIAN_POINT ( 'NONE',  ( 1.336863392178569754, 23.75319992234354771, 4.297206761780648421 ) ) ;
#10268=CARTESIAN_POINT ( 'NONE',  ( -1.135272562821019626, 31.50319992234354416, 3.311245368580577164 ) ) ;
#10269=CARTESIAN_POINT ( 'NONE',  ( 2.500000000000001332, 23.25319992234354771, 0.05647727720530566764 ) ) ;
#10271=CARTESIAN_POINT ( 'NONE',  ( -4.518350579753602325, 31.87819992234354416, 1.405661355842794391 ) ) ;
#10277=CARTESIAN_POINT ( 'NONE',  ( -2.798362969681365886, 32.74680007765648071, 2.102939460078824929 ) ) ;
#10280=CARTESIAN_POINT ( 'NONE',  ( -4.481649420246366589, 27.87180007765647716, 1.518615910253458878 ) ) ;
#10284=CARTESIAN_POINT ( 'NONE',  ( -2.115076519116362519, 32.62180007765646650, 3.012182706137107147 ) ) ;
#10292=CARTESIAN_POINT ( 'NONE',  ( 2.115076519116426024, 23.62819992234354416, 3.012182706137062294 ) ) ;
#10296=CARTESIAN_POINT ( 'NONE',  ( -1.497042530366477164, 22.62180007765647716, 2.161531897785062384 ) ) ;
#10297=CARTESIAN_POINT ( 'NONE',  ( -3.481649420246394122, 32.12819992234353350, -1.193696214020467883 ) ) ;
#10312=CARTESIAN_POINT ( 'NONE',  ( -1.989345975306457071, 29.75319992234354771, -1.515154207786300944 ) ) ;
#10314=CARTESIAN_POINT ( 'NONE',  ( -1.027846397803541700, 17.49680007765647716, 3.346150245485522312 ) ) ;
#10321=CARTESIAN_POINT ( 'NONE',  ( 1.135272562821090458, 39.74680007765648071, 3.311245368580554072 ) ) ;
#10333=CARTESIAN_POINT ( 'NONE',  ( 2.518350579753628971, 24.37180007765648071, 0.7558219633769073242 ) ) ;
#10335=CARTESIAN_POINT ( 'NONE',  ( 2.798362969681366330, 21.49680007765647716, -2.102939460078824929 ) ) ;
#10341=CARTESIAN_POINT ( 'NONE',  ( 3.518350579753605434, 18.12819992234353705, -1.080741659609877114 ) ) ;
#10345=CARTESIAN_POINT ( 'NONE',  ( 3.673772985318219053, 39.49680007765648071, 2.599342558260951730 ) ) ;
#10365=CARTESIAN_POINT ( 'NONE',  ( 2.733110507866328920, 26.12819992234354416, 3.862833514489095510 ) ) ;
#10367=CARTESIAN_POINT ( 'NONE',  ( 2.211161402132839182, 37.87819992234353350, -2.942372952327217739 ) ) ;
#10368=CARTESIAN_POINT ( 'NONE',  ( 2.518350579753611207, 23.12819992234354416, -0.7558219633769606149 ) ) ;
#10370=CARTESIAN_POINT ( 'NONE',  ( -2.829195390882805139, 15.87180007765647716, -3.793023760679206102 ) ) ;
#10375=CARTESIAN_POINT ( 'NONE',  ( -3.518350579753630747, 30.62180007765647716, -1.080741659609802729 ) ) ;
#10378=CARTESIAN_POINT ( 'NONE',  ( 0.05938372350929014415, 32.37180007765647360, 4.731580009072201776 ) ) ;
#10381=CARTESIAN_POINT ( 'NONE',  ( -2.864755990943265829, 28.24680007765648071, -2.011557305968488141 ) ) ;
#10388=CARTESIAN_POINT ( 'NONE',  ( -2.864755990943222308, 26.75319992234354771, 2.011557305968548093 ) ) ;
#10391=CARTESIAN_POINT ( 'NONE',  ( 2.055738996568313048, 19.49680007765648071, 1.423772053676023441 ) ) ;
#10394=CARTESIAN_POINT ( 'NONE',  ( -2.733110507866328476, 17.37819992234354416, -3.862833514489096398 ) ) ;
#10412=CARTESIAN_POINT ( 'NONE',  ( -0.05938372350921170689, 26.37819992234355126, 2.628655560595669183 ) ) ;
#10414=CARTESIAN_POINT ( 'NONE',  ( -2.211161402132902243, 23.37180007765647716, -2.942372952327172886 ) ) ;
#10417=CARTESIAN_POINT ( 'NONE',  ( 3.500000000000000444, 39.24680007765647360, -0.05647727720536935281 ) ) ;
#10429=CARTESIAN_POINT ( 'NONE',  ( 0.8262555684461332373, 27.24680007765648426, 2.360188852285403982 ) ) ;
#10431=CARTESIAN_POINT ( 'NONE',  ( 2.798362969681366330, 31.49680007765647716, -2.102939460078824929 ) ) ;
#10439=CARTESIAN_POINT ( 'NONE',  ( -2.211161402132839182, 19.12819992234353705, 2.942372952327218627 ) ) ;
#10442=CARTESIAN_POINT ( 'NONE',  ( -2.864755990943265829, 15.74680007765647716, -2.011557305968488141 ) ) ;
#10462=CARTESIAN_POINT ( 'NONE',  ( 1.444289557195957086, 25.25319992234354771, -4.262301884875733471 ) ) ;
#10463=CARTESIAN_POINT ( 'NONE',  ( 3.518350579753606322, 38.12819992234353350, -1.080741659609876892 ) ) ;
#10464=CARTESIAN_POINT ( 'NONE',  ( -1.497042530366522461, 19.87819992234354771, -2.161531897785030409 ) ) ;
#10467=CARTESIAN_POINT ( 'NONE',  ( 3.673772985318219053, 16.99680007765647716, 2.599342558260951730 ) ) ;
#10484=CARTESIAN_POINT ( 'NONE',  ( 2.798362969681409851, 23.50319992234354416, 2.102939460078764977 ) ) ;
#10487=CARTESIAN_POINT ( 'NONE',  ( 2.518350579753628971, 21.87180007765647360, 0.7558219633769073242 ) ) ;
#10489=CARTESIAN_POINT ( 'NONE',  ( -2.211161402132839182, 39.12819992234354771, 2.942372952327218627 ) ) ;
#10505=CARTESIAN_POINT ( 'NONE',  ( 2.055738996568281518, 30.50319992234354771, -1.423772053676066518 ) ) ;
#10508=CARTESIAN_POINT ( 'NONE',  ( 1.027846397803542144, 26.24680007765648071, -3.346150245485522312 ) ) ;
#10522=CARTESIAN_POINT ( 'NONE',  ( 1.497042530366477164, 31.37180007765648426, -2.161531897785062384 ) ) ;
#10525=CARTESIAN_POINT ( 'NONE',  ( -2.115076519116362519, 27.62180007765648071, 3.012182706137108035 ) ) ;
#10528=CARTESIAN_POINT ( 'NONE',  ( 1.027846397803612311, 21.25319992234354416, 3.346150245485499219 ) ) ;
#10531=CARTESIAN_POINT ( 'NONE',  ( -2.798362969681365886, 17.74680007765647716, 2.102939460078824929 ) ) ;
#10548=CARTESIAN_POINT ( 'NONE',  ( 2.829195390882724759, 22.87819992234354416, -3.793023760679264278 ) ) ;
#10549=CARTESIAN_POINT ( 'NONE',  ( 2.798362969681409851, 33.50319992234354771, 2.102939460078764977 ) ) ;
#10551=CARTESIAN_POINT ( 'NONE',  ( -2.518350579753611207, 21.87819992234354416, 0.7558219633769609480 ) ) ;
#10553=CARTESIAN_POINT ( 'NONE',  ( 3.607379964056306676, 18.99680007765647716, -2.690724712371305838 ) ) ;
#10559=CARTESIAN_POINT ( 'NONE',  ( 1.135272562821090458, 37.24680007765648071, 3.311245368580554072 ) ) ;
#10573=CARTESIAN_POINT ( 'NONE',  ( 2.798362969681409851, 31.00319992234354416, 2.102939460078764977 ) ) ;
#10576=CARTESIAN_POINT ( 'NONE',  ( -2.500000000000001332, 25.49680007765647716, 0.05647727720535858364 ) ) ;
#10578=CARTESIAN_POINT ( 'NONE',  ( -4.481649420246396787, 14.62819992234354594, -1.518615910253363399 ) ) ;
#10584=CARTESIAN_POINT ( 'NONE',  ( -3.500000000000000444, 15.49680007765647893, 0.05647727720536892260 ) ) ;
#10597=CARTESIAN_POINT ( 'NONE',  ( -1.989345975306457071, 32.25319992234354061, -1.515154207786300944 ) ) ;
#10600=CARTESIAN_POINT ( 'NONE',  ( -2.798362969681365886, 25.24680007765647716, 2.102939460078824929 ) ) ;
#10615=CARTESIAN_POINT ( 'NONE',  ( -0.7188294034286043521, 29.99680007765648071, 2.395093729190366005 ) ) ;
#10618=CARTESIAN_POINT ( 'NONE',  ( 0.05938372350927906967, 32.37180007765648071, 3.680117784833935701 ) ) ;
#10625=CARTESIAN_POINT ( 'NONE',  ( 3.500000000000000444, 19.24680007765648071, -0.05647727720536935281 ) ) ;
#10645=CARTESIAN_POINT ( 'NONE',  ( -0.05938372350918959958, 31.37819992234354061, 4.731580009072201776 ) ) ;
#10646=CARTESIAN_POINT ( 'NONE',  ( 1.135272562821020070, 32.75319992234354771, -3.311245368580577164 ) ) ;
#10648=CARTESIAN_POINT ( 'NONE',  ( 0.7188294034286553114, 21.25319992234354771, 2.395093729190349130 ) ) ;
#10650=CARTESIAN_POINT ( 'NONE',  ( 4.481649420246366589, 16.62180007765647716, -1.518615910253458212 ) ) ;
#10655=CARTESIAN_POINT ( 'NONE',  ( -3.500000000000000444, 40.49680007765648071, 0.05647727720536892260 ) ) ;
#10667=CARTESIAN_POINT ( 'NONE',  ( -3.481649420246394122, 27.12819992234354771, -1.193696214020467883 ) ) ;
#10670=CARTESIAN_POINT ( 'NONE',  ( 2.518350579753628971, 24.37180007765648071, 0.7558219633769073242 ) ) ;
#10672=CARTESIAN_POINT ( 'NONE',  ( 4.481649420246397675, 20.87819992234354416, 1.518615910253363177 ) ) ;
#10676=CARTESIAN_POINT ( 'NONE',  ( -3.607379964056306676, 35.24680007765647360, 2.690724712371306282 ) ) ;
#10689=CARTESIAN_POINT ( 'NONE',  ( -2.055738996568281518, 31.75319992234354771, 1.423772053676066962 ) ) ;
#10693=CARTESIAN_POINT ( 'NONE',  ( 2.798362969681366330, 26.49680007765648071, -2.102939460078824929 ) ) ;
#10706=CARTESIAN_POINT ( 'NONE',  ( -2.055738996568313048, 33.24680007765648782, -1.423772053676023441 ) ) ;
#10708=CARTESIAN_POINT ( 'NONE',  ( 2.211161402132902243, 32.12180007765648071, 2.942372952327172442 ) ) ;
#10715=CARTESIAN_POINT ( 'NONE',  ( 0.05938372350927906274, 22.37180007765648071, 3.680117784833935701 ) ) ;
#10730=CARTESIAN_POINT ( 'NONE',  ( -2.798362969681365886, 35.24680007765648071, 2.102939460078824929 ) ) ;
#10736=CARTESIAN_POINT ( 'NONE',  ( -4.518350579753602325, 34.37819992234354771, 1.405661355842794391 ) ) ;
#10737=CARTESIAN_POINT ( 'NONE',  ( -2.211161402132838738, 34.12819992234354771, 2.942372952327218183 ) ) ;
#10739=CARTESIAN_POINT ( 'NONE',  ( 1.497042530366522461, 28.62819992234355126, 2.161531897785029965 ) ) ;
#10741=CARTESIAN_POINT ( 'NONE',  ( -1.336863392178478716, 19.99680007765647716, 4.297206761780677731 ) ) ;
#10747=CARTESIAN_POINT ( 'NONE',  ( 1.135272562821090458, 39.74680007765648071, 3.311245368580554072 ) ) ;
#10759=CARTESIAN_POINT ( 'NONE',  ( -0.05938372350920063936, 38.87819992234354771, 3.680117784833935701 ) ) ;
#10763=CARTESIAN_POINT ( 'NONE',  ( 1.497042530366477164, 28.87180007765648426, -2.161531897785062384 ) ) ;
#10764=CARTESIAN_POINT ( 'NONE',  ( 2.829195390882724759, 15.37819992234354594, -3.793023760679264278 ) ) ;
#10768=CARTESIAN_POINT ( 'NONE',  ( -0.05938372350928957516, 38.62180007765647360, -4.731580009072201776 ) ) ;
#10775=ORIENTED_EDGE ( 'NONE', *, *, #2547, .F. ) ;
#10776=CARTESIAN_POINT ( 'NONE',  ( -2.115076519116362519, 17.62180007765647716, 3.012182706137107147 ) ) ;
#10780=CARTESIAN_POINT ( 'NONE',  ( -2.500000000000001332, 39.50319992234355482, -0.05647727720530596601 ) ) ;
#10782=CARTESIAN_POINT ( 'NONE',  ( -3.481649420246369697, 22.87180007765647360, 1.193696214020542490 ) ) ;
#10791=CARTESIAN_POINT ( 'NONE',  ( 0.05938372350929014415, 24.87180007765647716, 4.731580009072201776 ) ) ;
#10801=CARTESIAN_POINT ( 'NONE',  ( -2.500000000000001332, 27.99680007765648426, 0.05647727720535858364 ) ) ;
#10803=CARTESIAN_POINT ( 'NONE',  ( 2.115076519116362963, 31.37180007765647716, -3.012182706137107591 ) ) ;
#10809=CARTESIAN_POINT ( 'NONE',  ( 3.481649420246369697, 26.62180007765648071, -1.193696214020541824 ) ) ;
#10820=CARTESIAN_POINT ( 'NONE',  ( 2.115076519116362963, 33.87180007765648071, -3.012182706137107147 ) ) ;
#10824=CARTESIAN_POINT ( 'NONE',  ( 3.607379964056363075, 36.00319992234354771, 2.690724712371229010 ) ) ;
#10826=CARTESIAN_POINT ( 'NONE',  ( 1.497042530366522461, 31.12819992234354416, 2.161531897785029965 ) ) ;
#10829=CARTESIAN_POINT ( 'NONE',  ( 4.499999999999999112, 29.24680007765647716, -0.05647727720537982360 ) ) ;
#10834=CARTESIAN_POINT ( 'NONE',  ( 2.798362969681366330, 36.49680007765648071, -2.102939460078824929 ) ) ;
#10846=CARTESIAN_POINT ( 'NONE',  ( -3.518350579753605434, 36.87819992234354771, 1.080741659609877781 ) ) ;
#10849=CARTESIAN_POINT ( 'NONE',  ( 1.989345975306426206, 26.49680007765648426, -1.515154207786343799 ) ) ;
#10850=CARTESIAN_POINT ( 'NONE',  ( -3.607379964056363075, 27.25319992234354771, -2.690724712371229899 ) ) ;
#10857=CARTESIAN_POINT ( 'NONE',  ( 0.05938372350929014415, 37.37180007765647360, 4.731580009072201776 ) ) ;
#10870=CARTESIAN_POINT ( 'NONE',  ( -2.481649420246391902, 34.62819992234354771, -0.8687765177875723666 ) ) ;
#10872=CARTESIAN_POINT ( 'NONE',  ( 3.500000000000000444, 31.74680007765647716, -0.05647727720536935281 ) ) ;
#10873=CARTESIAN_POINT ( 'NONE',  ( -3.518350579753605434, 29.37819992234354416, 1.080741659609877781 ) ) ;
#10881=CARTESIAN_POINT ( 'NONE',  ( 1.444289557196047680, 24.74680007765647716, 4.262301884875704161 ) ) ;
#10889=CARTESIAN_POINT ( 'NONE',  ( -0.05938372350926768989, 36.12180007765648071, -2.628655560595669183 ) ) ;
#10891=CARTESIAN_POINT ( 'NONE',  ( -2.864755990943265829, 38.24680007765647360, -2.011557305968488141 ) ) ;
#10896=CARTESIAN_POINT ( 'NONE',  ( -2.417956891975437728, 15.00000000000001066, -3.010107623731891113 ) ) ;
#10900=CARTESIAN_POINT ( 'NONE',  ( -0.05938372350927861171, 23.62180007765647005, -3.680117784833935701 ) ) ;
#10906=( GEOMETRIC_REPRESENTATION_CONTEXT ( 3 ) GLOBAL_UNCERTAINTY_ASSIGNED_CONTEXT ( ( #14002 ) ) GLOBAL_UNIT_ASSIGNED_CONTEXT ( ( #2985, #480, #3358 ) ) REPRESENTATION_CONTEXT ( 'NONE', 'WORKASPACE' ) );
#10914=CARTESIAN_POINT ( 'NONE',  ( 1.027846397803542144, 36.24680007765648071, -3.346150245485522312 ) ) ;
#10918=CARTESIAN_POINT ( 'NONE',  ( -2.733110507866328476, 37.37819992234354771, -3.862833514489096398 ) ) ;
#10921=CARTESIAN_POINT ( 'NONE',  ( 2.055738996568281518, 30.50319992234354771, -1.423772053676066518 ) ) ;
#10924=CARTESIAN_POINT ( 'NONE',  ( 3.673772985318219053, 26.99680007765647716, 2.599342558260951730 ) ) ;
#10940=CARTESIAN_POINT ( 'NONE',  ( -1.135272562821019626, 34.00319992234354771, 3.311245368580577164 ) ) ;
#10941=CARTESIAN_POINT ( 'NONE',  ( 3.481649420246395010, 20.87819992234354416, 1.193696214020467439 ) ) ;
#10943=CARTESIAN_POINT ( 'NONE',  ( 0.8262555684461332373, 29.74680007765648426, 2.360188852285403982 ) ) ;
#10944=CARTESIAN_POINT ( 'NONE',  ( 2.733110507866328920, 26.12819992234354416, 3.862833514489095510 ) ) ;
#10949=CARTESIAN_POINT ( 'NONE',  ( 3.673772985318219053, 36.99680007765647360, 2.599342558260951730 ) ) ;
#10958=CARTESIAN_POINT ( 'NONE',  ( -1.135272562821090014, 15.99680007765647716, -3.311245368580554072 ) ) ;
#10965=CARTESIAN_POINT ( 'NONE',  ( 2.500000000000001332, 33.25319992234354771, 0.05647727720530566764 ) ) ;
#10967=CARTESIAN_POINT ( 'NONE',  ( -3.518350579753630747, 33.12180007765646650, -1.080741659609802729 ) ) ;
#10969=CARTESIAN_POINT ( 'NONE',  ( -1.027846397803611866, 25.00319992234354416, -3.346150245485499219 ) ) ;
#10977=CARTESIAN_POINT ( 'NONE',  ( 1.444289557196047680, 22.24680007765647716, 4.262301884875704161 ) ) ;
#10983=CARTESIAN_POINT ( 'NONE',  ( -2.518350579753628526, 35.62180007765647360, -0.7558219633769075463 ) ) ;
#10985=CARTESIAN_POINT ( 'NONE',  ( 0.05938372350927906967, 37.37180007765647360, 3.680117784833935701 ) ) ;
#10991=CARTESIAN_POINT ( 'NONE',  ( -3.500000000000000444, 22.99680007765647716, 0.05647727720536892260 ) ) ;
#11003=CARTESIAN_POINT ( 'NONE',  ( -2.211161402132902243, 38.37180007765648071, -2.942372952327172886 ) ) ;
#11006=CARTESIAN_POINT ( 'NONE',  ( -1.336863392178569088, 37.50319992234353350, -4.297206761780648421 ) ) ;
#11007=CARTESIAN_POINT ( 'NONE',  ( -1.593127413382952939, 31.62819992234354416, 2.091722143975172532 ) ) ;
#11011=CARTESIAN_POINT ( 'NONE',  ( 2.733110507866247652, 26.37180007765647716, -3.862833514489153686 ) ) ;
#11026=CARTESIAN_POINT ( 'NONE',  ( 2.798362969681366330, 16.49680007765647716, -2.102939460078824929 ) ) ;
#11029=CARTESIAN_POINT ( 'NONE',  ( -2.211161402132839182, 36.62819992234354771, 2.942372952327218627 ) ) ;
#11030=CARTESIAN_POINT ( 'NONE',  ( -1.135272562821019626, 21.50319992234354416, 3.311245368580577164 ) ) ;
#11032=CARTESIAN_POINT ( 'NONE',  ( 1.989345975306426206, 28.99680007765648071, -1.515154207786343799 ) ) ;
#11034=CARTESIAN_POINT ( 'NONE',  ( 2.829195390882724759, 25.37819992234354416, -3.793023760679264278 ) ) ;
#11040=CARTESIAN_POINT ( 'NONE',  ( -3.518350579753630747, 25.62180007765648071, -1.080741659609802729 ) ) ;
#11044=AXIS2_PLACEMENT_3D ( 'NONE', #805, #5057, #14536 ) ;
#11055=CARTESIAN_POINT ( 'NONE',  ( -0.8262555684460826111, 34.00319992234354771, 2.360188852285421302 ) ) ;
#11057=CARTESIAN_POINT ( 'NONE',  ( 3.481649420246369697, 34.12180007765648071, -1.193696214020541824 ) ) ;
#11058=CARTESIAN_POINT ( 'NONE',  ( 3.518350579753605434, 23.12819992234354416, -1.080741659609877114 ) ) ;
#11070=CARTESIAN_POINT ( 'NONE',  ( 0.8262555684461332373, 37.24680007765648071, 2.360188852285403982 ) ) ;
#11072=CARTESIAN_POINT ( 'NONE',  ( 3.500000000000000444, 39.24680007765647360, -0.05647727720536935281 ) ) ;
#11074=CARTESIAN_POINT ( 'NONE',  ( -1.454122949574299328, 15.00000000000144595, -3.397310229520432934 ) ) ;
#11077=CARTESIAN_POINT ( 'NONE',  ( 1.135272562821090458, 22.24680007765648071, 3.311245368580554072 ) ) ;
#11088=CARTESIAN_POINT ( 'NONE',  ( 3.481649420246369697, 39.12180007765646650, -1.193696214020541824 ) ) ;
#11090=( BOUNDED_SURFACE ( )  B_SPLINE_SURFACE ( 3, 2, ( 
 ( #12530, #9293, #13930, #5307, #10958, #16642, #4007, #7895, #1144, #15057, #3914, #5397, #3820, #1238, #9568, #15245, #5119, #10776, #16545, #2361, #2540, #6782, #12438, #16820, #963, #12162, #18130, #2451, #13552, #12254, #868, #17940, #5213, #3730, #15773, #5840, #14380, #9834, #12978, #7136, #6959, #11583, #10093, #12799, #4188, #9919, #2981, #15592, #9745, #4457, #1417, #3072, #1683, #17005, #15512, #11396, #4276, #14290, #17087, #1328, #106, #14106, #5760, #2892, #15427, #7046, #12709, #8527, #7316, #11224, #2724, #293, #8705, #5935, #5666, #11489, #12617, #14, #4094, #16911, #1501, #4359, #18305, #14198, #11310, #8356, #14017, #17184, #5575, #2808, #10010, #15686, #8438, #8612, #1593, #7227, #12885, #191, #12209, #7413, #6648, #6119, #10381, #10190, #8802, #3260, #15869, #475, #17276, #9336, #7511, #15013, #13601, #14484, #9000, #1878, #915, #4549, #6558, #13072, #9425, #3353, #14675, #17370, #16405, #6026, #1783, #16495, #12117, #17894, #388, #3166, #11769, #16061, #11676, #4635, #8897, #10284, #17465, #15968, #2311, #13164, #7944, #5166, #14575, #1973, #4734, #10820, #7598, #13507, #823, #6467, #3690, #15101, #3773, #17812, #1009, #5073, #10730, #2404, #8036, #13695, #4042, #9694, #15377, #14056, #10914, #16865, #12392, #2676, #8395, #6828, #5623, #6915, #8312, #8127, #2497, #13881, #5351, #13967, #12571, #1283, #2847, #11003, #15196, #11175, #1191, #12475, #16682, #11088, #9612, #15284, #9515, #11267, #1367, #4235, #18080, #8477, #18259, #13785, #1461 ),
 ( #17987, #12660, #2584, #18351, #9876, #18173, #3959, #5529, #5441, #4141, #9789, #1096, #15470, #8217, #2766, #16773, #5258, #6998, #16955, #15551, #14149, #6736, #16590, #12297, #3869, #16012, #8660, #8849, #15637, #4409, #3304, #14244, #4502, #8754, #4315, #1635, #3026, #4683, #17417, #11536, #17229, #7185, #5979, #1547, #9962, #6069, #1732, #1826, #2936, #14626, #14337, #242, #58, #17044, #11441, #5716, #7272, #7091, #17325, #15728, #4589, #3214, #8571, #10145, #10051, #14529, #12757, #15824, #5888, #12843, #11632, #10333, #7462, #147, #8946, #3120, #12928, #11355, #5797, #13122, #14428, #7366, #13026, #431, #17132, #10238, #341, #15915, #11723, #14813, #13573, #14909, #12001, #16109, #10429, #3486, #13309, #4960, #2203, #3577, #10801, #622, #4777, #799, #9133, #2111, #6261, #711, #17610, #4872, #17515, #893, #3671, #12187, #7643, #16470, #10615, #3399, #9401, #7919, #16290, #2016, #7741, #6445, #13399, #7553, #2290, #10522, #6535, #17874, #6359, #11913, #9227, #17695, #12093, #7829, #9042, #13485, #16195, #17789, #5050, #13208, #10706, #16382, #9316, #5143, #14718, #525, #3752, #1929, #6170, #14989, #11819, #5234, #12365, #5604, #3848, #12456, #16753, #12276, #9588, #10983, #12641, #2382, #4121, #10889, #2475, #4027, #15267, #6893, #9674, #17965, #5421, #6714, #11070, #2564, #8014, #18059, #5332, #8196, #18331, #9493, #13667, #11249, #8376, #16937, #16661, #16844, #16568, #3938, #4210, #15171, #18152, #15355, #8105, #13859, #1167, #15078, #987, #9770, #13764 ),
 ( #6631, #1076, #6807, #2654, #8291, #13948, #14038, #1347, #1261, #12552, #18238, #5507, #6979, #11154, #15447, #2743, #1528, #11702, #1711, #4573, #6053, #7070, #14318, #5957, #15533, #9857, #318, #14510, #14128, #8550, #15707, #11517, #1616, #5868, #10122, #1807, #2829, #8458, #3005, #1440, #15895, #8640, #17397, #7345, #7249, #4480, #219, #11612, #8731, #11420, #12908, #12738, #17208, #7442, #12823, #126, #17111, #15803, #3099, #39, #3192, #5693, #13101, #2916, #14225, #4386, #4297, #13006, #11333, #14404, #10031, #17027, #17307, #10216, #9943, #415, #8831, #15614, #7163, #5778, #3564, #9116, #1997, #3287, #6427, #16272, #873, #14794, #15995, #16089, #3650, #17494, #13189, #9023, #696, #10412, #14700, #5035, #7900, #504, #3382, #11798, #4854, #602, #16363, #9297, #13556, #14605, #6519, #11985, #14976, #2273, #12073, #9210, #7624, #12167, #14888, #17772, #4662, #1907, #2092, #782, #10312, #8923, #13471, #7537, #6149, #13290, #10505, #6341, #7720, #17679, #4941, #4760, #6242, #11892, #16175, #17591, #10689, #3471, #13381, #2185, #10597, #7813, #8178, #13935, #16736, #1059, #16647, #16453, #10965, #9750, #2457, #8087, #6694, #3920, #11055, #6965, #11139, #17858, #4100, #10870, #3826, #12348, #12258, #15335, #9384, #2546, #18040, #5123, #2635, #6788, #17944, #2729, #9572, #13838, #1243, #8362, #4013, #15251, #15152, #3734, #6877, #9656, #14022, #1333, #5312, #1148, #8275, #12444, #16550, #12535, #13748, #15432, #18224, #18136, #5493, #5404, #16827, #13650, #10780 ),
 ( #15062, #2365, #6614, #7996, #970, #5216, #9477, #5764, #5583, #4194, #17011, #11230, #14204, #1788, #4462, #2898, #10099, #8712, #9841, #4364, #15597, #14385, #12623, #10015, #11401, #1424, #11494, #10195, #1689, #21, #14489, #15690, #8533, #15875, #18312, #12984, #2988, #8619, #14297, #7322, #16918, #17189, #12715, #1598, #298, #7143, #5940, #7232, #12890, #8442, #2814, #1508, #5672, #197, #5848, #15781, #3171, #11317, #15517, #3079, #12805, #111, #4282, #17093, #9925, #11589, #14112, #17285, #4554, #8808, #7052, #16337, #10484, #10292, #14958, #13449, #16158, #7517, #13264, #6319, #582, #13077, #7794, #4740, #763, #5011, #1977, #13169, #14772, #7603, #17660, #2070, #4640, #3450, #17471, #9091, #6223, #395, #10388, #16066, #11872, #10667, #14581, #6031, #3628, #6408, #9278, #9006, #9186, #15973, #3361, #7420, #1886, #4836, #7699, #3266, #17564, #14681, #11682, #17375, #14867, #8904, #17749, #13360, #672, #482, #11968, #6125, #11776, #12053, #4922, #2162, #10573, #16248, #3542, #3801, #6673, #13815, #9724, #13910, #2253, #6855, #13629, #6585, #9456, #15039, #18110, #12142, #5285, #15129, #7878, #5380, #9545, #2344, #5468, #1033, #10940, #16712, #11113, #1126, #12327, #17922, #852, #3985, #6761, #16802, #4072, #2433, #8059, #12419, #13722, #941, #15312, #5194, #12509, #9634, #16623, #11029, #18013, #10846, #16434, #3898, #2523, #17835, #15223, #6497, #8153, #12236, #2611, #1218, #8251, #18204, #16522, #13535, #5099, #10759, #3713, #9363, #7976, #14364, #9813 ),
 ( #1663, #9989, #10077, #5556, #4531, #4259, #8504, #8336, #6942, #1396, #13995, #16982, #15409, #7212, #5647, #12866, #11469, #12595, #7118, #1568, #17163, #2704, #12778, #14177, #4170, #14271, #12959, #4437, #2791, #17258, #87, #11290, #274, #1310, #15756, #5740, #11380, #17067, #3056, #18283, #1574, #15494, #4342, #8687, #9902, #7299, #15664, #2962, #11204, #16893, #15573, #8422, #8596, #173, #5824, #5918, #1484, #14084, #11563, #7023, #12688, #2874, #12030, #7582, #6101, #7769, #10173, #10548, #1956, #13240, #558, #11947, #8782, #14749, #10267, #6200, #6293, #4715, #3517, #4814, #11849, #6007, #368, #11753, #3244, #17544, #10462, #16140, #743, #8882, #13057, #9070, #17447, #10365, #14560, #8983, #7491, #13149, #7397, #9164, #17641, #2138, #15947, #6387, #3429, #11662, #17723, #16224, #2046, #1860, #16045, #7676, #3337, #15850, #14845, #460, #13429, #3147, #14656, #13340, #650, #4898, #14462, #1766, #17354, #4617, #15018, #1013, #17900, #16317, #7949, #2318, #16500, #8222, #12122, #10645, #2588, #16685, #13886, #6562, #6740, #13513, #13606, #1196, #17816, #2409, #6654, #2230, #5170, #920, #6832, #3602, #12396, #829, #15288, #9431, #15106, #5077, #3874, #10736, #7856, #3963, #17992, #18085, #6470, #12481, #12213, #3779, #9253, #14938, #9340, #16410, #10824, #4989, #15202, #8040, #2501, #1100, #3694, #13701, #12301, #5358, #5264, #10918, #11006, #16596, #8130, #9520, #13790, #9615, #15474, #12665, #16776, #9794, #4047, #14059, #6919, #2771, #14408, #15807, #8734 ),
 ( #13974, #1714, #8314, #9697, #12575, #1371, #1288, #18262, #3103, #13009, #15382, #5532, #2681, #16868, #11180, #7348, #322, #5960, #4147, #18176, #7001, #5445, #11092, #8401, #222, #5870, #11521, #17211, #4483, #10126, #13567, #2468, #12703, #3662, #16375, #7039, #2887, #2282, #15071, #3839, #18051, #8096, #12359, #16655, #8520, #9308, #14982, #9486, #7912, #4271, #15162, #99, #8433, #13758, #10977, #6705, #9, #15260, #17955, #1068, #884, #5324, #14193, #980, #6624, #5227, #3931, #9581, #5755, #9914, #6528, #1496, #9394, #2376, #10881, #10791, #14100, #12178, #2556, #16561, #17867, #1411, #5660, #16462, #7131, #11304, #16998, #15587, #12794, #5133, #3743, #13660, #8006, #12268, #4632, #7595, #13253, #289, #17272, #10280, #4544, #10089, #6116, #8701, #3350, #15962, #15864, #14375, #10005, #13161, #3257, #572, #11391, #5931, #10186, #8895, #3161, #15769, #11766, #1679, #8997, #7505, #14478, #14572, #8798, #7312, #7223, #1780, #11673, #2977, #7410, #15682, #13069, #3068, #384, #10378, #471, #17460, #12972, #4730, #11578, #1875, #16057, #17083, #14671, #1589, #1969, #6022, #17367, #11483, #4355, #187, #14286, #8607, #12880, #5836, #17180, #4452, #10676, #1043, #18023, #6330, #5296, #3722, #8073, #6682, #3810, #954, #6417, #16633, #6597, #9466, #10949, #11976, #860, #10857, #2079, #14781, #5205, #12336, #683, #13461, #2263, #16443, #6508, #10768, #15048, #3906, #7709, #13368, #7887, #17668, #2442, #13545, #4931, #12243, #12154, #9373, #5110, #16533, #13639 ),
 ( #10584, #7802, #16260, #17932, #3640, #9286, #771, #17844, #12061, #17759, #3552, #13732, #15138, #9195, #2172, #14876, #2354, #5023, #16346, #14966, #7984, #9643, #15418, #8430, #2621, #12606, #9823, #11213, #96, #8261, #12429, #14094, #16812, #4082, #13920, #8346, #6864, #12520, #6771, #2884, #11300, #1493, #15321, #5750, #18296, #18121, #17079, #15582, #5566, #1229, #2714, #1408, #14006, #15234, #9911, #18212, #8516, #7128, #9735, #5480, #16903, #1318, #7036, #4179, #5389, #15505, #11124, #2800, #6951, #2532, #12698, #6, #5657, #12790, #16723, #8161, #11388, #14189, #9558, #16993, #4268, #11040, #13826, #1135, #3997, #1776, #6019, #1585, #468, #15860, #6111, #11858, #11763, #12875, #14667, #8793, #14475, #4448, #3252, #11480, #7220, #3347, #17363, #17457, #7590, #8604, #10086, #14569, #15677, #14282, #8697, #2974, #5928, #4351, #1871, #12969, #7501, #4724, #182, #7406, #7309, #10375, #10000, #13065, #3157, #17174, #8891, #1965, #16054, #15766, #6210, #380, #284, #13250, #5833, #8993, #11670, #4628, #10277, #569, #3065, #13158, #14372, #15958, #1674, #17269, #11574, #4541, #10183, #13349, #7687, #751, #1023, #14947, #13438, #15113, #17554, #17911, #9263, #2239, #7865, #929, #16147, #3702, #17649, #13523, #13616, #12039, #10834, #12130, #839, #659, #6305, #6396, #10559, #6481, #17824, #5086, #8048, #16236, #2057, #16420, #17735, #4999, #3527, #16327, #14854, #2147, #14759, #16509, #6571, #9441, #4907, #13711, #10747, #11956, #6663, #5179, #9349, #9174, #10655 ) ),
 .UNSPECIFIED., .T., .F., .T. ) 
 B_SPLINE_SURFACE_WITH_KNOTS ( ( 4, 3, 4 ),
 ( 3, 2, 2, 2, 2, 2, 2, 2, 2, 2, 2, 2, 2, 2, 2, 2, 2, 2, 2, 2, 2, 2, 2, 2, 2, 2, 2, 2, 2, 2, 2, 2, 2, 2, 2, 2, 2, 2, 2, 2, 2, 2, 2, 2, 2, 2, 2, 2, 2, 2, 2, 2, 2, 2, 2, 2, 2, 2, 2, 2, 2, 2, 2, 2, 2, 2, 2, 2, 2, 2, 2, 2, 2, 2, 2, 2, 2, 2, 2, 2, 2, 2, 2, 2, 2, 2, 2, 2, 2, 2, 2, 2, 2, 2, 2, 2, 2, 2, 2, 2, 3 ),
 ( 0.000000000000000000, 0.5000000000000000000, 1.000000000000000000 ),
 ( 0.000000000000000000, 0.01000000000000000021, 0.02000000000000000042, 0.02999999999999999889, 0.04000000000000000083, 0.05000000000000000278, 0.05999999999999999778, 0.07000000000000000666, 0.08000000000000000167, 0.08999999999999999667, 0.1000000000000000056, 0.1100000000000000006, 0.1199999999999999956, 0.1300000000000000044, 0.1400000000000000133, 0.1499999999999999944, 0.1600000000000000033, 0.1700000000000000122, 0.1799999999999999933, 0.1900000000000000022, 0.2000000000000000111, 0.2099999999999999922, 0.2200000000000000011, 0.2300000000000000100, 0.2399999999999999911, 0.2500000000000000000, 0.2600000000000000089, 0.2700000000000000178, 0.2800000000000000266, 0.2899999999999999800, 0.2999999999999999889, 0.3099999999999999978, 0.3200000000000000067, 0.3300000000000000155, 0.3400000000000000244, 0.3499999999999999778, 0.3599999999999999867, 0.3699999999999999956, 0.3800000000000000044, 0.3900000000000000133, 0.4000000000000000222, 0.4099999999999999756, 0.4199999999999999845, 0.4299999999999999933, 0.4400000000000000022, 0.4500000000000000111, 0.4600000000000000200, 0.4699999999999999734, 0.4799999999999999822, 0.4899999999999999911, 0.5000000000000000000, 0.5100000000000000089, 0.5200000000000000178, 0.5300000000000000266, 0.5400000000000000355, 0.5500000000000000444, 0.5600000000000000533, 0.5699999999999999512, 0.5799999999999999600, 0.5899999999999999689, 0.5999999999999999778, 0.6099999999999999867, 0.6199999999999999956, 0.6300000000000000044, 0.6400000000000000133, 0.6500000000000000222, 0.6600000000000000311, 0.6700000000000000400, 0.6800000000000000488, 0.6899999999999999467, 0.6999999999999999556, 0.7099999999999999645, 0.7199999999999999734, 0.7299999999999999822, 0.7399999999999999911, 0.7500000000000000000, 0.7600000000000000089, 0.7700000000000000178, 0.7800000000000000266, 0.7900000000000000355, 0.8000000000000000444, 0.8100000000000000533, 0.8199999999999999512, 0.8299999999999999600, 0.8399999999999999689, 0.8499999999999999778, 0.8599999999999999867, 0.8699999999999999956, 0.8800000000000000044, 0.8900000000000000133, 0.9000000000000000222, 0.9100000000000000311, 0.9200000000000000400, 0.9300000000000000488, 0.9399999999999999467, 0.9499999999999999556, 0.9599999999999999645, 0.9699999999999999734, 0.9799999999999999822, 0.9899999999999999911, 1.000000000000000000 ),
 .UNSPECIFIED. ) 
 GEOMETRIC_REPRESENTATION_ITEM ( )  RATIONAL_B_SPLINE_SURFACE ( (
 ( 1.000000000000000000, 0.9510565162951535312, 1.000000000000000000, 0.9510565162951535312, 1.000000000000000000, 0.9510565162951535312, 1.000000000000000000, 0.9510565162951535312, 1.000000000000000000, 0.9510565162951535312, 1.000000000000000000, 0.9510565162951535312, 1.000000000000000000, 0.9510565162951535312, 1.000000000000000000, 0.9510565162951535312, 1.000000000000000000, 0.9510565162951535312, 1.000000000000000000, 0.9510565162951535312, 1.000000000000000000, 0.9510565162951535312, 1.000000000000000000, 0.9510565162951535312, 1.000000000000000000, 0.9510565162951535312, 1.000000000000000000, 0.9510565162951535312, 1.000000000000000000, 0.9510565162951535312, 1.000000000000000000, 0.9510565162951535312, 1.000000000000000000, 0.9510565162951535312, 1.000000000000000000, 0.9510565162951535312, 1.000000000000000000, 0.9510565162951535312, 1.000000000000000000, 0.9510565162951535312, 1.000000000000000000, 0.9510565162951535312, 1.000000000000000000, 0.9510565162951535312, 1.000000000000000000, 0.9510565162951535312, 1.000000000000000000, 0.9510565162951535312, 1.000000000000000000, 0.9510565162951535312, 1.000000000000000000, 0.9510565162951535312, 1.000000000000000000, 0.9510565162951535312, 1.000000000000000000, 0.9510565162951535312, 1.000000000000000000, 0.9510565162951535312, 1.000000000000000000, 0.9510565162951535312, 1.000000000000000000, 0.9510565162951535312, 1.000000000000000000, 0.9510565162951535312, 1.000000000000000000, 0.9510565162951535312, 1.000000000000000000, 0.9510565162951535312, 1.000000000000000000, 0.9510565162951535312, 1.000000000000000000, 0.9510565162951535312, 1.000000000000000000, 0.9510565162951535312, 1.000000000000000000, 0.9510565162951535312, 1.000000000000000000, 0.9510565162951535312, 1.000000000000000000, 0.9510565162951535312, 1.000000000000000000, 0.9510565162951535312, 1.000000000000000000, 0.9510565162951535312, 1.000000000000000000, 0.9510565162951535312, 1.000000000000000000, 0.9510565162951535312, 1.000000000000000000, 0.9510565162951535312, 1.000000000000000000, 0.9510565162951535312, 1.000000000000000000, 0.9510565162951535312, 1.000000000000000000, 0.9510565162951535312, 1.000000000000000000, 0.9510565162951535312, 1.000000000000000000, 0.9510565162951535312, 1.000000000000000000, 0.9510565162951535312, 1.000000000000000000, 0.9510565162951535312, 1.000000000000000000, 0.9510565162951535312, 1.000000000000000000, 0.9510565162951535312, 1.000000000000000000, 0.9510565162951535312, 1.000000000000000000, 0.9510565162951535312, 1.000000000000000000, 0.9510565162951535312, 1.000000000000000000, 0.9510565162951535312, 1.000000000000000000, 0.9510565162951535312, 1.000000000000000000, 0.9510565162951535312, 1.000000000000000000, 0.9510565162951535312, 1.000000000000000000, 0.9510565162951535312, 1.000000000000000000, 0.9510565162951535312, 1.000000000000000000, 0.9510565162951535312, 1.000000000000000000, 0.9510565162951535312, 1.000000000000000000, 0.9510565162951535312, 1.000000000000000000, 0.9510565162951535312, 1.000000000000000000, 0.9510565162951535312, 1.000000000000000000, 0.9510565162951535312, 1.000000000000000000, 0.9510565162951535312, 1.000000000000000000, 0.9510565162951535312, 1.000000000000000000, 0.9510565162951535312, 1.000000000000000000, 0.9510565162951535312, 1.000000000000000000, 0.9510565162951535312, 1.000000000000000000, 0.9510565162951535312, 1.000000000000000000, 0.9510565162951535312, 1.000000000000000000, 0.9510565162951535312, 1.000000000000000000, 0.9510565162951535312, 1.000000000000000000, 0.9510565162951535312, 1.000000000000000000, 0.9510565162951535312, 1.000000000000000000, 0.9510565162951535312, 1.000000000000000000, 0.9510565162951535312, 1.000000000000000000, 0.9510565162951535312, 1.000000000000000000, 0.9510565162951535312, 1.000000000000000000, 0.9510565162951535312, 1.000000000000000000, 0.9510565162951535312, 1.000000000000000000, 0.9510565162951535312, 1.000000000000000000, 0.9510565162951535312, 1.000000000000000000, 0.9510565162951535312, 1.000000000000000000, 0.9510565162951535312, 1.000000000000000000, 0.9510565162951535312, 1.000000000000000000, 0.9510565162951535312, 1.000000000000000000, 0.9510565162951535312, 1.000000000000000000, 0.9510565162951535312, 1.000000000000000000, 0.9510565162951535312, 1.000000000000000000, 0.9510565162951535312, 1.000000000000000000, 0.9510565162951535312, 1.000000000000000000, 0.9510565162951535312, 1.000000000000000000, 0.9510565162951535312, 1.000000000000000000, 0.9510565162951535312, 1.000000000000000000),
 ( 0.3333333333333333703, 0.3170188387650512141, 0.3333333333333333703, 0.3170188387650512141, 0.3333333333333333703, 0.3170188387650512141, 0.3333333333333333703, 0.3170188387650512141, 0.3333333333333333703, 0.3170188387650512141, 0.3333333333333333703, 0.3170188387650512141, 0.3333333333333333703, 0.3170188387650512141, 0.3333333333333333703, 0.3170188387650512141, 0.3333333333333333703, 0.3170188387650512141, 0.3333333333333333703, 0.3170188387650512141, 0.3333333333333333703, 0.3170188387650512141, 0.3333333333333333703, 0.3170188387650512141, 0.3333333333333333703, 0.3170188387650512141, 0.3333333333333333703, 0.3170188387650512141, 0.3333333333333333703, 0.3170188387650512141, 0.3333333333333333703, 0.3170188387650512141, 0.3333333333333333703, 0.3170188387650512141, 0.3333333333333333703, 0.3170188387650512141, 0.3333333333333333703, 0.3170188387650512141, 0.3333333333333333703, 0.3170188387650512141, 0.3333333333333333703, 0.3170188387650512141, 0.3333333333333333703, 0.3170188387650512141, 0.3333333333333333703, 0.3170188387650512141, 0.3333333333333333703, 0.3170188387650512141, 0.3333333333333333703, 0.3170188387650512141, 0.3333333333333333703, 0.3170188387650512141, 0.3333333333333333703, 0.3170188387650512141, 0.3333333333333333703, 0.3170188387650512141, 0.3333333333333333703, 0.3170188387650512141, 0.3333333333333333703, 0.3170188387650512141, 0.3333333333333333703, 0.3170188387650512141, 0.3333333333333333703, 0.3170188387650512141, 0.3333333333333333703, 0.3170188387650512141, 0.3333333333333333703, 0.3170188387650512141, 0.3333333333333333703, 0.3170188387650512141, 0.3333333333333333703, 0.3170188387650512141, 0.3333333333333333703, 0.3170188387650512141, 0.3333333333333333703, 0.3170188387650512141, 0.3333333333333333703, 0.3170188387650512141, 0.3333333333333333703, 0.3170188387650512141, 0.3333333333333333703, 0.3170188387650512141, 0.3333333333333333703, 0.3170188387650512141, 0.3333333333333333703, 0.3170188387650512141, 0.3333333333333333703, 0.3170188387650512141, 0.3333333333333333703, 0.3170188387650512141, 0.3333333333333333703, 0.3170188387650512141, 0.3333333333333333703, 0.3170188387650512141, 0.3333333333333333703, 0.3170188387650512141, 0.3333333333333333703, 0.3170188387650512141, 0.3333333333333333703, 0.3170188387650512141, 0.3333333333333333703, 0.3170188387650512141, 0.3333333333333333703, 0.3170188387650512141, 0.3333333333333333703, 0.3170188387650512141, 0.3333333333333333703, 0.3170188387650512141, 0.3333333333333333703, 0.3170188387650512141, 0.3333333333333333703, 0.3170188387650512141, 0.3333333333333333703, 0.3170188387650512141, 0.3333333333333333703, 0.3170188387650512141, 0.3333333333333333703, 0.3170188387650512141, 0.3333333333333333703, 0.3170188387650512141, 0.3333333333333333703, 0.3170188387650512141, 0.3333333333333333703, 0.3170188387650512141, 0.3333333333333333703, 0.3170188387650512141, 0.3333333333333333703, 0.3170188387650512141, 0.3333333333333333703, 0.3170188387650512141, 0.3333333333333333703, 0.3170188387650512141, 0.3333333333333333703, 0.3170188387650512141, 0.3333333333333333703, 0.3170188387650512141, 0.3333333333333333703, 0.3170188387650512141, 0.3333333333333333703, 0.3170188387650512141, 0.3333333333333333703, 0.3170188387650512141, 0.3333333333333333703, 0.3170188387650512141, 0.3333333333333333703, 0.3170188387650512141, 0.3333333333333333703, 0.3170188387650512141, 0.3333333333333333703, 0.3170188387650512141, 0.3333333333333333703, 0.3170188387650512141, 0.3333333333333333703, 0.3170188387650512141, 0.3333333333333333703, 0.3170188387650512141, 0.3333333333333333703, 0.3170188387650512141, 0.3333333333333333703, 0.3170188387650512141, 0.3333333333333333703, 0.3170188387650512141, 0.3333333333333333703, 0.3170188387650512141, 0.3333333333333333703, 0.3170188387650512141, 0.3333333333333333703, 0.3170188387650512141, 0.3333333333333333703, 0.3170188387650512141, 0.3333333333333333703, 0.3170188387650512141, 0.3333333333333333703, 0.3170188387650512141, 0.3333333333333333703, 0.3170188387650512141, 0.3333333333333333703, 0.3170188387650512141, 0.3333333333333333703, 0.3170188387650512141, 0.3333333333333333703, 0.3170188387650512141, 0.3333333333333333703, 0.3170188387650512141, 0.3333333333333333703, 0.3170188387650512141, 0.3333333333333333703, 0.3170188387650512141, 0.3333333333333333703, 0.3170188387650512141, 0.3333333333333333703, 0.3170188387650512141, 0.3333333333333333703, 0.3170188387650512141, 0.3333333333333333703, 0.3170188387650512141, 0.3333333333333333703, 0.3170188387650512141, 0.3333333333333333703, 0.3170188387650512141, 0.3333333333333333703),
 ( 0.3333333333333333703, 0.3170188387650512141, 0.3333333333333333703, 0.3170188387650512141, 0.3333333333333333703, 0.3170188387650512141, 0.3333333333333333703, 0.3170188387650512141, 0.3333333333333333703, 0.3170188387650512141, 0.3333333333333333703, 0.3170188387650512141, 0.3333333333333333703, 0.3170188387650512141, 0.3333333333333333703, 0.3170188387650512141, 0.3333333333333333703, 0.3170188387650512141, 0.3333333333333333703, 0.3170188387650512141, 0.3333333333333333703, 0.3170188387650512141, 0.3333333333333333703, 0.3170188387650512141, 0.3333333333333333703, 0.3170188387650512141, 0.3333333333333333703, 0.3170188387650512141, 0.3333333333333333703, 0.3170188387650512141, 0.3333333333333333703, 0.3170188387650512141, 0.3333333333333333703, 0.3170188387650512141, 0.3333333333333333703, 0.3170188387650512141, 0.3333333333333333703, 0.3170188387650512141, 0.3333333333333333703, 0.3170188387650512141, 0.3333333333333333703, 0.3170188387650512141, 0.3333333333333333703, 0.3170188387650512141, 0.3333333333333333703, 0.3170188387650512141, 0.3333333333333333703, 0.3170188387650512141, 0.3333333333333333703, 0.3170188387650512141, 0.3333333333333333703, 0.3170188387650512141, 0.3333333333333333703, 0.3170188387650512141, 0.3333333333333333703, 0.3170188387650512141, 0.3333333333333333703, 0.3170188387650512141, 0.3333333333333333703, 0.3170188387650512141, 0.3333333333333333703, 0.3170188387650512141, 0.3333333333333333703, 0.3170188387650512141, 0.3333333333333333703, 0.3170188387650512141, 0.3333333333333333703, 0.3170188387650512141, 0.3333333333333333703, 0.3170188387650512141, 0.3333333333333333703, 0.3170188387650512141, 0.3333333333333333703, 0.3170188387650512141, 0.3333333333333333703, 0.3170188387650512141, 0.3333333333333333703, 0.3170188387650512141, 0.3333333333333333703, 0.3170188387650512141, 0.3333333333333333703, 0.3170188387650512141, 0.3333333333333333703, 0.3170188387650512141, 0.3333333333333333703, 0.3170188387650512141, 0.3333333333333333703, 0.3170188387650512141, 0.3333333333333333703, 0.3170188387650512141, 0.3333333333333333703, 0.3170188387650512141, 0.3333333333333333703, 0.3170188387650512141, 0.3333333333333333703, 0.3170188387650512141, 0.3333333333333333703, 0.3170188387650512141, 0.3333333333333333703, 0.3170188387650512141, 0.3333333333333333703, 0.3170188387650512141, 0.3333333333333333703, 0.3170188387650512141, 0.3333333333333333703, 0.3170188387650512141, 0.3333333333333333703, 0.3170188387650512141, 0.3333333333333333703, 0.3170188387650512141, 0.3333333333333333703, 0.3170188387650512141, 0.3333333333333333703, 0.3170188387650512141, 0.3333333333333333703, 0.3170188387650512141, 0.3333333333333333703, 0.3170188387650512141, 0.3333333333333333703, 0.3170188387650512141, 0.3333333333333333703, 0.3170188387650512141, 0.3333333333333333703, 0.3170188387650512141, 0.3333333333333333703, 0.3170188387650512141, 0.3333333333333333703, 0.3170188387650512141, 0.3333333333333333703, 0.3170188387650512141, 0.3333333333333333703, 0.3170188387650512141, 0.3333333333333333703, 0.3170188387650512141, 0.3333333333333333703, 0.3170188387650512141, 0.3333333333333333703, 0.3170188387650512141, 0.3333333333333333703, 0.3170188387650512141, 0.3333333333333333703, 0.3170188387650512141, 0.3333333333333333703, 0.3170188387650512141, 0.3333333333333333703, 0.3170188387650512141, 0.3333333333333333703, 0.3170188387650512141, 0.3333333333333333703, 0.3170188387650512141, 0.3333333333333333703, 0.3170188387650512141, 0.3333333333333333703, 0.3170188387650512141, 0.3333333333333333703, 0.3170188387650512141, 0.3333333333333333703, 0.3170188387650512141, 0.3333333333333333703, 0.3170188387650512141, 0.3333333333333333703, 0.3170188387650512141, 0.3333333333333333703, 0.3170188387650512141, 0.3333333333333333703, 0.3170188387650512141, 0.3333333333333333703, 0.3170188387650512141, 0.3333333333333333703, 0.3170188387650512141, 0.3333333333333333703, 0.3170188387650512141, 0.3333333333333333703, 0.3170188387650512141, 0.3333333333333333703, 0.3170188387650512141, 0.3333333333333333703, 0.3170188387650512141, 0.3333333333333333703, 0.3170188387650512141, 0.3333333333333333703, 0.3170188387650512141, 0.3333333333333333703, 0.3170188387650512141, 0.3333333333333333703, 0.3170188387650512141, 0.3333333333333333703, 0.3170188387650512141, 0.3333333333333333703, 0.3170188387650512141, 0.3333333333333333703, 0.3170188387650512141, 0.3333333333333333703, 0.3170188387650512141, 0.3333333333333333703, 0.3170188387650512141, 0.3333333333333333703, 0.3170188387650512141, 0.3333333333333333703, 0.3170188387650512141, 0.3333333333333333703),
 ( 1.000000000000000000, 0.9510565162951535312, 1.000000000000000000, 0.9510565162951535312, 1.000000000000000000, 0.9510565162951535312, 1.000000000000000000, 0.9510565162951535312, 1.000000000000000000, 0.9510565162951535312, 1.000000000000000000, 0.9510565162951535312, 1.000000000000000000, 0.9510565162951535312, 1.000000000000000000, 0.9510565162951535312, 1.000000000000000000, 0.9510565162951535312, 1.000000000000000000, 0.9510565162951535312, 1.000000000000000000, 0.9510565162951535312, 1.000000000000000000, 0.9510565162951535312, 1.000000000000000000, 0.9510565162951535312, 1.000000000000000000, 0.9510565162951535312, 1.000000000000000000, 0.9510565162951535312, 1.000000000000000000, 0.9510565162951535312, 1.000000000000000000, 0.9510565162951535312, 1.000000000000000000, 0.9510565162951535312, 1.000000000000000000, 0.9510565162951535312, 1.000000000000000000, 0.9510565162951535312, 1.000000000000000000, 0.9510565162951535312, 1.000000000000000000, 0.9510565162951535312, 1.000000000000000000, 0.9510565162951535312, 1.000000000000000000, 0.9510565162951535312, 1.000000000000000000, 0.9510565162951535312, 1.000000000000000000, 0.9510565162951535312, 1.000000000000000000, 0.9510565162951535312, 1.000000000000000000, 0.9510565162951535312, 1.000000000000000000, 0.9510565162951535312, 1.000000000000000000, 0.9510565162951535312, 1.000000000000000000, 0.9510565162951535312, 1.000000000000000000, 0.9510565162951535312, 1.000000000000000000, 0.9510565162951535312, 1.000000000000000000, 0.9510565162951535312, 1.000000000000000000, 0.9510565162951535312, 1.000000000000000000, 0.9510565162951535312, 1.000000000000000000, 0.9510565162951535312, 1.000000000000000000, 0.9510565162951535312, 1.000000000000000000, 0.9510565162951535312, 1.000000000000000000, 0.9510565162951535312, 1.000000000000000000, 0.9510565162951535312, 1.000000000000000000, 0.9510565162951535312, 1.000000000000000000, 0.9510565162951535312, 1.000000000000000000, 0.9510565162951535312, 1.000000000000000000, 0.9510565162951535312, 1.000000000000000000, 0.9510565162951535312, 1.000000000000000000, 0.9510565162951535312, 1.000000000000000000, 0.9510565162951535312, 1.000000000000000000, 0.9510565162951535312, 1.000000000000000000, 0.9510565162951535312, 1.000000000000000000, 0.9510565162951535312, 1.000000000000000000, 0.9510565162951535312, 1.000000000000000000, 0.9510565162951535312, 1.000000000000000000, 0.9510565162951535312, 1.000000000000000000, 0.9510565162951535312, 1.000000000000000000, 0.9510565162951535312, 1.000000000000000000, 0.9510565162951535312, 1.000000000000000000, 0.9510565162951535312, 1.000000000000000000, 0.9510565162951535312, 1.000000000000000000, 0.9510565162951535312, 1.000000000000000000, 0.9510565162951535312, 1.000000000000000000, 0.9510565162951535312, 1.000000000000000000, 0.9510565162951535312, 1.000000000000000000, 0.9510565162951535312, 1.000000000000000000, 0.9510565162951535312, 1.000000000000000000, 0.9510565162951535312, 1.000000000000000000, 0.9510565162951535312, 1.000000000000000000, 0.9510565162951535312, 1.000000000000000000, 0.9510565162951535312, 1.000000000000000000, 0.9510565162951535312, 1.000000000000000000, 0.9510565162951535312, 1.000000000000000000, 0.9510565162951535312, 1.000000000000000000, 0.9510565162951535312, 1.000000000000000000, 0.9510565162951535312, 1.000000000000000000, 0.9510565162951535312, 1.000000000000000000, 0.9510565162951535312, 1.000000000000000000, 0.9510565162951535312, 1.000000000000000000, 0.9510565162951535312, 1.000000000000000000, 0.9510565162951535312, 1.000000000000000000, 0.9510565162951535312, 1.000000000000000000, 0.9510565162951535312, 1.000000000000000000, 0.9510565162951535312, 1.000000000000000000, 0.9510565162951535312, 1.000000000000000000, 0.9510565162951535312, 1.000000000000000000, 0.9510565162951535312, 1.000000000000000000, 0.9510565162951535312, 1.000000000000000000, 0.9510565162951535312, 1.000000000000000000, 0.9510565162951535312, 1.000000000000000000, 0.9510565162951535312, 1.000000000000000000, 0.9510565162951535312, 1.000000000000000000, 0.9510565162951535312, 1.000000000000000000, 0.9510565162951535312, 1.000000000000000000, 0.9510565162951535312, 1.000000000000000000, 0.9510565162951535312, 1.000000000000000000, 0.9510565162951535312, 1.000000000000000000, 0.9510565162951535312, 1.000000000000000000, 0.9510565162951535312, 1.000000000000000000, 0.9510565162951535312, 1.000000000000000000, 0.9510565162951535312, 1.000000000000000000, 0.9510565162951535312, 1.000000000000000000),
 ( 0.3333333333333333703, 0.3170188387650512141, 0.3333333333333333703, 0.3170188387650512141, 0.3333333333333333703, 0.3170188387650512141, 0.3333333333333333703, 0.3170188387650512141, 0.3333333333333333703, 0.3170188387650512141, 0.3333333333333333703, 0.3170188387650512141, 0.3333333333333333703, 0.3170188387650512141, 0.3333333333333333703, 0.3170188387650512141, 0.3333333333333333703, 0.3170188387650512141, 0.3333333333333333703, 0.3170188387650512141, 0.3333333333333333703, 0.3170188387650512141, 0.3333333333333333703, 0.3170188387650512141, 0.3333333333333333703, 0.3170188387650512141, 0.3333333333333333703, 0.3170188387650512141, 0.3333333333333333703, 0.3170188387650512141, 0.3333333333333333703, 0.3170188387650512141, 0.3333333333333333703, 0.3170188387650512141, 0.3333333333333333703, 0.3170188387650512141, 0.3333333333333333703, 0.3170188387650512141, 0.3333333333333333703, 0.3170188387650512141, 0.3333333333333333703, 0.3170188387650512141, 0.3333333333333333703, 0.3170188387650512141, 0.3333333333333333703, 0.3170188387650512141, 0.3333333333333333703, 0.3170188387650512141, 0.3333333333333333703, 0.3170188387650512141, 0.3333333333333333703, 0.3170188387650512141, 0.3333333333333333703, 0.3170188387650512141, 0.3333333333333333703, 0.3170188387650512141, 0.3333333333333333703, 0.3170188387650512141, 0.3333333333333333703, 0.3170188387650512141, 0.3333333333333333703, 0.3170188387650512141, 0.3333333333333333703, 0.3170188387650512141, 0.3333333333333333703, 0.3170188387650512141, 0.3333333333333333703, 0.3170188387650512141, 0.3333333333333333703, 0.3170188387650512141, 0.3333333333333333703, 0.3170188387650512141, 0.3333333333333333703, 0.3170188387650512141, 0.3333333333333333703, 0.3170188387650512141, 0.3333333333333333703, 0.3170188387650512141, 0.3333333333333333703, 0.3170188387650512141, 0.3333333333333333703, 0.3170188387650512141, 0.3333333333333333703, 0.3170188387650512141, 0.3333333333333333703, 0.3170188387650512141, 0.3333333333333333703, 0.3170188387650512141, 0.3333333333333333703, 0.3170188387650512141, 0.3333333333333333703, 0.3170188387650512141, 0.3333333333333333703, 0.3170188387650512141, 0.3333333333333333703, 0.3170188387650512141, 0.3333333333333333703, 0.3170188387650512141, 0.3333333333333333703, 0.3170188387650512141, 0.3333333333333333703, 0.3170188387650512141, 0.3333333333333333703, 0.3170188387650512141, 0.3333333333333333703, 0.3170188387650512141, 0.3333333333333333703, 0.3170188387650512141, 0.3333333333333333703, 0.3170188387650512141, 0.3333333333333333703, 0.3170188387650512141, 0.3333333333333333703, 0.3170188387650512141, 0.3333333333333333703, 0.3170188387650512141, 0.3333333333333333703, 0.3170188387650512141, 0.3333333333333333703, 0.3170188387650512141, 0.3333333333333333703, 0.3170188387650512141, 0.3333333333333333703, 0.3170188387650512141, 0.3333333333333333703, 0.3170188387650512141, 0.3333333333333333703, 0.3170188387650512141, 0.3333333333333333703, 0.3170188387650512141, 0.3333333333333333703, 0.3170188387650512141, 0.3333333333333333703, 0.3170188387650512141, 0.3333333333333333703, 0.3170188387650512141, 0.3333333333333333703, 0.3170188387650512141, 0.3333333333333333703, 0.3170188387650512141, 0.3333333333333333703, 0.3170188387650512141, 0.3333333333333333703, 0.3170188387650512141, 0.3333333333333333703, 0.3170188387650512141, 0.3333333333333333703, 0.3170188387650512141, 0.3333333333333333703, 0.3170188387650512141, 0.3333333333333333703, 0.3170188387650512141, 0.3333333333333333703, 0.3170188387650512141, 0.3333333333333333703, 0.3170188387650512141, 0.3333333333333333703, 0.3170188387650512141, 0.3333333333333333703, 0.3170188387650512141, 0.3333333333333333703, 0.3170188387650512141, 0.3333333333333333703, 0.3170188387650512141, 0.3333333333333333703, 0.3170188387650512141, 0.3333333333333333703, 0.3170188387650512141, 0.3333333333333333703, 0.3170188387650512141, 0.3333333333333333703, 0.3170188387650512141, 0.3333333333333333703, 0.3170188387650512141, 0.3333333333333333703, 0.3170188387650512141, 0.3333333333333333703, 0.3170188387650512141, 0.3333333333333333703, 0.3170188387650512141, 0.3333333333333333703, 0.3170188387650512141, 0.3333333333333333703, 0.3170188387650512141, 0.3333333333333333703, 0.3170188387650512141, 0.3333333333333333703, 0.3170188387650512141, 0.3333333333333333703, 0.3170188387650512141, 0.3333333333333333703, 0.3170188387650512141, 0.3333333333333333703, 0.3170188387650512141, 0.3333333333333333703, 0.3170188387650512141, 0.3333333333333333703, 0.3170188387650512141, 0.3333333333333333703, 0.3170188387650512141, 0.3333333333333333703),
 ( 0.3333333333333333703, 0.3170188387650512141, 0.3333333333333333703, 0.3170188387650512141, 0.3333333333333333703, 0.3170188387650512141, 0.3333333333333333703, 0.3170188387650512141, 0.3333333333333333703, 0.3170188387650512141, 0.3333333333333333703, 0.3170188387650512141, 0.3333333333333333703, 0.3170188387650512141, 0.3333333333333333703, 0.3170188387650512141, 0.3333333333333333703, 0.3170188387650512141, 0.3333333333333333703, 0.3170188387650512141, 0.3333333333333333703, 0.3170188387650512141, 0.3333333333333333703, 0.3170188387650512141, 0.3333333333333333703, 0.3170188387650512141, 0.3333333333333333703, 0.3170188387650512141, 0.3333333333333333703, 0.3170188387650512141, 0.3333333333333333703, 0.3170188387650512141, 0.3333333333333333703, 0.3170188387650512141, 0.3333333333333333703, 0.3170188387650512141, 0.3333333333333333703, 0.3170188387650512141, 0.3333333333333333703, 0.3170188387650512141, 0.3333333333333333703, 0.3170188387650512141, 0.3333333333333333703, 0.3170188387650512141, 0.3333333333333333703, 0.3170188387650512141, 0.3333333333333333703, 0.3170188387650512141, 0.3333333333333333703, 0.3170188387650512141, 0.3333333333333333703, 0.3170188387650512141, 0.3333333333333333703, 0.3170188387650512141, 0.3333333333333333703, 0.3170188387650512141, 0.3333333333333333703, 0.3170188387650512141, 0.3333333333333333703, 0.3170188387650512141, 0.3333333333333333703, 0.3170188387650512141, 0.3333333333333333703, 0.3170188387650512141, 0.3333333333333333703, 0.3170188387650512141, 0.3333333333333333703, 0.3170188387650512141, 0.3333333333333333703, 0.3170188387650512141, 0.3333333333333333703, 0.3170188387650512141, 0.3333333333333333703, 0.3170188387650512141, 0.3333333333333333703, 0.3170188387650512141, 0.3333333333333333703, 0.3170188387650512141, 0.3333333333333333703, 0.3170188387650512141, 0.3333333333333333703, 0.3170188387650512141, 0.3333333333333333703, 0.3170188387650512141, 0.3333333333333333703, 0.3170188387650512141, 0.3333333333333333703, 0.3170188387650512141, 0.3333333333333333703, 0.3170188387650512141, 0.3333333333333333703, 0.3170188387650512141, 0.3333333333333333703, 0.3170188387650512141, 0.3333333333333333703, 0.3170188387650512141, 0.3333333333333333703, 0.3170188387650512141, 0.3333333333333333703, 0.3170188387650512141, 0.3333333333333333703, 0.3170188387650512141, 0.3333333333333333703, 0.3170188387650512141, 0.3333333333333333703, 0.3170188387650512141, 0.3333333333333333703, 0.3170188387650512141, 0.3333333333333333703, 0.3170188387650512141, 0.3333333333333333703, 0.3170188387650512141, 0.3333333333333333703, 0.3170188387650512141, 0.3333333333333333703, 0.3170188387650512141, 0.3333333333333333703, 0.3170188387650512141, 0.3333333333333333703, 0.3170188387650512141, 0.3333333333333333703, 0.3170188387650512141, 0.3333333333333333703, 0.3170188387650512141, 0.3333333333333333703, 0.3170188387650512141, 0.3333333333333333703, 0.3170188387650512141, 0.3333333333333333703, 0.3170188387650512141, 0.3333333333333333703, 0.3170188387650512141, 0.3333333333333333703, 0.3170188387650512141, 0.3333333333333333703, 0.3170188387650512141, 0.3333333333333333703, 0.3170188387650512141, 0.3333333333333333703, 0.3170188387650512141, 0.3333333333333333703, 0.3170188387650512141, 0.3333333333333333703, 0.3170188387650512141, 0.3333333333333333703, 0.3170188387650512141, 0.3333333333333333703, 0.3170188387650512141, 0.3333333333333333703, 0.3170188387650512141, 0.3333333333333333703, 0.3170188387650512141, 0.3333333333333333703, 0.3170188387650512141, 0.3333333333333333703, 0.3170188387650512141, 0.3333333333333333703, 0.3170188387650512141, 0.3333333333333333703, 0.3170188387650512141, 0.3333333333333333703, 0.3170188387650512141, 0.3333333333333333703, 0.3170188387650512141, 0.3333333333333333703, 0.3170188387650512141, 0.3333333333333333703, 0.3170188387650512141, 0.3333333333333333703, 0.3170188387650512141, 0.3333333333333333703, 0.3170188387650512141, 0.3333333333333333703, 0.3170188387650512141, 0.3333333333333333703, 0.3170188387650512141, 0.3333333333333333703, 0.3170188387650512141, 0.3333333333333333703, 0.3170188387650512141, 0.3333333333333333703, 0.3170188387650512141, 0.3333333333333333703, 0.3170188387650512141, 0.3333333333333333703, 0.3170188387650512141, 0.3333333333333333703, 0.3170188387650512141, 0.3333333333333333703, 0.3170188387650512141, 0.3333333333333333703, 0.3170188387650512141, 0.3333333333333333703, 0.3170188387650512141, 0.3333333333333333703, 0.3170188387650512141, 0.3333333333333333703, 0.3170188387650512141, 0.3333333333333333703, 0.3170188387650512141, 0.3333333333333333703),
 ( 1.000000000000000000, 0.9510565162951535312, 1.000000000000000000, 0.9510565162951535312, 1.000000000000000000, 0.9510565162951535312, 1.000000000000000000, 0.9510565162951535312, 1.000000000000000000, 0.9510565162951535312, 1.000000000000000000, 0.9510565162951535312, 1.000000000000000000, 0.9510565162951535312, 1.000000000000000000, 0.9510565162951535312, 1.000000000000000000, 0.9510565162951535312, 1.000000000000000000, 0.9510565162951535312, 1.000000000000000000, 0.9510565162951535312, 1.000000000000000000, 0.9510565162951535312, 1.000000000000000000, 0.9510565162951535312, 1.000000000000000000, 0.9510565162951535312, 1.000000000000000000, 0.9510565162951535312, 1.000000000000000000, 0.9510565162951535312, 1.000000000000000000, 0.9510565162951535312, 1.000000000000000000, 0.9510565162951535312, 1.000000000000000000, 0.9510565162951535312, 1.000000000000000000, 0.9510565162951535312, 1.000000000000000000, 0.9510565162951535312, 1.000000000000000000, 0.9510565162951535312, 1.000000000000000000, 0.9510565162951535312, 1.000000000000000000, 0.9510565162951535312, 1.000000000000000000, 0.9510565162951535312, 1.000000000000000000, 0.9510565162951535312, 1.000000000000000000, 0.9510565162951535312, 1.000000000000000000, 0.9510565162951535312, 1.000000000000000000, 0.9510565162951535312, 1.000000000000000000, 0.9510565162951535312, 1.000000000000000000, 0.9510565162951535312, 1.000000000000000000, 0.9510565162951535312, 1.000000000000000000, 0.9510565162951535312, 1.000000000000000000, 0.9510565162951535312, 1.000000000000000000, 0.9510565162951535312, 1.000000000000000000, 0.9510565162951535312, 1.000000000000000000, 0.9510565162951535312, 1.000000000000000000, 0.9510565162951535312, 1.000000000000000000, 0.9510565162951535312, 1.000000000000000000, 0.9510565162951535312, 1.000000000000000000, 0.9510565162951535312, 1.000000000000000000, 0.9510565162951535312, 1.000000000000000000, 0.9510565162951535312, 1.000000000000000000, 0.9510565162951535312, 1.000000000000000000, 0.9510565162951535312, 1.000000000000000000, 0.9510565162951535312, 1.000000000000000000, 0.9510565162951535312, 1.000000000000000000, 0.9510565162951535312, 1.000000000000000000, 0.9510565162951535312, 1.000000000000000000, 0.9510565162951535312, 1.000000000000000000, 0.9510565162951535312, 1.000000000000000000, 0.9510565162951535312, 1.000000000000000000, 0.9510565162951535312, 1.000000000000000000, 0.9510565162951535312, 1.000000000000000000, 0.9510565162951535312, 1.000000000000000000, 0.9510565162951535312, 1.000000000000000000, 0.9510565162951535312, 1.000000000000000000, 0.9510565162951535312, 1.000000000000000000, 0.9510565162951535312, 1.000000000000000000, 0.9510565162951535312, 1.000000000000000000, 0.9510565162951535312, 1.000000000000000000, 0.9510565162951535312, 1.000000000000000000, 0.9510565162951535312, 1.000000000000000000, 0.9510565162951535312, 1.000000000000000000, 0.9510565162951535312, 1.000000000000000000, 0.9510565162951535312, 1.000000000000000000, 0.9510565162951535312, 1.000000000000000000, 0.9510565162951535312, 1.000000000000000000, 0.9510565162951535312, 1.000000000000000000, 0.9510565162951535312, 1.000000000000000000, 0.9510565162951535312, 1.000000000000000000, 0.9510565162951535312, 1.000000000000000000, 0.9510565162951535312, 1.000000000000000000, 0.9510565162951535312, 1.000000000000000000, 0.9510565162951535312, 1.000000000000000000, 0.9510565162951535312, 1.000000000000000000, 0.9510565162951535312, 1.000000000000000000, 0.9510565162951535312, 1.000000000000000000, 0.9510565162951535312, 1.000000000000000000, 0.9510565162951535312, 1.000000000000000000, 0.9510565162951535312, 1.000000000000000000, 0.9510565162951535312, 1.000000000000000000, 0.9510565162951535312, 1.000000000000000000, 0.9510565162951535312, 1.000000000000000000, 0.9510565162951535312, 1.000000000000000000, 0.9510565162951535312, 1.000000000000000000, 0.9510565162951535312, 1.000000000000000000, 0.9510565162951535312, 1.000000000000000000, 0.9510565162951535312, 1.000000000000000000, 0.9510565162951535312, 1.000000000000000000, 0.9510565162951535312, 1.000000000000000000, 0.9510565162951535312, 1.000000000000000000, 0.9510565162951535312, 1.000000000000000000, 0.9510565162951535312, 1.000000000000000000, 0.9510565162951535312, 1.000000000000000000, 0.9510565162951535312, 1.000000000000000000, 0.9510565162951535312, 1.000000000000000000, 0.9510565162951535312, 1.000000000000000000, 0.9510565162951535312, 1.000000000000000000, 0.9510565162951535312, 1.000000000000000000) ) ) 
 REPRESENTATION_ITEM ( '' )  SURFACE ( )  );
#11092=CARTESIAN_POINT ( 'NONE',  ( -3.673772985318219053, 18.24680007765647716, -2.599342558260952174 ) ) ;
#11094=CARTESIAN_POINT ( 'NONE',  ( 2.518350579753611207, 28.12819992234355126, -0.7558219633769606149 ) ) ;
#11097=CARTESIAN_POINT ( 'NONE',  ( 0.05938372350929014415, 27.37180007765647716, 4.731580009072201776 ) ) ;
#11113=CARTESIAN_POINT ( 'NONE',  ( -2.864755990943222308, 34.25319992234354771, 2.011557305968548093 ) ) ;
#11114=CARTESIAN_POINT ( 'NONE',  ( -3.481649420246394566, 17.12819992234353705, -1.193696214020467883 ) ) ;
#11116=CARTESIAN_POINT ( 'NONE',  ( 2.500000000000001332, 29.24680007765648071, -0.05647727720535888202 ) ) ;
#11118=CARTESIAN_POINT ( 'NONE',  ( -4.499999999999999112, 22.00319992234354061, -0.05647727720528529505 ) ) ;
#11124=CARTESIAN_POINT ( 'NONE',  ( 1.027846397803542144, 23.74680007765647716, -3.346150245485522312 ) ) ;
#11139=CARTESIAN_POINT ( 'NONE',  ( -2.055738996568281518, 34.25319992234354061, 1.423772053676066962 ) ) ;
#11141=CARTESIAN_POINT ( 'NONE',  ( -2.211161402132902243, 30.87180007765647716, -2.942372952327172886 ) ) ;
#11142=CARTESIAN_POINT ( 'NONE',  ( 1.135272562821020070, 30.25319992234354416, -3.311245368580577164 ) ) ;
#11154=CARTESIAN_POINT ( 'NONE',  ( 1.497042530366522461, 16.12819992234354416, 2.161531897785029965 ) ) ;
#11156=CARTESIAN_POINT ( 'NONE',  ( -2.864755990943265829, 35.74680007765648071, -2.011557305968488141 ) ) ;
#11161=CARTESIAN_POINT ( 'NONE',  ( 2.115076519116362963, 31.37180007765647716, -3.012182706137107147 ) ) ;
#11175=CARTESIAN_POINT ( 'NONE',  ( -0.05938372350927861171, 38.62180007765648071, -3.680117784833935701 ) ) ;
#11180=CARTESIAN_POINT ( 'NONE',  ( 1.444289557196047680, 17.24680007765648071, 4.262301884875704161 ) ) ;
#11182=CARTESIAN_POINT ( 'NONE',  ( 0.7188294034286553114, 36.25319992234354771, 2.395093729190349130 ) ) ;
#11185=CARTESIAN_POINT ( 'NONE',  ( 1.444289557196047680, 29.74680007765648071, 4.262301884875704161 ) ) ;
#11203=SURFACE_SIDE_STYLE ('',( #5555 ) ) ;
#11204=CARTESIAN_POINT ( 'NONE',  ( 3.673772985318163098, 20.50319992234354771, -2.599342558261029001 ) ) ;
#11205=CARTESIAN_POINT ( 'NONE',  ( 0.05938372350920110426, 17.62819992234354771, -3.680117784833935701 ) ) ;
#11208=CARTESIAN_POINT ( 'NONE',  ( 2.518350579753628971, 36.87180007765648071, 0.7558219633769073242 ) ) ;
#11209=CARTESIAN_POINT ( 'NONE',  ( 2.829195390882724759, 27.87819992234354416, -3.793023760679264278 ) ) ;
#11213=CARTESIAN_POINT ( 'NONE',  ( 2.115076519116362963, 18.87180007765648071, -3.012182706137107147 ) ) ;
#11224=CARTESIAN_POINT ( 'NONE',  ( 3.481649420246369697, 24.12180007765648071, -1.193696214020541824 ) ) ;
#11230=CARTESIAN_POINT ( 'NONE',  ( 3.481649420246394122, 15.87819992234354594, 1.193696214020467439 ) ) ;
#11232=CARTESIAN_POINT ( 'NONE',  ( 3.518350579753631191, 31.87180007765647716, 1.080741659609802285 ) ) ;
#11234=CARTESIAN_POINT ( 'NONE',  ( 2.798362969681409851, 26.00319992234354771, 2.102939460078764977 ) ) ;
#11249=CARTESIAN_POINT ( 'NONE',  ( -1.593127413382998459, 38.37180007765647360, -2.091722143975139669 ) ) ;
#11256=CARTESIAN_POINT ( 'NONE',  ( 3.518350579753631191, 31.87180007765647716, 1.080741659609802285 ) ) ;
#11267=CARTESIAN_POINT ( 'NONE',  ( 2.211161402132902243, 39.62180007765646650, 2.942372952327172442 ) ) ;
#11273=CARTESIAN_POINT ( 'NONE',  ( -2.500000000000001332, 37.00319992234354771, -0.05647727720530596601 ) ) ;
#11276=CARTESIAN_POINT ( 'NONE',  ( -4.481649420246366589, 35.37180007765647360, 1.518615910253458878 ) ) ;
#11290=CARTESIAN_POINT ( 'NONE',  ( 4.481649420246397675, 18.37819992234354416, 1.518615910253363177 ) ) ;
#11291=CARTESIAN_POINT ( 'NONE',  ( 2.211161402132839182, 22.87819992234354416, -2.942372952327217739 ) ) ;
#11293=CARTESIAN_POINT ( 'NONE',  ( -1.497042530366477164, 40.12180007765647360, 2.161531897785062384 ) ) ;
#11294=CARTESIAN_POINT ( 'NONE',  ( -3.607379964056363075, 32.25319992234354061, -2.690724712371229899 ) ) ;
#11300=CARTESIAN_POINT ( 'NONE',  ( -3.500000000000000444, 20.49680007765647716, 0.05647727720536892260 ) ) ;
#11304=CARTESIAN_POINT ( 'NONE',  ( -0.05938372350928957516, 26.12180007765648426, -4.731580009072201776 ) ) ;
#11310=CARTESIAN_POINT ( 'NONE',  ( -1.135272562821090014, 25.99680007765648071, -3.311245368580554072 ) ) ;
#11317=CARTESIAN_POINT ( 'NONE',  ( -2.211161402132839182, 21.62819992234354771, 2.942372952327218627 ) ) ;
#11319=CARTESIAN_POINT ( 'NONE',  ( 1.497042530366477164, 16.37180007765648426, -2.161531897785062384 ) ) ;
#11320=CARTESIAN_POINT ( 'NONE',  ( 2.211161402132839626, 35.37819992234353350, -2.942372952327218183 ) ) ;
#11331=CARTESIAN_POINT ( 'NONE',  ( -1.318039840154427544, 15.00000000000000178, -3.027868313707952730 ) ) ;
#11333=CARTESIAN_POINT ( 'NONE',  ( 2.055738996568281518, 23.00319992234354771, -1.423772053676066518 ) ) ;
#11335=CARTESIAN_POINT ( 'NONE',  ( -2.864755990943265829, 18.24680007765648071, -2.011557305968488141 ) ) ;
#11342=CARTESIAN_POINT ( 'NONE',  ( 3.500000000000000444, 29.24680007765647716, -0.05647727720536935281 ) ) ;
#11347=DIRECTION ( 'NONE',  ( 0.000000000000000000, 1.000000000000000000, 0.000000000000000000 ) ) ;
#11355=CARTESIAN_POINT ( 'NONE',  ( -1.497042530366477164, 25.12180007765648071, 2.161531897785062384 ) ) ;
#11360=CARTESIAN_POINT ( 'NONE',  ( -0.8262555684460826111, 36.50319992234354061, 2.360188852285421302 ) ) ;
#11363=CARTESIAN_POINT ( 'NONE',  ( -1.444289557196047014, 30.99680007765647716, -4.262301884875704161 ) ) ;
#11380=CARTESIAN_POINT ( 'NONE',  ( -1.444289557195956863, 19.00319992234354771, 4.262301884875733471 ) ) ;
#11381=CARTESIAN_POINT ( 'NONE',  ( -0.05938372350920064630, 31.37819992234354416, 3.680117784833935701 ) ) ;
#11383=CARTESIAN_POINT ( 'NONE',  ( 1.497042530366477164, 36.37180007765648071, -2.161531897785062384 ) ) ;
#11384=CARTESIAN_POINT ( 'NONE',  ( -2.733110507866328476, 37.37819992234354771, -3.862833514489096398 ) ) ;
#11388=CARTESIAN_POINT ( 'NONE',  ( -1.027846397803541700, 24.99680007765647716, 3.346150245485522312 ) ) ;
#11391=CARTESIAN_POINT ( 'NONE',  ( 3.673772985318219053, 29.49680007765647360, 2.599342558260951730 ) ) ;
#11396=CARTESIAN_POINT ( 'NONE',  ( 0.05938372350927906274, 22.37180007765648071, 3.680117784833935701 ) ) ;
#11401=CARTESIAN_POINT ( 'NONE',  ( -1.027846397803611866, 17.50319992234354416, -3.346150245485499219 ) ) ;
#11403=CARTESIAN_POINT ( 'NONE',  ( -1.027846397803541700, 37.49680007765647360, 3.346150245485522312 ) ) ;
#11405=CARTESIAN_POINT ( 'NONE',  ( -2.211161402132839182, 36.62819992234354771, 2.942372952327218627 ) ) ;
#11420=CARTESIAN_POINT ( 'NONE',  ( 2.518350579753611207, 20.62819992234354771, -0.7558219633769606149 ) ) ;
#11423=CARTESIAN_POINT ( 'NONE',  ( -2.864755990943265829, 15.74680007765647716, -2.011557305968488141 ) ) ;
#11428=CARTESIAN_POINT ( 'NONE',  ( 3.500000000000000444, 31.74680007765647716, -0.05647727720536935281 ) ) ;
#11441=CARTESIAN_POINT ( 'NONE',  ( 0.8262555684461332373, 22.24680007765648071, 2.360188852285403982 ) ) ;
#11443=CARTESIAN_POINT ( 'NONE',  ( 2.864755990943265829, 21.99680007765647716, 2.011557305968487697 ) ) ;
#11448=CARTESIAN_POINT ( 'NONE',  ( 2.055738996568281518, 38.00319992234354061, -1.423772053676066518 ) ) ;
#11451=CARTESIAN_POINT ( 'NONE',  ( 1.444289557196047680, 34.74680007765647360, 4.262301884875704161 ) ) ;
#11469=CARTESIAN_POINT ( 'NONE',  ( -1.444289557195956863, 16.50319992234354416, 4.262301884875733471 ) ) ;
#11470=CARTESIAN_POINT ( 'NONE',  ( -3.518350579753606322, 31.87819992234354416, 1.080741659609877781 ) ) ;
#11471=CARTESIAN_POINT ( 'NONE',  ( -2.481649420246374138, 40.37180007765647360, 0.8687765177876256573 ) ) ;
#11474=CARTESIAN_POINT ( 'NONE',  ( -3.673772985318163098, 34.25319992234354061, 2.599342558261029001 ) ) ;
#11480=CARTESIAN_POINT ( 'NONE',  ( -3.481649420246369697, 27.87180007765647360, 1.193696214020542490 ) ) ;
#11483=CARTESIAN_POINT ( 'NONE',  ( 4.481649420246366589, 34.12180007765647360, -1.518615910253458212 ) ) ;
#11489=CARTESIAN_POINT ( 'NONE',  ( 0.05938372350927906274, 24.87180007765647005, 3.680117784833935701 ) ) ;
#11494=CARTESIAN_POINT ( 'NONE',  ( 1.135272562821020070, 17.75319992234354771, -3.311245368580577164 ) ) ;
#11497=CARTESIAN_POINT ( 'NONE',  ( 2.211161402132902243, 39.62180007765646650, 2.942372952327172442 ) ) ;
#11498=CARTESIAN_POINT ( 'NONE',  ( 0.05938372350920109732, 35.12819992234354771, -3.680117784833935701 ) ) ;
#11513=CARTESIAN_POINT ( 'NONE',  ( -1.158310996484859468, 15.00000000000000533, -3.163418999597361836 ) ) ;
#11517=CARTESIAN_POINT ( 'NONE',  ( 2.481649420246391902, 18.37819992234354416, 0.8687765177875720335 ) ) ;
#11520=CARTESIAN_POINT ( 'NONE',  ( -2.798362969681365886, 17.74680007765647716, 2.102939460078824929 ) ) ;
#11521=CARTESIAN_POINT ( 'NONE',  ( 1.336863392178479160, 18.74680007765647005, -4.297206761780677731 ) ) ;
#11525=CARTESIAN_POINT ( 'NONE',  ( -2.211161402132902243, 30.87180007765647716, -2.942372952327172886 ) ) ;
#11536=CARTESIAN_POINT ( 'NONE',  ( -2.481649420246374138, 20.37180007765648426, 0.8687765177876256573 ) ) ;
#11539=CARTESIAN_POINT ( 'NONE',  ( 3.518350579753631191, 24.37180007765647716, 1.080741659609802729 ) ) ;
#11544=CARTESIAN_POINT ( 'NONE',  ( 2.055738996568281518, 35.50319992234354771, -1.423772053676066518 ) ) ;
#11547=CARTESIAN_POINT ( 'NONE',  ( -0.05938372350928957516, 31.12180007765647716, -4.731580009072201776 ) ) ;
#11563=CARTESIAN_POINT ( 'NONE',  ( -3.673772985318163098, 21.75319992234354416, 2.599342558261029001 ) ) ;
#11564=CARTESIAN_POINT ( 'NONE',  ( -1.135272562821019626, 29.00319992234354416, 3.311245368580577164 ) ) ;
#11565=CARTESIAN_POINT ( 'NONE',  ( 2.481649420246391902, 15.87819992234354771, 0.8687765177875720335 ) ) ;
#11568=CARTESIAN_POINT ( 'NONE',  ( -0.05938372350918959958, 36.37819992234354771, 4.731580009072201776 ) ) ;
#11574=CARTESIAN_POINT ( 'NONE',  ( 1.027846397803542144, 33.74680007765648071, -3.346150245485522312 ) ) ;
#11578=CARTESIAN_POINT ( 'NONE',  ( -4.499999999999999112, 32.99680007765648071, 0.05647727720537927543 ) ) ;
#11583=CARTESIAN_POINT ( 'NONE',  ( -3.518350579753630747, 20.62180007765646650, -1.080741659609802729 ) ) ;
#11589=CARTESIAN_POINT ( 'NONE',  ( 0.05938372350920109732, 22.62819992234354416, -3.680117784833935701 ) ) ;
#11592=CARTESIAN_POINT ( 'NONE',  ( -0.05938372350927861171, 38.62180007765648071, -3.680117784833935701 ) ) ;
#11594=CARTESIAN_POINT ( 'NONE',  ( 1.135272562821020070, 32.75319992234354771, -3.311245368580577164 ) ) ;
#11612=CARTESIAN_POINT ( 'NONE',  ( 1.593127413382953383, 20.37819992234354771, -2.091722143975172532 ) ) ;
#11619=CARTESIAN_POINT ( 'NONE',  ( -3.518350579753630747, 38.12180007765648071, -1.080741659609802729 ) ) ;
#11632=CARTESIAN_POINT ( 'NONE',  ( 2.500000000000001332, 24.24680007765647716, -0.05647727720535888202 ) ) ;
#11634=CARTESIAN_POINT ( 'NONE',  ( -2.864755990943265829, 20.74680007765647716, -2.011557305968488141 ) ) ;
#11638=CARTESIAN_POINT ( 'NONE',  ( 2.211161402132839626, 15.37819992234354771, -2.942372952327218183 ) ) ;
#11641=CARTESIAN_POINT ( 'NONE',  ( -4.518350579753632523, 38.12180007765647360, -1.405661355842698468 ) ) ;
#11647=AXIS2_PLACEMENT_3D ( 'NONE', #14616, #424, #17409 ) ;
#11654=ORIENTED_EDGE ( 'NONE', *, *, #818, .F. ) ;
#11662=CARTESIAN_POINT ( 'NONE',  ( 0.05938372350919016857, 27.62819992234354416, -4.731580009072201776 ) ) ;
#11663=CARTESIAN_POINT ( 'NONE',  ( 3.518350579753606322, 28.12819992234354416, -1.080741659609876892 ) ) ;
#11664=CARTESIAN_POINT ( 'NONE',  ( 0.7188294034286553114, 16.25319992234354771, 2.395093729190349130 ) ) ;
#11666=CARTESIAN_POINT ( 'NONE',  ( -1.444289557195956863, 34.00319992234354771, 4.262301884875733471 ) ) ;
#11670=CARTESIAN_POINT ( 'NONE',  ( -1.027846397803541700, 32.49680007765648071, 3.346150245485522312 ) ) ;
#11673=CARTESIAN_POINT ( 'NONE',  ( 3.607379964056306676, 31.49680007765647716, -2.690724712371305838 ) ) ;
#11676=CARTESIAN_POINT ( 'NONE',  ( 1.135272562821090458, 32.24680007765648071, 3.311245368580554072 ) ) ;
#11682=CARTESIAN_POINT ( 'NONE',  ( -2.864755990943222308, 29.25319992234354416, 2.011557305968548093 ) ) ;
#11686=CARTESIAN_POINT ( 'NONE',  ( -1.135272562821090014, 38.49680007765647360, -3.311245368580554072 ) ) ;
#11688=CARTESIAN_POINT ( 'NONE',  ( 2.211161402132839626, 37.87819992234352640, -2.942372952327218183 ) ) ;
#11702=CARTESIAN_POINT ( 'NONE',  ( -1.593127413382952939, 16.62819992234354061, 2.091722143975172532 ) ) ;
#11711=CARTESIAN_POINT ( 'NONE',  ( -3.500000000000000444, 37.99680007765647360, 0.05647727720536892260 ) ) ;
#11721=CARTESIAN_POINT ( 'NONE',  ( -3.500000000000000444, 14.50319992234354416, -0.05647727720529563400 ) ) ;
#11723=CARTESIAN_POINT ( 'NONE',  ( 1.989345975306426206, 26.49680007765648426, -1.515154207786343799 ) ) ;
#11725=CARTESIAN_POINT ( 'NONE',  ( 2.864755990943265829, 19.49680007765648071, 2.011557305968487697 ) ) ;
#11729=CARTESIAN_POINT ( 'NONE',  ( 1.135272562821020070, 22.75319992234354416, -3.311245368580577164 ) ) ;
#11732=CARTESIAN_POINT ( 'NONE',  ( 1.336863392178479160, 38.74680007765646650, -4.297206761780677731 ) ) ;
#11753=CARTESIAN_POINT ( 'NONE',  ( -2.733110507866328476, 24.87819992234354771, -3.862833514489096398 ) ) ;
#11754=CARTESIAN_POINT ( 'NONE',  ( 2.115076519116425580, 38.62819992234354061, 3.012182706137062294 ) ) ;
#11756=CARTESIAN_POINT ( 'NONE',  ( -0.8262555684460826111, 19.00319992234354771, 2.360188852285421302 ) ) ;
#11758=CARTESIAN_POINT ( 'NONE',  ( 2.733110507866247652, 18.87180007765647716, -3.862833514489153686 ) ) ;
#11763=CARTESIAN_POINT ( 'NONE',  ( 2.864755990943265829, 26.99680007765648071, 2.011557305968487697 ) ) ;
#11766=CARTESIAN_POINT ( 'NONE',  ( -3.607379964056306676, 30.24680007765647360, 2.690724712371306282 ) ) ;
#11769=CARTESIAN_POINT ( 'NONE',  ( 2.864755990943265829, 31.99680007765647716, 2.011557305968487697 ) ) ;
#11776=CARTESIAN_POINT ( 'NONE',  ( 2.864755990943222308, 30.50319992234354416, -2.011557305968548093 ) ) ;
#11780=CARTESIAN_POINT ( 'NONE',  ( 2.481649420246374138, 24.12180007765648071, -0.8687765177876252132 ) ) ;
#11781=CARTESIAN_POINT ( 'NONE',  ( -0.05938372350918959958, 18.87819992234354416, 4.731580009072201776 ) ) ;
#11798=CARTESIAN_POINT ( 'NONE',  ( -2.481649420246391902, 27.12819992234355126, -0.8687765177875723666 ) ) ;
#11800=CARTESIAN_POINT ( 'NONE',  ( 3.500000000000000444, 19.24680007765648071, -0.05647727720536935281 ) ) ;
#11805=CARTESIAN_POINT ( 'NONE',  ( -2.115076519116362519, 37.62180007765648071, 3.012182706137107147 ) ) ;
#11819=CARTESIAN_POINT ( 'NONE',  ( 2.055738996568313048, 34.49680007765648071, 1.423772053676023441 ) ) ;
#11821=CARTESIAN_POINT ( 'NONE',  ( -2.211161402132901799, 18.37180007765647716, -2.942372952327172886 ) ) ;
#11827=CARTESIAN_POINT ( 'NONE',  ( -2.211161402132839182, 16.62819992234354416, 2.942372952327218627 ) ) ;
#11831=CARTESIAN_POINT ( 'NONE',  ( 4.518350579753633411, 39.37180007765647360, 1.405661355842698468 ) ) ;
#11849=CARTESIAN_POINT ( 'NONE',  ( -4.499999999999999112, 24.50319992234354771, -0.05647727720528529505 ) ) ;
#11850=CARTESIAN_POINT ( 'NONE',  ( 0.05938372350920110426, 32.62819992234354771, -3.680117784833935701 ) ) ;
#11851=CARTESIAN_POINT ( 'NONE',  ( -0.7188294034286550893, 17.50319992234354771, -2.395093729190349130 ) ) ;
#11853=CARTESIAN_POINT ( 'NONE',  ( 0.05938372350929014415, 19.87180007765647716, 4.731580009072201776 ) ) ;
#11858=CARTESIAN_POINT ( 'NONE',  ( 3.518350579753631191, 26.87180007765647360, 1.080741659609802285 ) ) ;
#11872=CARTESIAN_POINT ( 'NONE',  ( -3.500000000000000444, 27.00319992234354771, -0.05647727720529563400 ) ) ;
#11875=CARTESIAN_POINT ( 'NONE',  ( 2.500000000000001332, 19.24680007765648071, -0.05647727720535888202 ) ) ;
#11877=CARTESIAN_POINT ( 'NONE',  ( 2.829195390882724759, 17.87819992234354416, -3.793023760679264278 ) ) ;
#11892=CARTESIAN_POINT ( 'NONE',  ( -0.05938372350921170689, 31.37819992234354061, 2.628655560595669183 ) ) ;
#11895=CARTESIAN_POINT ( 'NONE',  ( -1.027846397803541700, 24.99680007765647716, 3.346150245485522312 ) ) ;
#11913=CARTESIAN_POINT ( 'NONE',  ( 2.518350579753628971, 31.87180007765648426, 0.7558219633769073242 ) ) ;
#11915=CARTESIAN_POINT ( 'NONE',  ( -2.798362969681365886, 32.74680007765648071, 2.102939460078824929 ) ) ;
#11921=CARTESIAN_POINT ( 'NONE',  ( -0.05938372350920063936, 18.87819992234354771, 3.680117784833935701 ) ) ;
#11925=CARTESIAN_POINT ( 'NONE',  ( -1.444289557196047014, 38.49680007765647360, -4.262301884875704161 ) ) ;
#11947=CARTESIAN_POINT ( 'NONE',  ( 4.481649420246397675, 23.37819992234354416, 1.518615910253363177 ) ) ;
#11948=CARTESIAN_POINT ( 'NONE',  ( 2.211161402132839182, 35.37819992234354061, -2.942372952327217739 ) ) ;
#11949=CARTESIAN_POINT ( 'NONE',  ( -1.989345975306457071, 22.25319992234354771, -1.515154207786300944 ) ) ;
#11952=CARTESIAN_POINT ( 'NONE',  ( 1.444289557196047680, 19.74680007765647716, 4.262301884875704161 ) ) ;
#11956=CARTESIAN_POINT ( 'NONE',  ( 0.05938372350927906274, 39.87180007765648071, 3.680117784833935701 ) ) ;
#11968=CARTESIAN_POINT ( 'NONE',  ( 1.135272562821020070, 30.25319992234354416, -3.311245368580577164 ) ) ;
#11969=CARTESIAN_POINT ( 'NONE',  ( 3.500000000000000444, 15.75319992234354416, 0.05647727720529520379 ) ) ;
#11971=CARTESIAN_POINT ( 'NONE',  ( -1.497042530366477164, 25.12180007765648071, 2.161531897785062384 ) ) ;
#11972=CARTESIAN_POINT ( 'NONE',  ( -2.733110507866328476, 14.87819992234354238, -3.862833514489096398 ) ) ;
#11976=CARTESIAN_POINT ( 'NONE',  ( 2.829195390882805583, 37.12180007765647360, 3.793023760679204770 ) ) ;
#11985=CARTESIAN_POINT ( 'NONE',  ( 2.518350579753611207, 28.12819992234355126, -0.7558219633769606149 ) ) ;
#11987=CARTESIAN_POINT ( 'NONE',  ( 3.518350579753631191, 21.87180007765647360, 1.080741659609802285 ) ) ;
#12001=CARTESIAN_POINT ( 'NONE',  ( 2.055738996568313048, 26.99680007765647716, 1.423772053676023441 ) ) ;
#12003=CARTESIAN_POINT ( 'NONE',  ( 3.481649420246370141, 29.12180007765647360, -1.193696214020541602 ) ) ;
#12009=CARTESIAN_POINT ( 'NONE',  ( -2.115076519116362519, 17.62180007765647716, 3.012182706137107147 ) ) ;
#12030=CARTESIAN_POINT ( 'NONE',  ( -3.607379964056363075, 22.25319992234354416, -2.690724712371229899 ) ) ;
#12031=CARTESIAN_POINT ( 'NONE',  ( -3.481649420246394566, 34.62819992234354771, -1.193696214020467883 ) ) ;
#12033=CARTESIAN_POINT ( 'NONE',  ( -2.481649420246391902, 22.12819992234354771, -0.8687765177875723666 ) ) ;
#12035=CARTESIAN_POINT ( 'NONE',  ( 2.733110507866247652, 16.37180007765647716, -3.862833514489153686 ) ) ;
#12039=CARTESIAN_POINT ( 'NONE',  ( 2.115076519116362963, 36.37180007765648782, -3.012182706137107147 ) ) ;
#12047=CARTESIAN_POINT ( 'NONE',  ( -3.500000000000000444, 15.49680007765647893, 0.05647727720536901974 ) ) ;
#12053=CARTESIAN_POINT ( 'NONE',  ( 3.518350579753605434, 30.62819992234353705, -1.080741659609877114 ) ) ;
#12056=CARTESIAN_POINT ( 'NONE',  ( -0.7188294034286043521, 19.99680007765648071, 2.395093729190366005 ) ) ;
#12057=CARTESIAN_POINT ( 'NONE',  ( -4.499999999999999112, 17.00319992234354416, -0.05647727720528529505 ) ) ;
#12061=CARTESIAN_POINT ( 'NONE',  ( 2.798362969681366330, 16.49680007765647716, -2.102939460078824929 ) ) ;
#12073=CARTESIAN_POINT ( 'NONE',  ( 1.989345975306457071, 28.50319992234355126, 1.515154207786300500 ) ) ;
#12076=CARTESIAN_POINT ( 'NONE',  ( 2.798362969681366330, 23.99680007765647716, -2.102939460078824929 ) ) ;
#12093=CARTESIAN_POINT ( 'NONE',  ( 0.8262555684461332373, 32.24680007765648071, 2.360188852285403982 ) ) ;
#12096=CARTESIAN_POINT ( 'NONE',  ( -2.798362969681365886, 30.24680007765648071, 2.102939460078824929 ) ) ;
#12102=CARTESIAN_POINT ( 'NONE',  ( 2.864755990943265829, 21.99680007765647716, 2.011557305968487697 ) ) ;
#12116=AXIS2_PLACEMENT_3D ( 'NONE', #3485, #16289, #9132 ) ;
#12117=CARTESIAN_POINT ( 'NONE',  ( 2.798362969681366330, 31.49680007765647716, -2.102939460078824929 ) ) ;
#12122=CARTESIAN_POINT ( 'NONE',  ( 1.336863392178569754, 31.25319992234354416, 4.297206761780648421 ) ) ;
#12123=CARTESIAN_POINT ( 'NONE',  ( -1.027846397803611866, 35.00319992234354771, -3.346150245485499219 ) ) ;
#12124=CARTESIAN_POINT ( 'NONE',  ( 1.989345975306457071, 26.00319992234354771, 1.515154207786300500 ) ) ;
#12126=CARTESIAN_POINT ( 'NONE',  ( -4.518350579753602325, 39.37819992234354771, 1.405661355842794391 ) ) ;
#12130=CARTESIAN_POINT ( 'NONE',  ( 3.481649420246369697, 36.62180007765648071, -1.193696214020541824 ) ) ;
#12142=CARTESIAN_POINT ( 'NONE',  ( 2.211161402132839626, 32.87819992234354771, -2.942372952327218183 ) ) ;
#12145=CARTESIAN_POINT ( 'NONE',  ( -2.518350579753628526, 23.12180007765647005, -0.7558219633769075463 ) ) ;
#12146=EDGE_CURVE ( 'NONE', #9517, #13037, #6171, .T. ) ;
#12148=CARTESIAN_POINT ( 'NONE',  ( 4.499999999999999112, 18.25319992234354771, 0.05647727720528474687 ) ) ;
#12154=CARTESIAN_POINT ( 'NONE',  ( -1.336863392178478716, 39.99680007765647360, 4.297206761780677731 ) ) ;
#12162=CARTESIAN_POINT ( 'NONE',  ( -0.05938372350927861171, 18.62180007765647005, -3.680117784833935701 ) ) ;
#12167=CARTESIAN_POINT ( 'NONE',  ( -0.05938372350921170689, 28.87819992234354416, 2.628655560595669183 ) ) ;
#12170=CARTESIAN_POINT ( 'NONE',  ( -2.115076519116362519, 20.12180007765648071, 3.012182706137107147 ) ) ;
#12178=CARTESIAN_POINT ( 'NONE',  ( -2.733110507866247652, 25.12180007765648071, 3.862833514489154574 ) ) ;
#12185=STYLED_ITEM ( 'NONE', ( #4436 ), #9153 ) ;
#12187=CARTESIAN_POINT ( 'NONE',  ( 1.593127413382998903, 29.62180007765647716, 2.091722143975139669 ) ) ;
#12189=CARTESIAN_POINT ( 'NONE',  ( 2.798362969681366330, 28.99680007765647716, -2.102939460078824929 ) ) ;
#12195=CARTESIAN_POINT ( 'NONE',  ( -0.05938372350927861171, 26.12180007765647005, -3.680117784833935701 ) ) ;
#12209=CARTESIAN_POINT ( 'NONE',  ( -2.798362969681365886, 27.74680007765648071, 2.102939460078824929 ) ) ;
#12213=CARTESIAN_POINT ( 'NONE',  ( 1.444289557195957086, 35.25319992234354771, -4.262301884875733471 ) ) ;
#12215=CARTESIAN_POINT ( 'NONE',  ( 0.05938372350921204690, 30.12819992234354416, -2.628655560595669183 ) ) ;
#12217=CARTESIAN_POINT ( 'NONE',  ( 3.607379964056306676, 28.99680007765648071, -2.690724712371305838 ) ) ;
#12231=CARTESIAN_POINT ( 'NONE',  ( 1.027846397803542144, 16.24680007765647716, -3.346150245485522312 ) ) ;
#12236=CARTESIAN_POINT ( 'NONE',  ( 2.211161402132839626, 37.87819992234352640, -2.942372952327218183 ) ) ;
#12238=CARTESIAN_POINT ( 'NONE',  ( 1.497042530366477164, 31.37180007765648426, -2.161531897785062384 ) ) ;
#12239=CARTESIAN_POINT ( 'NONE',  ( 1.444289557195957086, 27.75319992234354416, -4.262301884875733471 ) ) ;
#12243=CARTESIAN_POINT ( 'NONE',  ( 0.05938372350929014415, 39.87180007765647360, 4.731580009072201776 ) ) ;
#12254=CARTESIAN_POINT ( 'NONE',  ( 3.481649420246369697, 19.12180007765648071, -1.193696214020541824 ) ) ;
#12258=CARTESIAN_POINT ( 'NONE',  ( -0.7188294034286550893, 35.00319992234354771, -2.395093729190349130 ) ) ;
#12260=CARTESIAN_POINT ( 'NONE',  ( -2.864755990943265829, 30.74680007765647716, -2.011557305968488141 ) ) ;
#12263=CARTESIAN_POINT ( 'NONE',  ( 2.864755990943222308, 15.50319992234354416, -2.011557305968548093 ) ) ;
#12268=CARTESIAN_POINT ( 'NONE',  ( 2.829195390882805583, 27.12180007765647716, 3.793023760679204770 ) ) ;
#12276=CARTESIAN_POINT ( 'NONE',  ( -2.481649420246374138, 35.37180007765647360, 0.8687765177876256573 ) ) ;
#12278=CARTESIAN_POINT ( 'NONE',  ( -1.027846397803541700, 32.49680007765648071, 3.346150245485522312 ) ) ;
#12281=CARTESIAN_POINT ( 'NONE',  ( -3.636013921692167639, 15.00000000000000178, -1.612974510979999332 ) ) ;
#12285=CARTESIAN_POINT ( 'NONE',  ( -3.481649420246369697, 22.87180007765647360, 1.193696214020542490 ) ) ;
#12297=CARTESIAN_POINT ( 'NONE',  ( -1.593127413382998459, 18.37180007765648071, -2.091722143975139669 ) ) ;
#12301=CARTESIAN_POINT ( 'NONE',  ( -4.499999999999999112, 37.00319992234354771, -0.05647727720528529505 ) ) ;
#12303=CARTESIAN_POINT ( 'NONE',  ( -0.7188294034286550893, 27.50319992234354771, -2.395093729190349130 ) ) ;
#12307=CARTESIAN_POINT ( 'NONE',  ( 2.733110507866247652, 23.87180007765647716, -3.862833514489153686 ) ) ;
#12310=VERTEX_POINT ( 'NONE', #10025 ) ;
#12320=ORIENTED_EDGE ( 'NONE', *, *, #818, .T. ) ;
#12327=CARTESIAN_POINT ( 'NONE',  ( -3.500000000000000444, 34.50319992234354771, -0.05647727720529563400 ) ) ;
#12328=CARTESIAN_POINT ( 'NONE',  ( 3.481649420246395010, 23.37819992234354061, 1.193696214020467439 ) ) ;
#12330=CARTESIAN_POINT ( 'NONE',  ( 1.593127413382998903, 27.12180007765647716, 2.091722143975139669 ) ) ;
#12331=CARTESIAN_POINT ( 'NONE',  ( -4.481649420246396787, 24.62819992234354416, -1.518615910253363399 ) ) ;
#12336=CARTESIAN_POINT ( 'NONE',  ( -4.481649420246366589, 37.87180007765647360, 1.518615910253458878 ) ) ;
#12348=CARTESIAN_POINT ( 'NONE',  ( -1.497042530366522461, 34.87819992234354771, -2.161531897785030409 ) ) ;
#12351=CARTESIAN_POINT ( 'NONE',  ( 1.135272562821090458, 27.24680007765648071, 3.311245368580554072 ) ) ;
#12352=CARTESIAN_POINT ( 'NONE',  ( -3.500000000000000444, 29.50319992234354416, -0.05647727720529563400 ) ) ;
#12359=CARTESIAN_POINT ( 'NONE',  ( -3.673772985318219053, 20.74680007765647716, -2.599342558260952174 ) ) ;
#12365=CARTESIAN_POINT ( 'NONE',  ( 0.8262555684461332373, 34.74680007765647360, 2.360188852285403982 ) ) ;
#12367=CARTESIAN_POINT ( 'NONE',  ( 2.864755990943265829, 39.49680007765647360, 2.011557305968487697 ) ) ;
#12377=CARTESIAN_POINT ( 'NONE',  ( -3.500000000000000444, 25.49680007765647716, 0.05647727720536892260 ) ) ;
#12384=STYLED_ITEM('',(#18410),#14305);
#12392=CARTESIAN_POINT ( 'NONE',  ( 2.798362969681366330, 36.49680007765648071, -2.102939460078824929 ) ) ;
#12396=CARTESIAN_POINT ( 'NONE',  ( 3.607379964056363075, 33.50319992234354061, 2.690724712371229010 ) ) ;
#12398=CARTESIAN_POINT ( 'NONE',  ( -2.055738996568281518, 29.25319992234355126, 1.423772053676066962 ) ) ;
#12402=CARTESIAN_POINT ( 'NONE',  ( -1.444289557196047014, 25.99680007765648071, -4.262301884875704161 ) ) ;
#12404=ORIENTED_EDGE ( 'NONE', *, *, #379, .T. ) ;
#12416=CARTESIAN_POINT ( 'NONE',  ( -2.798362969681365886, 17.74680007765647716, 2.102939460078824929 ) ) ;
#12419=CARTESIAN_POINT ( 'NONE',  ( 3.518350579753605434, 35.62819992234353350, -1.080741659609877114 ) ) ;
#12420=CARTESIAN_POINT ( 'NONE',  ( -1.135272562821019626, 16.50319992234354416, 3.311245368580577164 ) ) ;
#12422=CARTESIAN_POINT ( 'NONE',  ( 0.05938372350926800214, 27.37180007765647716, 2.628655560595669183 ) ) ;
#12423=CARTESIAN_POINT ( 'NONE',  ( -4.518350579753602325, 21.87819992234354416, 1.405661355842794391 ) ) ;
#12429=CARTESIAN_POINT ( 'NONE',  ( 3.500000000000000444, 19.24680007765648071, -0.05647727720536935281 ) ) ;
#12438=CARTESIAN_POINT ( 'NONE',  ( -2.864755990943265829, 18.24680007765648071, -2.011557305968488141 ) ) ;
#12444=CARTESIAN_POINT ( 'NONE',  ( 2.518350579753611207, 38.12819992234354771, -0.7558219633769606149 ) ) ;
#12446=CARTESIAN_POINT ( 'NONE',  ( 2.798362969681366330, 33.99680007765648071, -2.102939460078824929 ) ) ;
#12447=CARTESIAN_POINT ( 'NONE',  ( -2.798362969681409851, 24.75319992234354416, -2.102939460078765421 ) ) ;
#12456=CARTESIAN_POINT ( 'NONE',  ( -1.497042530366477164, 35.12180007765647360, 2.161531897785062384 ) ) ;
#12459=CARTESIAN_POINT ( 'NONE',  ( 2.211161402132902243, 37.12180007765647360, 2.942372952327172442 ) ) ;
#12466=CARTESIAN_POINT ( 'NONE',  ( 1.135272562821090458, 27.24680007765648071, 3.311245368580554072 ) ) ;
#12475=CARTESIAN_POINT ( 'NONE',  ( 2.115076519116362963, 38.87180007765645939, -3.012182706137107147 ) ) ;
#12481=CARTESIAN_POINT ( 'NONE',  ( 0.05938372350919016857, 35.12819992234354771, -4.731580009072201776 ) ) ;
#12485=CARTESIAN_POINT ( 'NONE',  ( 1.593127413382953383, 25.37819992234354416, -2.091722143975172532 ) ) ;
#12489=CARTESIAN_POINT ( 'NONE',  ( -1.336863392178478716, 24.99680007765647716, 4.297206761780677731 ) ) ;
#12509=CARTESIAN_POINT ( 'NONE',  ( 1.027846397803612311, 36.25319992234354771, 3.346150245485499219 ) ) ;
#12510=CARTESIAN_POINT ( 'NONE',  ( 2.798362969681409851, 18.50319992234354771, 2.102939460078764977 ) ) ;
#12512=CARTESIAN_POINT ( 'NONE',  ( -0.05938372350926768989, 26.12180007765648426, -2.628655560595669183 ) ) ;
#12514=CARTESIAN_POINT ( 'NONE',  ( -4.518350579753602325, 29.37819992234355126, 1.405661355842794391 ) ) ;
#12520=CARTESIAN_POINT ( 'NONE',  ( -2.115076519116362519, 20.12180007765648071, 3.012182706137107147 ) ) ;
#12530=CARTESIAN_POINT ( 'NONE',  ( -3.500000000000000444, 15.49680007765647893, 0.05647727720536892260 ) ) ;
#12535=CARTESIAN_POINT ( 'NONE',  ( 2.481649420246391902, 38.37819992234354061, 0.8687765177875720335 ) ) ;
#12537=CARTESIAN_POINT ( 'NONE',  ( -2.115076519116362519, 35.12180007765645939, 3.012182706137107147 ) ) ;
#12538=CARTESIAN_POINT ( 'NONE',  ( 0.05938372350920109732, 30.12819992234354416, -3.680117784833935701 ) ) ;
#12552=CARTESIAN_POINT ( 'NONE',  ( 2.518350579753611207, 15.62819992234354594, -0.7558219633769606149 ) ) ;
#12562=CARTESIAN_POINT ( 'NONE',  ( -3.500000000000000444, 35.49680007765648071, 0.05647727720536892260 ) ) ;
#12571=CARTESIAN_POINT ( 'NONE',  ( -3.500000000000000444, 37.99680007765647360, 0.05647727720536892260 ) ) ;
#12575=CARTESIAN_POINT ( 'NONE',  ( -1.444289557196047014, 15.99680007765647716, -4.262301884875704161 ) ) ;
#12577=CARTESIAN_POINT ( 'NONE',  ( 1.497042530366522461, 38.62819992234354771, 2.161531897785029965 ) ) ;
#12580=CARTESIAN_POINT ( 'NONE',  ( 0.05938372350929014415, 24.87180007765647716, 4.731580009072201776 ) ) ;
#12595=CARTESIAN_POINT ( 'NONE',  ( -2.829195390882724315, 16.62819992234354061, 3.793023760679264722 ) ) ;
#12596=CARTESIAN_POINT ( 'NONE',  ( 3.500000000000000444, 23.25319992234354416, 0.05647727720529520379 ) ) ;
#12598=CARTESIAN_POINT ( 'NONE',  ( 2.055738996568313048, 31.99680007765648426, 1.423772053676023441 ) ) ;
#12599=CARTESIAN_POINT ( 'NONE',  ( -3.673772985318163098, 21.75319992234354416, 2.599342558261029001 ) ) ;
#12606=CARTESIAN_POINT ( 'NONE',  ( -0.05938372350927861171, 18.62180007765647005, -3.680117784833935701 ) ) ;
#12617=CARTESIAN_POINT ( 'NONE',  ( -1.027846397803541700, 24.99680007765647716, 3.346150245485522312 ) ) ;
#12623=CARTESIAN_POINT ( 'NONE',  ( -2.798362969681409851, 17.25319992234354416, -2.102939460078765421 ) ) ;
#12625=CARTESIAN_POINT ( 'NONE',  ( -2.798362969681365886, 27.74680007765648071, 2.102939460078824929 ) ) ;
#12626=CARTESIAN_POINT ( 'NONE',  ( 2.798362969681409851, 23.50319992234354416, 2.102939460078764977 ) ) ;
#12638=CARTESIAN_POINT ( 'NONE',  ( -3.000000000000003553, 15.00000000000000711, -0.1687737011545533683 ) ) ;
#12641=CARTESIAN_POINT ( 'NONE',  ( -2.055738996568313048, 35.74680007765648071, -1.423772053676023441 ) ) ;
#12643=CARTESIAN_POINT ( 'NONE',  ( 1.027846397803542144, 38.74680007765647360, -3.346150245485522312 ) ) ;
#12647=CARTESIAN_POINT ( 'NONE',  ( 0.05938372350927906274, 34.87180007765645939, 3.680117784833935701 ) ) ;
#12660=CARTESIAN_POINT ( 'NONE',  ( -2.518350579753628526, 15.62180007765648071, -0.7558219633769075463 ) ) ;
#12665=CARTESIAN_POINT ( 'NONE',  ( 4.481649420246397675, 38.37819992234354061, 1.518615910253363177 ) ) ;
#12667=CARTESIAN_POINT ( 'NONE',  ( -0.7188294034286550893, 32.50319992234354771, -2.395093729190349130 ) ) ;
#12670=CARTESIAN_POINT ( 'NONE',  ( 0.05938372350929014415, 37.37180007765647360, 4.731580009072201776 ) ) ;
#12688=CARTESIAN_POINT ( 'NONE',  ( -4.499999999999999112, 22.00319992234354061, -0.05647727720528529505 ) ) ;
#12689=CARTESIAN_POINT ( 'NONE',  ( -1.027846397803611866, 22.50319992234354416, -3.346150245485499219 ) ) ;
#12692=CARTESIAN_POINT ( 'NONE',  ( -1.989345975306426206, 37.74680007765647360, 1.515154207786343799 ) ) ;
#12693=CARTESIAN_POINT ( 'NONE',  ( -1.336863392178569088, 30.00319992234354416, -4.297206761780648421 ) ) ;
#12698=CARTESIAN_POINT ( 'NONE',  ( 3.500000000000000444, 24.24680007765647716, -0.05647727720536935281 ) ) ;
#12703=CARTESIAN_POINT ( 'NONE',  ( 3.673772985318219053, 19.49680007765647005, 2.599342558260951730 ) ) ;
#12709=CARTESIAN_POINT ( 'NONE',  ( 1.027846397803542144, 23.74680007765647716, -3.346150245485522312 ) ) ;
#12715=CARTESIAN_POINT ( 'NONE',  ( -2.798362969681409851, 19.75319992234354416, -2.102939460078765421 ) ) ;
#12719=CARTESIAN_POINT ( 'NONE',  ( -0.05938372350926768989, 16.12180007765648071, -2.628655560595669183 ) ) ;
#12722=CARTESIAN_POINT ( 'NONE',  ( -2.798362969681409851, 27.25319992234354771, -2.102939460078765421 ) ) ;
#12725=( BOUNDED_SURFACE ( )  B_SPLINE_SURFACE ( 3, 2, ( 
 ( #10218, #12825, #11423, #7445, #14320, #13103, #5780, #7347, #13008, #417, #3194, #7251, #6055, #8833, #3007, #4299, #10314, #15997, #11520, #14607, #1909, #12740, #11335, #15617, #2918, #8552, #14227, #1530, #17113, #4389, #11800, #6245, #13383, #16274, #698, #17775, #16455, #12170, #509, #13192, #6344, #16093, #6151, #9026, #2094, #17497, #3474, #14978, #6431, #9118, #6521, #11987, #3385, #3736, #17681, #13473, #17861, #5125, #2275, #10782, #9387, #14797, #3567, #10414, #4762, #9213, #4945, #14703, #12076, #7904, #14891, #2001, #7627, #13292, #7722, #605, #11895, #15064, #10600, #2188, #3652, #7816, #784, #17594, #4857, #5037, #10508, #7539, #10693, #16366, #16177, #9299, #13559, #876, #12351, #2459, #13937, #9574, #12625, #15434, #6967, #8180, #17947, #2368, #18315, #18226, #18042, #1335, #1150, #5495, #6791, #16738, #6617, #13652, #2549, #16552, #6696, #9479, #9753, #1245, #2731, #15253, #12260, #11141, #15154, #7998, #8089, #972, #5219, #14024, #10872, #11232, #5315, #4102, #3828, #18138, #13751, #9659, #1061, #8278, #8364, #10967, #4196, #5406, #16649, #9843, #13840, #3922, #12446, #11057, #4015, #5586, #15338, #2637, #6879, #16831, #16920, #12537, #23, #8444, #13080, #17192, #15692, #17288, #4465, #7235, #3082, #12893, #14492, #398, #6034, #8622, #17378, #113, #5766, #17013, #11403, #2816, #7423, #200, #2990, #7054, #5943, #1600, #11686, #11592, #2901, #17095, #5851, #15599, #14299, #14388, #8535, #11497, #4643, #4284, #10102, #15519, #4558, #14114, #4367 ),
 ( #10017, #1427, #10198, #1791, #15785, #12719, #5674, #11319, #12987, #7145, #9928, #8715, #301, #1692, #7327, #14206, #1511, #15877, #12807, #3174, #8812, #855, #16069, #6501, #3364, #9281, #4743, #486, #13268, #675, #11875, #3545, #10391, #9009, #17753, #17567, #12056, #6128, #1889, #7702, #14584, #2256, #2165, #16252, #17474, #9189, #16161, #4839, #1980, #14684, #14871, #10487, #7881, #5014, #14961, #3453, #7520, #10296, #13538, #7797, #7607, #12145, #9094, #13454, #14776, #6322, #13172, #3270, #2073, #11780, #585, #10670, #17838, #6226, #15976, #13363, #8907, #11971, #17663, #4925, #10576, #766, #6411, #16340, #3632, #12512, #6677, #6858, #10849, #18113, #2526, #18207, #8255, #12330, #16805, #12422, #2436, #9366, #13913, #9729, #3901, #13998, #8339, #5471, #1313, #2348, #9548, #10763, #11032, #16438, #11116, #15412, #15042, #3804, #10943, #13819, #16626, #15315, #6945, #2707, #3716, #7979, #15226, #13632, #944, #6588, #18016, #12238, #1036, #4075, #3988, #5290, #12598, #8156, #17926, #5102, #1129, #16715, #5198, #16525, #9459, #15132, #8062, #6765, #5383, #13725, #9637, #2615, #1221, #16897, #17165, #277, #8598, #4173, #9816, #14088, #12782, #1399, #5559, #3151, #17071, #2964, #14366, #90, #1577, #5743, #14273, #11383, #10079, #8784, #4533, #11208, #15497, #4344, #8425, #2794, #7027, #9991, #12692, #14180, #7301, #4439, #1487, #17260, #15666, #18369, #14465, #7214, #5826, #10175, #15853, #12961, #1769, #7399, #7121, #12868, #5651, #11293, #176, #11471, #16985 ),
 ( #1666, #4262, #8507, #15758, #9905, #3058, #8690, #15577, #5920, #18286, #2877, #11565, #13059, #14848, #11664, #3339, #16047, #6296, #8985, #9167, #4816, #3431, #13242, #13431, #11851, #14658, #14940, #745, #17643, #1958, #17449, #6104, #9255, #17547, #2232, #2140, #11756, #7493, #3606, #370, #7771, #561, #16226, #10464, #16142, #6203, #16319, #6389, #3246, #4991, #9072, #6009, #13342, #4900, #10648, #1862, #14751, #13151, #2048, #10551, #462, #12033, #11949, #17725, #7584, #4621, #3519, #4718, #17356, #10368, #10269, #15949, #8884, #14562, #7680, #652, #9617, #7858, #5266, #13516, #15204, #9342, #13793, #15291, #13608, #9700, #16779, #12485, #831, #6472, #1015, #16412, #12124, #15021, #2411, #17818, #3782, #2591, #6743, #9433, #6835, #6656, #3696, #4049, #12303, #1103, #18178, #5447, #8224, #11094, #15385, #15108, #3876, #10739, #5079, #16600, #17995, #2320, #12398, #13888, #9523, #7951, #922, #6564, #8042, #12215, #17902, #5172, #10921, #2504, #3965, #13703, #8132, #10826, #16503, #18090, #5360, #11007, #16687, #1199, #9796, #14250, #8484, #9884, #12667, #2774, #1552, #15556, #12937, #15734, #7279, #14156, #18265, #2684, #249, #154, #18356, #1641, #1467, #5805, #7098, #17050, #6921, #13977, #2851, #16870, #7004, #4415, #11544, #8404, #17235, #14061, #5894, #15477, #11182, #5630, #11360, #4240, #7191, #1374, #11273, #10058, #12761, #3035, #16962, #15643, #65, #8666, #11448, #5720, #14343, #9967, #4321, #12577, #17138, #4509, #2943, #10151, #8316, #1290, #5535 ),
 ( #4149, #8578, #12848, #3312, #6178, #8955, #7649, #11638, #12263, #1936, #3407, #14819, #7999, #4877, #13653, #17948, #17425, #11827, #348, #14437, #17523, #14633, #1739, #14725, #16201, #4786, #7372, #13033, #17332, #10341, #4595, #3126, #974, #7559, #532, #11921, #16021, #10439, #10245, #5986, #13215, #15924, #6618, #13315, #9049, #3222, #2024, #16115, #4691, #7470, #8858, #629, #6267, #5220, #10528, #2118, #17617, #14537, #15830, #8761, #3494, #13128, #1833, #9139, #437, #6076, #11729, #15155, #3831, #11058, #6697, #15255, #12626, #1428, #16650, #7055, #3924, #9845, #5317, #1062, #13841, #1246, #12447, #4103, #10969, #9575, #18316, #18140, #5588, #2551, #5496, #8280, #11234, #14026, #5408, #4197, #18228, #8181, #2462, #1336, #15520, #9661, #12722, #14115, #16922, #24, #8090, #15339, #16553, #16833, #9480, #2818, #8445, #13753, #1152, #16740, #6881, #4016, #2732, #10873, #12352, #18043, #6794, #2638, #13938, #12538, #11142, #9755, #15435, #8365, #6968, #4560, #7237, #4644, #4466, #202, #9930, #1601, #13082, #10199, #12894, #10297, #10105, #1513, #1890, #15788, #11594, #15977, #3273, #399, #8910, #7522, #5853, #1694, #8536, #4285, #14389, #3083, #15601, #15878, #6037, #7329, #2902, #14209, #7146, #11498, #12808, #11320, #14587, #8716, #12989, #1792, #17194, #303, #114, #5767, #5945, #11405, #13175, #3175, #17291, #17097, #8813, #14494, #7425, #15694, #4368, #11688, #17379, #5675, #17014, #10018, #2992, #8624, #14301, #5104, #16341, #10489, #17840, #17664, #3634 ),
 ( #9282, #10578, #16254, #11972, #3717, #7882, #9010, #10764, #4926, #15044, #767, #5016, #16439, #7608, #3546, #13269, #9191, #14962, #586, #13540, #12057, #856, #7704, #10394, #2257, #6228, #6129, #11877, #487, #16071, #12148, #4745, #9367, #3455, #6502, #11781, #14872, #17475, #7798, #1982, #6412, #2349, #17570, #7980, #2167, #14686, #3366, #6324, #4840, #13455, #17755, #10672, #16162, #9096, #14777, #2074, #13364, #677, #12599, #12423, #11118, #18115, #9639, #17927, #6591, #13820, #9460, #18018, #15413, #4175, #1037, #9817, #6678, #18288, #8065, #3805, #16628, #3991, #15228, #6859, #13727, #12331, #2709, #2528, #8340, #5291, #8256, #11034, #14000, #16806, #8157, #6946, #2616, #10944, #5200, #4078, #5561, #5384, #15499, #16898, #1314, #2795, #10850, #16717, #946, #1223, #12239, #11209, #13634, #16527, #3902, #1130, #15317, #6766, #5472, #15134, #2437, #9550, #13914, #12514, #18208, #9730, #9906, #2968, #12693, #4346, #15855, #7303, #9994, #7401, #7216, #4263, #4623, #12870, #14368, #13061, #372, #3153, #6013, #10271, #15669, #4441, #11294, #7030, #17167, #178, #1, #12964, #8786, #10082, #5652, #16987, #15578, #8600, #2878, #14089, #11666, #5828, #11474, #4536, #14276, #15760, #8509, #14183, #3060, #1488, #17358, #279, #1668, #7123, #5922, #1580, #8692, #92, #12784, #11568, #17263, #15952, #14470, #8426, #10178, #5744, #1400, #11384, #17073, #1771, #747, #13244, #2234, #2051, #6392, #7682, #17645, #7495, #14565, #3433, #17452, #7586, #4994, #12126, #8988 ),
 ( #3522, #7773, #13519, #10370, #655, #16050, #13344, #12035, #3341, #10650, #14850, #3609, #10467, #13153, #17727, #14661, #8886, #1960, #3248, #464, #14943, #6106, #17820, #6205, #16321, #1865, #6298, #11758, #10553, #4720, #9169, #9257, #564, #5081, #11952, #11853, #10741, #9074, #17550, #4903, #16228, #2143, #7861, #4818, #13434, #16144, #833, #6474, #14753, #924, #9344, #13980, #18093, #16604, #18181, #5364, #8136, #3969, #13798, #15388, #1294, #6925, #9527, #18268, #1018, #6659, #17906, #12307, #3698, #8319, #1106, #3879, #7953, #6838, #2508, #12580, #12489, #3784, #17998, #6746, #16505, #15207, #15294, #9437, #12402, #5538, #5174, #11011, #16415, #5450, #15023, #5269, #10924, #9620, #16690, #11097, #2595, #8228, #13891, #16783, #1202, #4052, #2323, #9704, #2687, #13610, #15110, #6567, #12217, #2413, #10829, #8044, #13705, #8581, #11185, #12941, #9799, #1471, #14159, #4419, #7102, #7282, #2947, #1557, #11363, #11547, #9970, #12764, #13036, #17238, #15738, #69, #15560, #4244, #7376, #15646, #351, #252, #9887, #5634, #1745, #16875, #5898, #17054, #14346, #14254, #7194, #4325, #14441, #4512, #1378, #3129, #12851, #4152, #11451, #3040, #8764, #18361, #158, #11276, #5809, #8669, #16966, #10155, #10061, #15833, #5723, #2777, #1645, #2854, #15481, #8487, #8408, #14064, #7007, #12670, #17141, #8958, #7750, #5989, #3410, #11641, #13319, #7473, #11925, #13410, #11732, #7841, #9052, #1836, #13493, #11831, #10345, #16118, #14728, #2028, #722, #3225, #7652, #16025, #3498 ),
 ( #13131, #2213, #10442, #17620, #4969, #16299, #6368, #3586, #17336, #7562, #633, #8863, #4598, #6271, #4790, #10248, #4880, #12009, #10531, #15927, #14540, #441, #535, #6081, #13219, #16205, #17428, #4694, #17705, #6181, #10625, #3315, #9144, #14823, #9236, #2121, #17527, #14921, #14636, #1939, #5060, #3948, #5431, #17975, #9681, #4034, #13869, #15366, #16391, #5243, #6455, #6722, #12102, #8205, #11077, #10715, #17883, #6639, #9503, #12285, #10991, #2664, #16761, #17799, #3679, #10900, #9325, #14999, #2297, #13677, #7930, #15086, #1175, #18067, #2392, #18160, #16577, #13586, #8298, #3856, #12377, #808, #902, #6816, #6543, #12195, #8023, #15179, #5152, #10809, #2484, #8114, #16481, #5339, #12466, #13773, #3762, #9411, #997, #1085, #16669, #9599, #15274, #2573, #17035, #10038, #14135, #15623, #9779, #5516, #11342, #18247, #5878, #5786, #1536, #2753, #7171, #1448, #2837, #5610, #14046, #12831, #8466, #11525, #8648, #229, #7078, #11161, #13957, #17217, #11428, #11256, #12917, #12746, #17118, #47, #9951, #16853, #6904, #5701, #15456, #18339, #15715, #4489, #1355, #10131, #6986, #15812, #8383, #4130, #16944, #4304, #7257, #2924, #4219, #12647, #4398, #3109, #8557, #1269, #12562, #14326, #9865, #15539, #14233, #134, #3015, #1623, #1915, #6156, #1719, #4579, #1815, #6059, #7450, #3294, #17502, #11805, #14414, #8739, #11711, #11619, #328, #17313, #13108, #5964, #422, #4766, #14613, #17405, #10417, #4668, #10224, #7355, #10321, #7543, #13015, #15902, #3199, #8839, #14516 ) ),
 .UNSPECIFIED., .T., .F., .F. ) 
 B_SPLINE_SURFACE_WITH_KNOTS ( ( 4, 3, 4 ),
 ( 3, 2, 2, 2, 2, 2, 2, 2, 2, 2, 2, 2, 2, 2, 2, 2, 2, 2, 2, 2, 2, 2, 2, 2, 2, 2, 2, 2, 2, 2, 2, 2, 2, 2, 2, 2, 2, 2, 2, 2, 2, 2, 2, 2, 2, 2, 2, 2, 2, 2, 2, 2, 2, 2, 2, 2, 2, 2, 2, 2, 2, 2, 2, 2, 2, 2, 2, 2, 2, 2, 2, 2, 2, 2, 2, 2, 2, 2, 2, 2, 2, 2, 2, 2, 2, 2, 2, 2, 2, 2, 2, 2, 2, 2, 2, 2, 2, 2, 2, 2, 3 ),
 ( 0.000000000000000000, 0.5000000000000000000, 1.000000000000000000 ),
 ( 0.000000000000000000, 0.01000000000000000021, 0.02000000000000000042, 0.02999999999999999889, 0.04000000000000000083, 0.05000000000000000278, 0.05999999999999999778, 0.07000000000000000666, 0.08000000000000000167, 0.08999999999999999667, 0.1000000000000000056, 0.1100000000000000006, 0.1199999999999999956, 0.1300000000000000044, 0.1400000000000000133, 0.1499999999999999944, 0.1600000000000000033, 0.1700000000000000122, 0.1799999999999999933, 0.1900000000000000022, 0.2000000000000000111, 0.2099999999999999922, 0.2200000000000000011, 0.2300000000000000100, 0.2399999999999999911, 0.2500000000000000000, 0.2600000000000000089, 0.2700000000000000178, 0.2800000000000000266, 0.2899999999999999800, 0.2999999999999999889, 0.3099999999999999978, 0.3200000000000000067, 0.3300000000000000155, 0.3400000000000000244, 0.3499999999999999778, 0.3599999999999999867, 0.3699999999999999956, 0.3800000000000000044, 0.3900000000000000133, 0.4000000000000000222, 0.4099999999999999756, 0.4199999999999999845, 0.4299999999999999933, 0.4400000000000000022, 0.4500000000000000111, 0.4600000000000000200, 0.4699999999999999734, 0.4799999999999999822, 0.4899999999999999911, 0.5000000000000000000, 0.5100000000000000089, 0.5200000000000000178, 0.5300000000000000266, 0.5400000000000000355, 0.5500000000000000444, 0.5600000000000000533, 0.5699999999999999512, 0.5799999999999999600, 0.5899999999999999689, 0.5999999999999999778, 0.6099999999999999867, 0.6199999999999999956, 0.6300000000000000044, 0.6400000000000000133, 0.6500000000000000222, 0.6600000000000000311, 0.6700000000000000400, 0.6800000000000000488, 0.6899999999999999467, 0.6999999999999999556, 0.7099999999999999645, 0.7199999999999999734, 0.7299999999999999822, 0.7399999999999999911, 0.7500000000000000000, 0.7600000000000000089, 0.7700000000000000178, 0.7800000000000000266, 0.7900000000000000355, 0.8000000000000000444, 0.8100000000000000533, 0.8199999999999999512, 0.8299999999999999600, 0.8399999999999999689, 0.8499999999999999778, 0.8599999999999999867, 0.8699999999999999956, 0.8800000000000000044, 0.8900000000000000133, 0.9000000000000000222, 0.9100000000000000311, 0.9200000000000000400, 0.9300000000000000488, 0.9399999999999999467, 0.9499999999999999556, 0.9599999999999999645, 0.9699999999999999734, 0.9799999999999999822, 0.9899999999999999911, 1.000000000000000000 ),
 .UNSPECIFIED. ) 
 GEOMETRIC_REPRESENTATION_ITEM ( )  RATIONAL_B_SPLINE_SURFACE ( (
 ( 1.000000000000000000, 0.9510565162951535312, 1.000000000000000000, 0.9510565162951535312, 1.000000000000000000, 0.9510565162951535312, 1.000000000000000000, 0.9510565162951535312, 1.000000000000000000, 0.9510565162951535312, 1.000000000000000000, 0.9510565162951535312, 1.000000000000000000, 0.9510565162951535312, 1.000000000000000000, 0.9510565162951535312, 1.000000000000000000, 0.9510565162951535312, 1.000000000000000000, 0.9510565162951535312, 1.000000000000000000, 0.9510565162951535312, 1.000000000000000000, 0.9510565162951535312, 1.000000000000000000, 0.9510565162951535312, 1.000000000000000000, 0.9510565162951535312, 1.000000000000000000, 0.9510565162951535312, 1.000000000000000000, 0.9510565162951535312, 1.000000000000000000, 0.9510565162951535312, 1.000000000000000000, 0.9510565162951535312, 1.000000000000000000, 0.9510565162951535312, 1.000000000000000000, 0.9510565162951535312, 1.000000000000000000, 0.9510565162951535312, 1.000000000000000000, 0.9510565162951535312, 1.000000000000000000, 0.9510565162951535312, 1.000000000000000000, 0.9510565162951535312, 1.000000000000000000, 0.9510565162951535312, 1.000000000000000000, 0.9510565162951535312, 1.000000000000000000, 0.9510565162951535312, 1.000000000000000000, 0.9510565162951535312, 1.000000000000000000, 0.9510565162951535312, 1.000000000000000000, 0.9510565162951535312, 1.000000000000000000, 0.9510565162951535312, 1.000000000000000000, 0.9510565162951535312, 1.000000000000000000, 0.9510565162951535312, 1.000000000000000000, 0.9510565162951535312, 1.000000000000000000, 0.9510565162951535312, 1.000000000000000000, 0.9510565162951535312, 1.000000000000000000, 0.9510565162951535312, 1.000000000000000000, 0.9510565162951535312, 1.000000000000000000, 0.9510565162951535312, 1.000000000000000000, 0.9510565162951535312, 1.000000000000000000, 0.9510565162951535312, 1.000000000000000000, 0.9510565162951535312, 1.000000000000000000, 0.9510565162951535312, 1.000000000000000000, 0.9510565162951535312, 1.000000000000000000, 0.9510565162951535312, 1.000000000000000000, 0.9510565162951535312, 1.000000000000000000, 0.9510565162951535312, 1.000000000000000000, 0.9510565162951535312, 1.000000000000000000, 0.9510565162951535312, 1.000000000000000000, 0.9510565162951535312, 1.000000000000000000, 0.9510565162951535312, 1.000000000000000000, 0.9510565162951535312, 1.000000000000000000, 0.9510565162951535312, 1.000000000000000000, 0.9510565162951535312, 1.000000000000000000, 0.9510565162951535312, 1.000000000000000000, 0.9510565162951535312, 1.000000000000000000, 0.9510565162951535312, 1.000000000000000000, 0.9510565162951535312, 1.000000000000000000, 0.9510565162951535312, 1.000000000000000000, 0.9510565162951535312, 1.000000000000000000, 0.9510565162951535312, 1.000000000000000000, 0.9510565162951535312, 1.000000000000000000, 0.9510565162951535312, 1.000000000000000000, 0.9510565162951535312, 1.000000000000000000, 0.9510565162951535312, 1.000000000000000000, 0.9510565162951535312, 1.000000000000000000, 0.9510565162951535312, 1.000000000000000000, 0.9510565162951535312, 1.000000000000000000, 0.9510565162951535312, 1.000000000000000000, 0.9510565162951535312, 1.000000000000000000, 0.9510565162951535312, 1.000000000000000000, 0.9510565162951535312, 1.000000000000000000, 0.9510565162951535312, 1.000000000000000000, 0.9510565162951535312, 1.000000000000000000, 0.9510565162951535312, 1.000000000000000000, 0.9510565162951535312, 1.000000000000000000, 0.9510565162951535312, 1.000000000000000000, 0.9510565162951535312, 1.000000000000000000, 0.9510565162951535312, 1.000000000000000000, 0.9510565162951535312, 1.000000000000000000, 0.9510565162951535312, 1.000000000000000000, 0.9510565162951535312, 1.000000000000000000, 0.9510565162951535312, 1.000000000000000000, 0.9510565162951535312, 1.000000000000000000, 0.9510565162951535312, 1.000000000000000000, 0.9510565162951535312, 1.000000000000000000, 0.9510565162951535312, 1.000000000000000000, 0.9510565162951535312, 1.000000000000000000, 0.9510565162951535312, 1.000000000000000000, 0.9510565162951535312, 1.000000000000000000, 0.9510565162951535312, 1.000000000000000000, 0.9510565162951535312, 1.000000000000000000, 0.9510565162951535312, 1.000000000000000000, 0.9510565162951535312, 1.000000000000000000, 0.9510565162951535312, 1.000000000000000000, 0.9510565162951535312, 1.000000000000000000, 0.9510565162951535312, 1.000000000000000000, 0.9510565162951535312, 1.000000000000000000, 0.9510565162951535312, 1.000000000000000000, 0.9510565162951535312, 1.000000000000000000),
 ( 0.3333333333333333703, 0.3170188387650512141, 0.3333333333333333703, 0.3170188387650512141, 0.3333333333333333703, 0.3170188387650512141, 0.3333333333333333703, 0.3170188387650512141, 0.3333333333333333703, 0.3170188387650512141, 0.3333333333333333703, 0.3170188387650512141, 0.3333333333333333703, 0.3170188387650512141, 0.3333333333333333703, 0.3170188387650512141, 0.3333333333333333703, 0.3170188387650512141, 0.3333333333333333703, 0.3170188387650512141, 0.3333333333333333703, 0.3170188387650512141, 0.3333333333333333703, 0.3170188387650512141, 0.3333333333333333703, 0.3170188387650512141, 0.3333333333333333703, 0.3170188387650512141, 0.3333333333333333703, 0.3170188387650512141, 0.3333333333333333703, 0.3170188387650512141, 0.3333333333333333703, 0.3170188387650512141, 0.3333333333333333703, 0.3170188387650512141, 0.3333333333333333703, 0.3170188387650512141, 0.3333333333333333703, 0.3170188387650512141, 0.3333333333333333703, 0.3170188387650512141, 0.3333333333333333703, 0.3170188387650512141, 0.3333333333333333703, 0.3170188387650512141, 0.3333333333333333703, 0.3170188387650512141, 0.3333333333333333703, 0.3170188387650512141, 0.3333333333333333703, 0.3170188387650512141, 0.3333333333333333703, 0.3170188387650512141, 0.3333333333333333703, 0.3170188387650512141, 0.3333333333333333703, 0.3170188387650512141, 0.3333333333333333703, 0.3170188387650512141, 0.3333333333333333703, 0.3170188387650512141, 0.3333333333333333703, 0.3170188387650512141, 0.3333333333333333703, 0.3170188387650512141, 0.3333333333333333703, 0.3170188387650512141, 0.3333333333333333703, 0.3170188387650512141, 0.3333333333333333703, 0.3170188387650512141, 0.3333333333333333703, 0.3170188387650512141, 0.3333333333333333703, 0.3170188387650512141, 0.3333333333333333703, 0.3170188387650512141, 0.3333333333333333703, 0.3170188387650512141, 0.3333333333333333703, 0.3170188387650512141, 0.3333333333333333703, 0.3170188387650512141, 0.3333333333333333703, 0.3170188387650512141, 0.3333333333333333703, 0.3170188387650512141, 0.3333333333333333703, 0.3170188387650512141, 0.3333333333333333703, 0.3170188387650512141, 0.3333333333333333703, 0.3170188387650512141, 0.3333333333333333703, 0.3170188387650512141, 0.3333333333333333703, 0.3170188387650512141, 0.3333333333333333703, 0.3170188387650512141, 0.3333333333333333703, 0.3170188387650512141, 0.3333333333333333703, 0.3170188387650512141, 0.3333333333333333703, 0.3170188387650512141, 0.3333333333333333703, 0.3170188387650512141, 0.3333333333333333703, 0.3170188387650512141, 0.3333333333333333703, 0.3170188387650512141, 0.3333333333333333703, 0.3170188387650512141, 0.3333333333333333703, 0.3170188387650512141, 0.3333333333333333703, 0.3170188387650512141, 0.3333333333333333703, 0.3170188387650512141, 0.3333333333333333703, 0.3170188387650512141, 0.3333333333333333703, 0.3170188387650512141, 0.3333333333333333703, 0.3170188387650512141, 0.3333333333333333703, 0.3170188387650512141, 0.3333333333333333703, 0.3170188387650512141, 0.3333333333333333703, 0.3170188387650512141, 0.3333333333333333703, 0.3170188387650512141, 0.3333333333333333703, 0.3170188387650512141, 0.3333333333333333703, 0.3170188387650512141, 0.3333333333333333703, 0.3170188387650512141, 0.3333333333333333703, 0.3170188387650512141, 0.3333333333333333703, 0.3170188387650512141, 0.3333333333333333703, 0.3170188387650512141, 0.3333333333333333703, 0.3170188387650512141, 0.3333333333333333703, 0.3170188387650512141, 0.3333333333333333703, 0.3170188387650512141, 0.3333333333333333703, 0.3170188387650512141, 0.3333333333333333703, 0.3170188387650512141, 0.3333333333333333703, 0.3170188387650512141, 0.3333333333333333703, 0.3170188387650512141, 0.3333333333333333703, 0.3170188387650512141, 0.3333333333333333703, 0.3170188387650512141, 0.3333333333333333703, 0.3170188387650512141, 0.3333333333333333703, 0.3170188387650512141, 0.3333333333333333703, 0.3170188387650512141, 0.3333333333333333703, 0.3170188387650512141, 0.3333333333333333703, 0.3170188387650512141, 0.3333333333333333703, 0.3170188387650512141, 0.3333333333333333703, 0.3170188387650512141, 0.3333333333333333703, 0.3170188387650512141, 0.3333333333333333703, 0.3170188387650512141, 0.3333333333333333703, 0.3170188387650512141, 0.3333333333333333703, 0.3170188387650512141, 0.3333333333333333703, 0.3170188387650512141, 0.3333333333333333703, 0.3170188387650512141, 0.3333333333333333703, 0.3170188387650512141, 0.3333333333333333703, 0.3170188387650512141, 0.3333333333333333703, 0.3170188387650512141, 0.3333333333333333703, 0.3170188387650512141, 0.3333333333333333703, 0.3170188387650512141, 0.3333333333333333703),
 ( 0.3333333333333333703, 0.3170188387650512141, 0.3333333333333333703, 0.3170188387650512141, 0.3333333333333333703, 0.3170188387650512141, 0.3333333333333333703, 0.3170188387650512141, 0.3333333333333333703, 0.3170188387650512141, 0.3333333333333333703, 0.3170188387650512141, 0.3333333333333333703, 0.3170188387650512141, 0.3333333333333333703, 0.3170188387650512141, 0.3333333333333333703, 0.3170188387650512141, 0.3333333333333333703, 0.3170188387650512141, 0.3333333333333333703, 0.3170188387650512141, 0.3333333333333333703, 0.3170188387650512141, 0.3333333333333333703, 0.3170188387650512141, 0.3333333333333333703, 0.3170188387650512141, 0.3333333333333333703, 0.3170188387650512141, 0.3333333333333333703, 0.3170188387650512141, 0.3333333333333333703, 0.3170188387650512141, 0.3333333333333333703, 0.3170188387650512141, 0.3333333333333333703, 0.3170188387650512141, 0.3333333333333333703, 0.3170188387650512141, 0.3333333333333333703, 0.3170188387650512141, 0.3333333333333333703, 0.3170188387650512141, 0.3333333333333333703, 0.3170188387650512141, 0.3333333333333333703, 0.3170188387650512141, 0.3333333333333333703, 0.3170188387650512141, 0.3333333333333333703, 0.3170188387650512141, 0.3333333333333333703, 0.3170188387650512141, 0.3333333333333333703, 0.3170188387650512141, 0.3333333333333333703, 0.3170188387650512141, 0.3333333333333333703, 0.3170188387650512141, 0.3333333333333333703, 0.3170188387650512141, 0.3333333333333333703, 0.3170188387650512141, 0.3333333333333333703, 0.3170188387650512141, 0.3333333333333333703, 0.3170188387650512141, 0.3333333333333333703, 0.3170188387650512141, 0.3333333333333333703, 0.3170188387650512141, 0.3333333333333333703, 0.3170188387650512141, 0.3333333333333333703, 0.3170188387650512141, 0.3333333333333333703, 0.3170188387650512141, 0.3333333333333333703, 0.3170188387650512141, 0.3333333333333333703, 0.3170188387650512141, 0.3333333333333333703, 0.3170188387650512141, 0.3333333333333333703, 0.3170188387650512141, 0.3333333333333333703, 0.3170188387650512141, 0.3333333333333333703, 0.3170188387650512141, 0.3333333333333333703, 0.3170188387650512141, 0.3333333333333333703, 0.3170188387650512141, 0.3333333333333333703, 0.3170188387650512141, 0.3333333333333333703, 0.3170188387650512141, 0.3333333333333333703, 0.3170188387650512141, 0.3333333333333333703, 0.3170188387650512141, 0.3333333333333333703, 0.3170188387650512141, 0.3333333333333333703, 0.3170188387650512141, 0.3333333333333333703, 0.3170188387650512141, 0.3333333333333333703, 0.3170188387650512141, 0.3333333333333333703, 0.3170188387650512141, 0.3333333333333333703, 0.3170188387650512141, 0.3333333333333333703, 0.3170188387650512141, 0.3333333333333333703, 0.3170188387650512141, 0.3333333333333333703, 0.3170188387650512141, 0.3333333333333333703, 0.3170188387650512141, 0.3333333333333333703, 0.3170188387650512141, 0.3333333333333333703, 0.3170188387650512141, 0.3333333333333333703, 0.3170188387650512141, 0.3333333333333333703, 0.3170188387650512141, 0.3333333333333333703, 0.3170188387650512141, 0.3333333333333333703, 0.3170188387650512141, 0.3333333333333333703, 0.3170188387650512141, 0.3333333333333333703, 0.3170188387650512141, 0.3333333333333333703, 0.3170188387650512141, 0.3333333333333333703, 0.3170188387650512141, 0.3333333333333333703, 0.3170188387650512141, 0.3333333333333333703, 0.3170188387650512141, 0.3333333333333333703, 0.3170188387650512141, 0.3333333333333333703, 0.3170188387650512141, 0.3333333333333333703, 0.3170188387650512141, 0.3333333333333333703, 0.3170188387650512141, 0.3333333333333333703, 0.3170188387650512141, 0.3333333333333333703, 0.3170188387650512141, 0.3333333333333333703, 0.3170188387650512141, 0.3333333333333333703, 0.3170188387650512141, 0.3333333333333333703, 0.3170188387650512141, 0.3333333333333333703, 0.3170188387650512141, 0.3333333333333333703, 0.3170188387650512141, 0.3333333333333333703, 0.3170188387650512141, 0.3333333333333333703, 0.3170188387650512141, 0.3333333333333333703, 0.3170188387650512141, 0.3333333333333333703, 0.3170188387650512141, 0.3333333333333333703, 0.3170188387650512141, 0.3333333333333333703, 0.3170188387650512141, 0.3333333333333333703, 0.3170188387650512141, 0.3333333333333333703, 0.3170188387650512141, 0.3333333333333333703, 0.3170188387650512141, 0.3333333333333333703, 0.3170188387650512141, 0.3333333333333333703, 0.3170188387650512141, 0.3333333333333333703, 0.3170188387650512141, 0.3333333333333333703, 0.3170188387650512141, 0.3333333333333333703, 0.3170188387650512141, 0.3333333333333333703, 0.3170188387650512141, 0.3333333333333333703, 0.3170188387650512141, 0.3333333333333333703),
 ( 1.000000000000000000, 0.9510565162951535312, 1.000000000000000000, 0.9510565162951535312, 1.000000000000000000, 0.9510565162951535312, 1.000000000000000000, 0.9510565162951535312, 1.000000000000000000, 0.9510565162951535312, 1.000000000000000000, 0.9510565162951535312, 1.000000000000000000, 0.9510565162951535312, 1.000000000000000000, 0.9510565162951535312, 1.000000000000000000, 0.9510565162951535312, 1.000000000000000000, 0.9510565162951535312, 1.000000000000000000, 0.9510565162951535312, 1.000000000000000000, 0.9510565162951535312, 1.000000000000000000, 0.9510565162951535312, 1.000000000000000000, 0.9510565162951535312, 1.000000000000000000, 0.9510565162951535312, 1.000000000000000000, 0.9510565162951535312, 1.000000000000000000, 0.9510565162951535312, 1.000000000000000000, 0.9510565162951535312, 1.000000000000000000, 0.9510565162951535312, 1.000000000000000000, 0.9510565162951535312, 1.000000000000000000, 0.9510565162951535312, 1.000000000000000000, 0.9510565162951535312, 1.000000000000000000, 0.9510565162951535312, 1.000000000000000000, 0.9510565162951535312, 1.000000000000000000, 0.9510565162951535312, 1.000000000000000000, 0.9510565162951535312, 1.000000000000000000, 0.9510565162951535312, 1.000000000000000000, 0.9510565162951535312, 1.000000000000000000, 0.9510565162951535312, 1.000000000000000000, 0.9510565162951535312, 1.000000000000000000, 0.9510565162951535312, 1.000000000000000000, 0.9510565162951535312, 1.000000000000000000, 0.9510565162951535312, 1.000000000000000000, 0.9510565162951535312, 1.000000000000000000, 0.9510565162951535312, 1.000000000000000000, 0.9510565162951535312, 1.000000000000000000, 0.9510565162951535312, 1.000000000000000000, 0.9510565162951535312, 1.000000000000000000, 0.9510565162951535312, 1.000000000000000000, 0.9510565162951535312, 1.000000000000000000, 0.9510565162951535312, 1.000000000000000000, 0.9510565162951535312, 1.000000000000000000, 0.9510565162951535312, 1.000000000000000000, 0.9510565162951535312, 1.000000000000000000, 0.9510565162951535312, 1.000000000000000000, 0.9510565162951535312, 1.000000000000000000, 0.9510565162951535312, 1.000000000000000000, 0.9510565162951535312, 1.000000000000000000, 0.9510565162951535312, 1.000000000000000000, 0.9510565162951535312, 1.000000000000000000, 0.9510565162951535312, 1.000000000000000000, 0.9510565162951535312, 1.000000000000000000, 0.9510565162951535312, 1.000000000000000000, 0.9510565162951535312, 1.000000000000000000, 0.9510565162951535312, 1.000000000000000000, 0.9510565162951535312, 1.000000000000000000, 0.9510565162951535312, 1.000000000000000000, 0.9510565162951535312, 1.000000000000000000, 0.9510565162951535312, 1.000000000000000000, 0.9510565162951535312, 1.000000000000000000, 0.9510565162951535312, 1.000000000000000000, 0.9510565162951535312, 1.000000000000000000, 0.9510565162951535312, 1.000000000000000000, 0.9510565162951535312, 1.000000000000000000, 0.9510565162951535312, 1.000000000000000000, 0.9510565162951535312, 1.000000000000000000, 0.9510565162951535312, 1.000000000000000000, 0.9510565162951535312, 1.000000000000000000, 0.9510565162951535312, 1.000000000000000000, 0.9510565162951535312, 1.000000000000000000, 0.9510565162951535312, 1.000000000000000000, 0.9510565162951535312, 1.000000000000000000, 0.9510565162951535312, 1.000000000000000000, 0.9510565162951535312, 1.000000000000000000, 0.9510565162951535312, 1.000000000000000000, 0.9510565162951535312, 1.000000000000000000, 0.9510565162951535312, 1.000000000000000000, 0.9510565162951535312, 1.000000000000000000, 0.9510565162951535312, 1.000000000000000000, 0.9510565162951535312, 1.000000000000000000, 0.9510565162951535312, 1.000000000000000000, 0.9510565162951535312, 1.000000000000000000, 0.9510565162951535312, 1.000000000000000000, 0.9510565162951535312, 1.000000000000000000, 0.9510565162951535312, 1.000000000000000000, 0.9510565162951535312, 1.000000000000000000, 0.9510565162951535312, 1.000000000000000000, 0.9510565162951535312, 1.000000000000000000, 0.9510565162951535312, 1.000000000000000000, 0.9510565162951535312, 1.000000000000000000, 0.9510565162951535312, 1.000000000000000000, 0.9510565162951535312, 1.000000000000000000, 0.9510565162951535312, 1.000000000000000000, 0.9510565162951535312, 1.000000000000000000, 0.9510565162951535312, 1.000000000000000000, 0.9510565162951535312, 1.000000000000000000, 0.9510565162951535312, 1.000000000000000000, 0.9510565162951535312, 1.000000000000000000, 0.9510565162951535312, 1.000000000000000000, 0.9510565162951535312, 1.000000000000000000),
 ( 0.3333333333333333703, 0.3170188387650512141, 0.3333333333333333703, 0.3170188387650512141, 0.3333333333333333703, 0.3170188387650512141, 0.3333333333333333703, 0.3170188387650512141, 0.3333333333333333703, 0.3170188387650512141, 0.3333333333333333703, 0.3170188387650512141, 0.3333333333333333703, 0.3170188387650512141, 0.3333333333333333703, 0.3170188387650512141, 0.3333333333333333703, 0.3170188387650512141, 0.3333333333333333703, 0.3170188387650512141, 0.3333333333333333703, 0.3170188387650512141, 0.3333333333333333703, 0.3170188387650512141, 0.3333333333333333703, 0.3170188387650512141, 0.3333333333333333703, 0.3170188387650512141, 0.3333333333333333703, 0.3170188387650512141, 0.3333333333333333703, 0.3170188387650512141, 0.3333333333333333703, 0.3170188387650512141, 0.3333333333333333703, 0.3170188387650512141, 0.3333333333333333703, 0.3170188387650512141, 0.3333333333333333703, 0.3170188387650512141, 0.3333333333333333703, 0.3170188387650512141, 0.3333333333333333703, 0.3170188387650512141, 0.3333333333333333703, 0.3170188387650512141, 0.3333333333333333703, 0.3170188387650512141, 0.3333333333333333703, 0.3170188387650512141, 0.3333333333333333703, 0.3170188387650512141, 0.3333333333333333703, 0.3170188387650512141, 0.3333333333333333703, 0.3170188387650512141, 0.3333333333333333703, 0.3170188387650512141, 0.3333333333333333703, 0.3170188387650512141, 0.3333333333333333703, 0.3170188387650512141, 0.3333333333333333703, 0.3170188387650512141, 0.3333333333333333703, 0.3170188387650512141, 0.3333333333333333703, 0.3170188387650512141, 0.3333333333333333703, 0.3170188387650512141, 0.3333333333333333703, 0.3170188387650512141, 0.3333333333333333703, 0.3170188387650512141, 0.3333333333333333703, 0.3170188387650512141, 0.3333333333333333703, 0.3170188387650512141, 0.3333333333333333703, 0.3170188387650512141, 0.3333333333333333703, 0.3170188387650512141, 0.3333333333333333703, 0.3170188387650512141, 0.3333333333333333703, 0.3170188387650512141, 0.3333333333333333703, 0.3170188387650512141, 0.3333333333333333703, 0.3170188387650512141, 0.3333333333333333703, 0.3170188387650512141, 0.3333333333333333703, 0.3170188387650512141, 0.3333333333333333703, 0.3170188387650512141, 0.3333333333333333703, 0.3170188387650512141, 0.3333333333333333703, 0.3170188387650512141, 0.3333333333333333703, 0.3170188387650512141, 0.3333333333333333703, 0.3170188387650512141, 0.3333333333333333703, 0.3170188387650512141, 0.3333333333333333703, 0.3170188387650512141, 0.3333333333333333703, 0.3170188387650512141, 0.3333333333333333703, 0.3170188387650512141, 0.3333333333333333703, 0.3170188387650512141, 0.3333333333333333703, 0.3170188387650512141, 0.3333333333333333703, 0.3170188387650512141, 0.3333333333333333703, 0.3170188387650512141, 0.3333333333333333703, 0.3170188387650512141, 0.3333333333333333703, 0.3170188387650512141, 0.3333333333333333703, 0.3170188387650512141, 0.3333333333333333703, 0.3170188387650512141, 0.3333333333333333703, 0.3170188387650512141, 0.3333333333333333703, 0.3170188387650512141, 0.3333333333333333703, 0.3170188387650512141, 0.3333333333333333703, 0.3170188387650512141, 0.3333333333333333703, 0.3170188387650512141, 0.3333333333333333703, 0.3170188387650512141, 0.3333333333333333703, 0.3170188387650512141, 0.3333333333333333703, 0.3170188387650512141, 0.3333333333333333703, 0.3170188387650512141, 0.3333333333333333703, 0.3170188387650512141, 0.3333333333333333703, 0.3170188387650512141, 0.3333333333333333703, 0.3170188387650512141, 0.3333333333333333703, 0.3170188387650512141, 0.3333333333333333703, 0.3170188387650512141, 0.3333333333333333703, 0.3170188387650512141, 0.3333333333333333703, 0.3170188387650512141, 0.3333333333333333703, 0.3170188387650512141, 0.3333333333333333703, 0.3170188387650512141, 0.3333333333333333703, 0.3170188387650512141, 0.3333333333333333703, 0.3170188387650512141, 0.3333333333333333703, 0.3170188387650512141, 0.3333333333333333703, 0.3170188387650512141, 0.3333333333333333703, 0.3170188387650512141, 0.3333333333333333703, 0.3170188387650512141, 0.3333333333333333703, 0.3170188387650512141, 0.3333333333333333703, 0.3170188387650512141, 0.3333333333333333703, 0.3170188387650512141, 0.3333333333333333703, 0.3170188387650512141, 0.3333333333333333703, 0.3170188387650512141, 0.3333333333333333703, 0.3170188387650512141, 0.3333333333333333703, 0.3170188387650512141, 0.3333333333333333703, 0.3170188387650512141, 0.3333333333333333703, 0.3170188387650512141, 0.3333333333333333703, 0.3170188387650512141, 0.3333333333333333703, 0.3170188387650512141, 0.3333333333333333703, 0.3170188387650512141, 0.3333333333333333703),
 ( 0.3333333333333333703, 0.3170188387650512141, 0.3333333333333333703, 0.3170188387650512141, 0.3333333333333333703, 0.3170188387650512141, 0.3333333333333333703, 0.3170188387650512141, 0.3333333333333333703, 0.3170188387650512141, 0.3333333333333333703, 0.3170188387650512141, 0.3333333333333333703, 0.3170188387650512141, 0.3333333333333333703, 0.3170188387650512141, 0.3333333333333333703, 0.3170188387650512141, 0.3333333333333333703, 0.3170188387650512141, 0.3333333333333333703, 0.3170188387650512141, 0.3333333333333333703, 0.3170188387650512141, 0.3333333333333333703, 0.3170188387650512141, 0.3333333333333333703, 0.3170188387650512141, 0.3333333333333333703, 0.3170188387650512141, 0.3333333333333333703, 0.3170188387650512141, 0.3333333333333333703, 0.3170188387650512141, 0.3333333333333333703, 0.3170188387650512141, 0.3333333333333333703, 0.3170188387650512141, 0.3333333333333333703, 0.3170188387650512141, 0.3333333333333333703, 0.3170188387650512141, 0.3333333333333333703, 0.3170188387650512141, 0.3333333333333333703, 0.3170188387650512141, 0.3333333333333333703, 0.3170188387650512141, 0.3333333333333333703, 0.3170188387650512141, 0.3333333333333333703, 0.3170188387650512141, 0.3333333333333333703, 0.3170188387650512141, 0.3333333333333333703, 0.3170188387650512141, 0.3333333333333333703, 0.3170188387650512141, 0.3333333333333333703, 0.3170188387650512141, 0.3333333333333333703, 0.3170188387650512141, 0.3333333333333333703, 0.3170188387650512141, 0.3333333333333333703, 0.3170188387650512141, 0.3333333333333333703, 0.3170188387650512141, 0.3333333333333333703, 0.3170188387650512141, 0.3333333333333333703, 0.3170188387650512141, 0.3333333333333333703, 0.3170188387650512141, 0.3333333333333333703, 0.3170188387650512141, 0.3333333333333333703, 0.3170188387650512141, 0.3333333333333333703, 0.3170188387650512141, 0.3333333333333333703, 0.3170188387650512141, 0.3333333333333333703, 0.3170188387650512141, 0.3333333333333333703, 0.3170188387650512141, 0.3333333333333333703, 0.3170188387650512141, 0.3333333333333333703, 0.3170188387650512141, 0.3333333333333333703, 0.3170188387650512141, 0.3333333333333333703, 0.3170188387650512141, 0.3333333333333333703, 0.3170188387650512141, 0.3333333333333333703, 0.3170188387650512141, 0.3333333333333333703, 0.3170188387650512141, 0.3333333333333333703, 0.3170188387650512141, 0.3333333333333333703, 0.3170188387650512141, 0.3333333333333333703, 0.3170188387650512141, 0.3333333333333333703, 0.3170188387650512141, 0.3333333333333333703, 0.3170188387650512141, 0.3333333333333333703, 0.3170188387650512141, 0.3333333333333333703, 0.3170188387650512141, 0.3333333333333333703, 0.3170188387650512141, 0.3333333333333333703, 0.3170188387650512141, 0.3333333333333333703, 0.3170188387650512141, 0.3333333333333333703, 0.3170188387650512141, 0.3333333333333333703, 0.3170188387650512141, 0.3333333333333333703, 0.3170188387650512141, 0.3333333333333333703, 0.3170188387650512141, 0.3333333333333333703, 0.3170188387650512141, 0.3333333333333333703, 0.3170188387650512141, 0.3333333333333333703, 0.3170188387650512141, 0.3333333333333333703, 0.3170188387650512141, 0.3333333333333333703, 0.3170188387650512141, 0.3333333333333333703, 0.3170188387650512141, 0.3333333333333333703, 0.3170188387650512141, 0.3333333333333333703, 0.3170188387650512141, 0.3333333333333333703, 0.3170188387650512141, 0.3333333333333333703, 0.3170188387650512141, 0.3333333333333333703, 0.3170188387650512141, 0.3333333333333333703, 0.3170188387650512141, 0.3333333333333333703, 0.3170188387650512141, 0.3333333333333333703, 0.3170188387650512141, 0.3333333333333333703, 0.3170188387650512141, 0.3333333333333333703, 0.3170188387650512141, 0.3333333333333333703, 0.3170188387650512141, 0.3333333333333333703, 0.3170188387650512141, 0.3333333333333333703, 0.3170188387650512141, 0.3333333333333333703, 0.3170188387650512141, 0.3333333333333333703, 0.3170188387650512141, 0.3333333333333333703, 0.3170188387650512141, 0.3333333333333333703, 0.3170188387650512141, 0.3333333333333333703, 0.3170188387650512141, 0.3333333333333333703, 0.3170188387650512141, 0.3333333333333333703, 0.3170188387650512141, 0.3333333333333333703, 0.3170188387650512141, 0.3333333333333333703, 0.3170188387650512141, 0.3333333333333333703, 0.3170188387650512141, 0.3333333333333333703, 0.3170188387650512141, 0.3333333333333333703, 0.3170188387650512141, 0.3333333333333333703, 0.3170188387650512141, 0.3333333333333333703, 0.3170188387650512141, 0.3333333333333333703, 0.3170188387650512141, 0.3333333333333333703, 0.3170188387650512141, 0.3333333333333333703, 0.3170188387650512141, 0.3333333333333333703),
 ( 1.000000000000000000, 0.9510565162951535312, 1.000000000000000000, 0.9510565162951535312, 1.000000000000000000, 0.9510565162951535312, 1.000000000000000000, 0.9510565162951535312, 1.000000000000000000, 0.9510565162951535312, 1.000000000000000000, 0.9510565162951535312, 1.000000000000000000, 0.9510565162951535312, 1.000000000000000000, 0.9510565162951535312, 1.000000000000000000, 0.9510565162951535312, 1.000000000000000000, 0.9510565162951535312, 1.000000000000000000, 0.9510565162951535312, 1.000000000000000000, 0.9510565162951535312, 1.000000000000000000, 0.9510565162951535312, 1.000000000000000000, 0.9510565162951535312, 1.000000000000000000, 0.9510565162951535312, 1.000000000000000000, 0.9510565162951535312, 1.000000000000000000, 0.9510565162951535312, 1.000000000000000000, 0.9510565162951535312, 1.000000000000000000, 0.9510565162951535312, 1.000000000000000000, 0.9510565162951535312, 1.000000000000000000, 0.9510565162951535312, 1.000000000000000000, 0.9510565162951535312, 1.000000000000000000, 0.9510565162951535312, 1.000000000000000000, 0.9510565162951535312, 1.000000000000000000, 0.9510565162951535312, 1.000000000000000000, 0.9510565162951535312, 1.000000000000000000, 0.9510565162951535312, 1.000000000000000000, 0.9510565162951535312, 1.000000000000000000, 0.9510565162951535312, 1.000000000000000000, 0.9510565162951535312, 1.000000000000000000, 0.9510565162951535312, 1.000000000000000000, 0.9510565162951535312, 1.000000000000000000, 0.9510565162951535312, 1.000000000000000000, 0.9510565162951535312, 1.000000000000000000, 0.9510565162951535312, 1.000000000000000000, 0.9510565162951535312, 1.000000000000000000, 0.9510565162951535312, 1.000000000000000000, 0.9510565162951535312, 1.000000000000000000, 0.9510565162951535312, 1.000000000000000000, 0.9510565162951535312, 1.000000000000000000, 0.9510565162951535312, 1.000000000000000000, 0.9510565162951535312, 1.000000000000000000, 0.9510565162951535312, 1.000000000000000000, 0.9510565162951535312, 1.000000000000000000, 0.9510565162951535312, 1.000000000000000000, 0.9510565162951535312, 1.000000000000000000, 0.9510565162951535312, 1.000000000000000000, 0.9510565162951535312, 1.000000000000000000, 0.9510565162951535312, 1.000000000000000000, 0.9510565162951535312, 1.000000000000000000, 0.9510565162951535312, 1.000000000000000000, 0.9510565162951535312, 1.000000000000000000, 0.9510565162951535312, 1.000000000000000000, 0.9510565162951535312, 1.000000000000000000, 0.9510565162951535312, 1.000000000000000000, 0.9510565162951535312, 1.000000000000000000, 0.9510565162951535312, 1.000000000000000000, 0.9510565162951535312, 1.000000000000000000, 0.9510565162951535312, 1.000000000000000000, 0.9510565162951535312, 1.000000000000000000, 0.9510565162951535312, 1.000000000000000000, 0.9510565162951535312, 1.000000000000000000, 0.9510565162951535312, 1.000000000000000000, 0.9510565162951535312, 1.000000000000000000, 0.9510565162951535312, 1.000000000000000000, 0.9510565162951535312, 1.000000000000000000, 0.9510565162951535312, 1.000000000000000000, 0.9510565162951535312, 1.000000000000000000, 0.9510565162951535312, 1.000000000000000000, 0.9510565162951535312, 1.000000000000000000, 0.9510565162951535312, 1.000000000000000000, 0.9510565162951535312, 1.000000000000000000, 0.9510565162951535312, 1.000000000000000000, 0.9510565162951535312, 1.000000000000000000, 0.9510565162951535312, 1.000000000000000000, 0.9510565162951535312, 1.000000000000000000, 0.9510565162951535312, 1.000000000000000000, 0.9510565162951535312, 1.000000000000000000, 0.9510565162951535312, 1.000000000000000000, 0.9510565162951535312, 1.000000000000000000, 0.9510565162951535312, 1.000000000000000000, 0.9510565162951535312, 1.000000000000000000, 0.9510565162951535312, 1.000000000000000000, 0.9510565162951535312, 1.000000000000000000, 0.9510565162951535312, 1.000000000000000000, 0.9510565162951535312, 1.000000000000000000, 0.9510565162951535312, 1.000000000000000000, 0.9510565162951535312, 1.000000000000000000, 0.9510565162951535312, 1.000000000000000000, 0.9510565162951535312, 1.000000000000000000, 0.9510565162951535312, 1.000000000000000000, 0.9510565162951535312, 1.000000000000000000, 0.9510565162951535312, 1.000000000000000000, 0.9510565162951535312, 1.000000000000000000, 0.9510565162951535312, 1.000000000000000000, 0.9510565162951535312, 1.000000000000000000, 0.9510565162951535312, 1.000000000000000000, 0.9510565162951535312, 1.000000000000000000, 0.9510565162951535312, 1.000000000000000000, 0.9510565162951535312, 1.000000000000000000) ) ) 
 REPRESENTATION_ITEM ( '' )  SURFACE ( )  );
#12735=CARTESIAN_POINT ( 'NONE',  ( -1.127657100080120323, 15.00000000000000888, -3.191926594068459799 ) ) ;
#12738=CARTESIAN_POINT ( 'NONE',  ( 2.481649420246391902, 20.87819992234355126, 0.8687765177875720335 ) ) ;
#12740=CARTESIAN_POINT ( 'NONE',  ( -3.518350579753630747, 18.12180007765648071, -1.080741659609802729 ) ) ;
#12746=CARTESIAN_POINT ( 'NONE',  ( 2.211161402132902243, 32.12180007765647360, 2.942372952327172442 ) ) ;
#12757=CARTESIAN_POINT ( 'NONE',  ( 0.7188294034286049072, 23.74680007765648426, -2.395093729190366005 ) ) ;
#12761=CARTESIAN_POINT ( 'NONE',  ( -1.989345975306457071, 37.25319992234354061, -1.515154207786300944 ) ) ;
#12764=CARTESIAN_POINT ( 'NONE',  ( 2.733110507866247652, 31.37180007765647716, -3.862833514489153686 ) ) ;
#12778=CARTESIAN_POINT ( 'NONE',  ( -3.607379964056363075, 17.25319992234354416, -2.690724712371229899 ) ) ;
#12779=CARTESIAN_POINT ( 'NONE',  ( 0.05938372350920110426, 25.12819992234354416, -3.680117784833935701 ) ) ;
#12782=CARTESIAN_POINT ( 'NONE',  ( -0.7188294034286043521, 34.99680007765648071, 2.395093729190366005 ) ) ;
#12784=CARTESIAN_POINT ( 'NONE',  ( 1.336863392178569754, 36.25319992234354771, 4.297206761780648421 ) ) ;
#12790=CARTESIAN_POINT ( 'NONE',  ( 2.211161402132902243, 24.62180007765647716, 2.942372952327172442 ) ) ;
#12794=CARTESIAN_POINT ( 'NONE',  ( 3.607379964056306676, 26.49680007765647716, -2.690724712371305838 ) ) ;
#12799=CARTESIAN_POINT ( 'NONE',  ( -2.211161402132902243, 20.87180007765647716, -2.942372952327172886 ) ) ;
#12805=CARTESIAN_POINT ( 'NONE',  ( -3.500000000000000444, 22.00319992234354416, -0.05647727720529563400 ) ) ;
#12807=CARTESIAN_POINT ( 'NONE',  ( -1.989345975306426206, 17.74680007765647716, 1.515154207786343799 ) ) ;
#12808=CARTESIAN_POINT ( 'NONE',  ( 1.135272562821020070, 35.25319992234354771, -3.311245368580577164 ) ) ;
#12823=CARTESIAN_POINT ( 'NONE',  ( 0.7188294034286553114, 21.25319992234354771, 2.395093729190349130 ) ) ;
#12825=CARTESIAN_POINT ( 'NONE',  ( -3.518350579753630747, 15.62180007765647538, -1.080741659609802729 ) ) ;
#12831=CARTESIAN_POINT ( 'NONE',  ( -3.518350579753630747, 30.62180007765647716, -1.080741659609802729 ) ) ;
#12841=DIRECTION ( 'NONE',  ( 1.047034504275222322E-14, -0.1129545544106647231, 0.9936001553129348851 ) ) ;
#12843=CARTESIAN_POINT ( 'NONE',  ( 2.481649420246374138, 24.12180007765648071, -0.8687765177876252132 ) ) ;
#12845=CARTESIAN_POINT ( 'NONE',  ( -3.481649420246370141, 20.37180007765647716, 1.193696214020542268 ) ) ;
#12848=CARTESIAN_POINT ( 'NONE',  ( -2.798362969681409851, 14.75319992234354594, -2.102939460078765421 ) ) ;
#12851=CARTESIAN_POINT ( 'NONE',  ( 3.673772985318219053, 34.49680007765647360, 2.599342558260951730 ) ) ;
#12866=CARTESIAN_POINT ( 'NONE',  ( -0.05938372350918959958, 16.37819992234354416, 4.731580009072201776 ) ) ;
#12867=CARTESIAN_POINT ( 'NONE',  ( 2.211161402132839182, 30.37819992234354416, -2.942372952327217739 ) ) ;
#12868=CARTESIAN_POINT ( 'NONE',  ( 0.05938372350926800214, 39.87180007765647360, 2.628655560595669183 ) ) ;
#12870=CARTESIAN_POINT ( 'NONE',  ( 2.733110507866328920, 31.12819992234354416, 3.862833514489095510 ) ) ;
#12875=CARTESIAN_POINT ( 'NONE',  ( 2.211161402132902243, 27.12180007765647360, 2.942372952327172442 ) ) ;
#12880=CARTESIAN_POINT ( 'NONE',  ( 1.444289557196047680, 34.74680007765647360, 4.262301884875704161 ) ) ;
#12883=ORIENTED_EDGE ( 'NONE', *, *, #2547, .T. ) ;
#12885=CARTESIAN_POINT ( 'NONE',  ( -1.027846397803541700, 27.49680007765648071, 3.346150245485522312 ) ) ;
#12890=CARTESIAN_POINT ( 'NONE',  ( 2.864755990943222308, 20.50319992234354416, -2.011557305968548093 ) ) ;
#12893=CARTESIAN_POINT ( 'NONE',  ( 2.115076519116362963, 36.37180007765648782, -3.012182706137107147 ) ) ;
#12894=CARTESIAN_POINT ( 'NONE',  ( -3.500000000000000444, 32.00319992234354771, -0.05647727720529563400 ) ) ;
#12908=CARTESIAN_POINT ( 'NONE',  ( 2.500000000000001332, 20.75319992234354771, 0.05647727720530566764 ) ) ;
#12917=CARTESIAN_POINT ( 'NONE',  ( 2.864755990943265829, 31.99680007765647716, 2.011557305968487697 ) ) ;
#12928=CARTESIAN_POINT ( 'NONE',  ( -0.7188294034286043521, 24.99680007765647716, 2.395093729190366005 ) ) ;
#12930=CARTESIAN_POINT ( 'NONE',  ( 3.481649420246370141, 24.12180007765648071, -1.193696214020541602 ) ) ;
#12937=CARTESIAN_POINT ( 'NONE',  ( 2.055738996568281518, 33.00319992234354771, -1.423772053676066518 ) ) ;
#12941=CARTESIAN_POINT ( 'NONE',  ( 0.05938372350929014415, 29.87180007765647005, 4.731580009072201776 ) ) ;
#12959=CARTESIAN_POINT ( 'NONE',  ( 1.444289557195957086, 17.75319992234354061, -4.262301884875733471 ) ) ;
#12960=CARTESIAN_POINT ( 'NONE',  ( 1.027846397803612311, 26.25319992234354771, 3.346150245485499219 ) ) ;
#12961=CARTESIAN_POINT ( 'NONE',  ( 2.518350579753628971, 39.37180007765647360, 0.7558219633769073242 ) ) ;
#12964=CARTESIAN_POINT ( 'NONE',  ( 2.829195390882724759, 32.87819992234354771, -3.793023760679264278 ) ) ;
#12969=CARTESIAN_POINT ( 'NONE',  ( 0.05938372350927906274, 29.87180007765648071, 3.680117784833935701 ) ) ;
#12972=CARTESIAN_POINT ( 'NONE',  ( -3.607379964056306676, 32.74680007765648071, 2.690724712371306282 ) ) ;
#12978=CARTESIAN_POINT ( 'NONE',  ( -2.798362969681365886, 20.24680007765647716, 2.102939460078824929 ) ) ;
#12984=CARTESIAN_POINT ( 'NONE',  ( -0.05938372350920063936, 18.87819992234354771, 3.680117784833935701 ) ) ;
#12987=CARTESIAN_POINT ( 'NONE',  ( 1.989345975306426206, 16.49680007765648071, -1.515154207786343799 ) ) ;
#12989=CARTESIAN_POINT ( 'NONE',  ( 3.500000000000000444, 35.75319992234354771, 0.05647727720529520379 ) ) ;
#13000=VERTEX_POINT ( 'NONE', #3620 ) ;
#13006=CARTESIAN_POINT ( 'NONE',  ( 1.593127413382953383, 22.87819992234354771, -2.091722143975172532 ) ) ;
#13008=CARTESIAN_POINT ( 'NONE',  ( 2.798362969681366330, 16.49680007765647716, -2.102939460078824929 ) ) ;
#13009=CARTESIAN_POINT ( 'NONE',  ( 4.481649420246366589, 16.62180007765647716, -1.518615910253458212 ) ) ;
#13015=CARTESIAN_POINT ( 'NONE',  ( -1.027846397803541700, 39.99680007765648071, 3.346150245485522312 ) ) ;
#13026=CARTESIAN_POINT ( 'NONE',  ( -2.055738996568313048, 25.74680007765648426, -1.423772053676023441 ) ) ;
#13028=CARTESIAN_POINT ( 'NONE',  ( 3.500000000000000444, 19.24680007765648071, -0.05647727720536935281 ) ) ;
#13033=CARTESIAN_POINT ( 'NONE',  ( 2.211161402132839626, 17.87819992234354771, -2.942372952327218183 ) ) ;
#13036=CARTESIAN_POINT ( 'NONE',  ( 3.607379964056306676, 31.49680007765647716, -2.690724712371305838 ) ) ;
#13037=VERTEX_POINT ( 'NONE', #12047 ) ;
#13057=CARTESIAN_POINT ( 'NONE',  ( 4.499999999999999112, 25.75319992234354771, 0.05647727720528474687 ) ) ;
#13058=CARTESIAN_POINT ( 'NONE',  ( 0.05938372350920110426, 30.12819992234354416, -3.680117784833935701 ) ) ;
#13059=CARTESIAN_POINT ( 'NONE',  ( 1.989345975306457071, 16.00319992234354771, 1.515154207786300500 ) ) ;
#13061=CARTESIAN_POINT ( 'NONE',  ( -0.05938372350918959958, 31.37819992234354061, 4.731580009072201776 ) ) ;
#13065=CARTESIAN_POINT ( 'NONE',  ( -2.211161402132902243, 30.87180007765647716, -2.942372952327172886 ) ) ;
#13069=CARTESIAN_POINT ( 'NONE',  ( 3.673772985318219053, 31.99680007765648071, 2.599342558260951730 ) ) ;
#13071=EDGE_LOOP ( 'NONE', ( #11654, #16448, #2677, #10775, #8086 ) ) ;
#13072=CARTESIAN_POINT ( 'NONE',  ( -3.481649420246369697, 30.37180007765647005, 1.193696214020542490 ) ) ;
#13077=CARTESIAN_POINT ( 'NONE',  ( -3.481649420246394122, 24.62819992234354061, -1.193696214020467883 ) ) ;
#13080=CARTESIAN_POINT ( 'NONE',  ( -3.500000000000000444, 35.49680007765648071, 0.05647727720536892260 ) ) ;
#13082=CARTESIAN_POINT ( 'NONE',  ( -2.864755990943222308, 31.75319992234354416, 2.011557305968548093 ) ) ;
#13100=EDGE_LOOP ( 'NONE', ( #5118, #3857 ) ) ;
#13101=CARTESIAN_POINT ( 'NONE',  ( -1.989345975306457071, 22.25319992234354771, -1.515154207786300944 ) ) ;
#13103=CARTESIAN_POINT ( 'NONE',  ( -0.05938372350927861171, 16.12180007765647716, -3.680117784833935701 ) ) ;
#13108=CARTESIAN_POINT ( 'NONE',  ( -1.135272562821090014, 38.49680007765647360, -3.311245368580554072 ) ) ;
#13122=CARTESIAN_POINT ( 'NONE',  ( -2.481649420246374138, 25.37180007765648426, 0.8687765177876256573 ) ) ;
#13124=CARTESIAN_POINT ( 'NONE',  ( 3.500000000000000444, 24.24680007765647716, -0.05647727720536935281 ) ) ;
#13128=CARTESIAN_POINT ( 'NONE',  ( -3.481649420246394122, 22.12819992234353705, -1.193696214020467883 ) ) ;
#13131=CARTESIAN_POINT ( 'NONE',  ( -3.500000000000000444, 15.49680007765647893, 0.05647727720536892260 ) ) ;
#13149=CARTESIAN_POINT ( 'NONE',  ( -2.829195390882724315, 26.62819992234354416, 3.793023760679264722 ) ) ;
#13150=CARTESIAN_POINT ( 'NONE',  ( -1.027846397803611866, 27.50319992234354771, -3.346150245485499219 ) ) ;
#13151=CARTESIAN_POINT ( 'NONE',  ( -1.593127413382952939, 21.62819992234354416, 2.091722143975172532 ) ) ;
#13153=CARTESIAN_POINT ( 'NONE',  ( 2.829195390882805583, 17.12180007765647716, 3.793023760679204770 ) ) ;
#13158=CARTESIAN_POINT ( 'NONE',  ( -3.518350579753630747, 33.12180007765646650, -1.080741659609802729 ) ) ;
#13161=CARTESIAN_POINT ( 'NONE',  ( 4.481649420246366589, 29.12180007765647005, -1.518615910253458212 ) ) ;
#13164=CARTESIAN_POINT ( 'NONE',  ( -3.518350579753630747, 33.12180007765646650, -1.080741659609802729 ) ) ;
#13169=CARTESIAN_POINT ( 'NONE',  ( 2.211161402132839626, 25.37819992234353705, -2.942372952327218183 ) ) ;
#13172=CARTESIAN_POINT ( 'NONE',  ( 0.7188294034286049072, 23.74680007765648426, -2.395093729190366005 ) ) ;
#13175=CARTESIAN_POINT ( 'NONE',  ( -2.864755990943222308, 36.75319992234354061, 2.011557305968548093 ) ) ;
#13189=CARTESIAN_POINT ( 'NONE',  ( 1.989345975306457071, 26.00319992234354771, 1.515154207786300500 ) ) ;
#13192=CARTESIAN_POINT ( 'NONE',  ( -3.481649420246369697, 20.37180007765647716, 1.193696214020542490 ) ) ;
#13208=CARTESIAN_POINT ( 'NONE',  ( -2.518350579753628526, 33.12180007765648071, -0.7558219633769075463 ) ) ;
#13210=CARTESIAN_POINT ( 'NONE',  ( -1.027846397803541700, 22.49680007765648071, 3.346150245485522312 ) ) ;
#13215=CARTESIAN_POINT ( 'NONE',  ( -3.500000000000000444, 19.50319992234354416, -0.05647727720529563400 ) ) ;
#13219=CARTESIAN_POINT ( 'NONE',  ( -1.135272562821090014, 18.49680007765648071, -3.311245368580554072 ) ) ;
#13240=CARTESIAN_POINT ( 'NONE',  ( 4.518350579753602325, 23.12819992234354416, -1.405661355842793725 ) ) ;
#13241=CARTESIAN_POINT ( 'NONE',  ( 1.135272562821020070, 37.75319992234354061, -3.311245368580577164 ) ) ;
#13242=CARTESIAN_POINT ( 'NONE',  ( -1.989345975306457071, 17.25319992234354416, -1.515154207786300944 ) ) ;
#13244=CARTESIAN_POINT ( 'NONE',  ( 2.829195390882724759, 37.87819992234353350, -3.793023760679264278 ) ) ;
#13250=CARTESIAN_POINT ( 'NONE',  ( 2.211161402132902243, 32.12180007765647360, 2.942372952327172442 ) ) ;
#13253=CARTESIAN_POINT ( 'NONE',  ( -1.336863392178478716, 27.49680007765647360, 4.297206761780677731 ) ) ;
#13264=CARTESIAN_POINT ( 'NONE',  ( -2.864755990943222308, 24.25319992234354416, 2.011557305968548093 ) ) ;
#13268=CARTESIAN_POINT ( 'NONE',  ( 1.989345975306426206, 18.99680007765647716, -1.515154207786343799 ) ) ;
#13269=CARTESIAN_POINT ( 'NONE',  ( -0.05938372350918959958, 16.37819992234354416, 4.731580009072201776 ) ) ;
#13290=CARTESIAN_POINT ( 'NONE',  ( 1.593127413382953383, 30.37819992234354061, -2.091722143975172532 ) ) ;
#13292=CARTESIAN_POINT ( 'NONE',  ( 2.211161402132902243, 24.62180007765647716, 2.942372952327172442 ) ) ;
#13309=CARTESIAN_POINT ( 'NONE',  ( -0.7188294034286043521, 27.49680007765648071, 2.395093729190366005 ) ) ;
#13311=CARTESIAN_POINT ( 'NONE',  ( -3.518350579753630303, 28.12180007765647716, -1.080741659609802952 ) ) ;
#13315=CARTESIAN_POINT ( 'NONE',  ( -2.115076519116425580, 19.87819992234354416, -3.012182706137062738 ) ) ;
#13319=CARTESIAN_POINT ( 'NONE',  ( -3.673772985318219053, 38.24680007765647360, -2.599342558260952174 ) ) ;
#13339=( LENGTH_UNIT ( ) NAMED_UNIT ( * ) SI_UNIT ( .MILLI., .METRE. ) );
#13340=CARTESIAN_POINT ( 'NONE',  ( -4.518350579753602325, 29.37819992234355126, 1.405661355842794391 ) ) ;
#13342=CARTESIAN_POINT ( 'NONE',  ( 1.989345975306457071, 21.00319992234354771, 1.515154207786300500 ) ) ;
#13344=CARTESIAN_POINT ( 'NONE',  ( 1.336863392178479160, 16.24680007765647716, -4.297206761780677731 ) ) ;
#13349=CARTESIAN_POINT ( 'NONE',  ( 3.481649420246369697, 34.12180007765648071, -1.193696214020541824 ) ) ;
#13360=CARTESIAN_POINT ( 'NONE',  ( -2.115076519116425580, 29.87819992234353350, -3.012182706137062738 ) ) ;
#13361=CARTESIAN_POINT ( 'NONE',  ( -1.027846397803611866, 15.00319992234354594, -3.346150245485499219 ) ) ;
#13363=CARTESIAN_POINT ( 'NONE',  ( 0.05938372350926800214, 24.87180007765647716, 2.628655560595669183 ) ) ;
#13364=CARTESIAN_POINT ( 'NONE',  ( -1.444289557195956863, 21.50319992234354771, 4.262301884875733471 ) ) ;
#13368=CARTESIAN_POINT ( 'NONE',  ( 4.481649420246366589, 39.12180007765647360, -1.518615910253458212 ) ) ;
#13381=CARTESIAN_POINT ( 'NONE',  ( -2.500000000000001332, 32.00319992234354061, -0.05647727720530596601 ) ) ;
#13383=CARTESIAN_POINT ( 'NONE',  ( 2.864755990943265829, 19.49680007765648071, 2.011557305968487697 ) ) ;
#13399=CARTESIAN_POINT ( 'NONE',  ( -0.8262555684461330152, 30.99680007765647716, -2.360188852285403982 ) ) ;
#13401=CARTESIAN_POINT ( 'NONE',  ( -3.481649420246370141, 30.37180007765647716, 1.193696214020542268 ) ) ;
#13410=CARTESIAN_POINT ( 'NONE',  ( -0.05938372350928957516, 38.62180007765647360, -4.731580009072201776 ) ) ;
#13429=CARTESIAN_POINT ( 'NONE',  ( -1.444289557195956863, 29.00319992234354771, 4.262301884875733471 ) ) ;
#13430=CARTESIAN_POINT ( 'NONE',  ( 1.027846397803612311, 38.75319992234354061, 3.346150245485499219 ) ) ;
#13431=CARTESIAN_POINT ( 'NONE',  ( -1.497042530366522461, 17.37819992234354416, -2.161531897785030409 ) ) ;
#13434=CARTESIAN_POINT ( 'NONE',  ( -1.444289557196047014, 20.99680007765647360, -4.262301884875704161 ) ) ;
#13438=CARTESIAN_POINT ( 'NONE',  ( 1.135272562821090458, 34.74680007765648071, 3.311245368580554072 ) ) ;
#13449=CARTESIAN_POINT ( 'NONE',  ( -0.05938372350920063936, 23.87819992234354416, 3.680117784833935701 ) ) ;
#13454=CARTESIAN_POINT ( 'NONE',  ( -1.593127413382998459, 23.37180007765648071, -2.091722143975139669 ) ) ;
#13455=CARTESIAN_POINT ( 'NONE',  ( 4.518350579753602325, 20.62819992234354416, -1.405661355842793725 ) ) ;
#13461=CARTESIAN_POINT ( 'NONE',  ( -4.518350579753632523, 38.12180007765647360, -1.405661355842698468 ) ) ;
#13471=CARTESIAN_POINT ( 'NONE',  ( -0.7188294034286550893, 30.00319992234354416, -2.395093729190349130 ) ) ;
#13473=CARTESIAN_POINT ( 'NONE',  ( 0.05938372350927906274, 22.37180007765648071, 3.680117784833935701 ) ) ;
#13485=CARTESIAN_POINT ( 'NONE',  ( -1.497042530366477164, 32.62180007765647360, 2.161531897785062384 ) ) ;
#13487=CARTESIAN_POINT ( 'NONE',  ( -2.211161402132901799, 28.37180007765647716, -2.942372952327172886 ) ) ;
#13493=CARTESIAN_POINT ( 'NONE',  ( 4.499999999999999112, 39.24680007765647360, -0.05647727720537982360 ) ) ;
#13507=CARTESIAN_POINT ( 'NONE',  ( 3.481649420246369697, 34.12180007765648071, -1.193696214020541824 ) ) ;
#13513=CARTESIAN_POINT ( 'NONE',  ( -4.481649420246396787, 32.12819992234354771, -1.518615910253363399 ) ) ;
#13514=CARTESIAN_POINT ( 'NONE',  ( -1.135272562821019626, 39.00319992234354061, 3.311245368580577164 ) ) ;
#13516=CARTESIAN_POINT ( 'NONE',  ( -2.518350579753611207, 24.37819992234354416, 0.7558219633769609480 ) ) ;
#13519=CARTESIAN_POINT ( 'NONE',  ( -3.673772985318219053, 15.74680007765647716, -2.599342558260952174 ) ) ;
#13523=CARTESIAN_POINT ( 'NONE',  ( -0.05938372350927861171, 36.12180007765648782, -3.680117784833935701 ) ) ;
#13532=CARTESIAN_POINT ( 'NONE',  ( 2.864755990943265829, 16.99680007765647716, 2.011557305968487697 ) ) ;
#13535=CARTESIAN_POINT ( 'NONE',  ( 2.115076519116426024, 38.62819992234354771, 3.012182706137062294 ) ) ;
#13538=CARTESIAN_POINT ( 'NONE',  ( -1.989345975306426206, 22.74680007765647716, 1.515154207786343799 ) ) ;
#13540=CARTESIAN_POINT ( 'NONE',  ( -4.518350579753602325, 16.87819992234354416, 1.405661355842794391 ) ) ;
#13545=CARTESIAN_POINT ( 'NONE',  ( 2.829195390882805583, 39.62180007765647360, 3.793023760679204770 ) ) ;
#13552=CARTESIAN_POINT ( 'NONE',  ( 2.798362969681366330, 18.99680007765648071, -2.102939460078824929 ) ) ;
#13556=CARTESIAN_POINT ( 'NONE',  ( 0.8262555684460829442, 27.75319992234355126, -2.360188852285421302 ) ) ;
#13557=DIRECTION ( 'NONE',  ( 0.000000000000000000, 0.000000000000000000, 1.000000000000000000 ) ) ;
#13559=CARTESIAN_POINT ( 'NONE',  ( 2.864755990943265829, 26.99680007765648071, 2.011557305968487697 ) ) ;
#13567=CARTESIAN_POINT ( 'NONE',  ( 4.499999999999999112, 19.24680007765647716, -0.05647727720537982360 ) ) ;
#13573=CARTESIAN_POINT ( 'NONE',  ( 2.500000000000001332, 26.74680007765648071, -0.05647727720535888202 ) ) ;
#13578=CARTESIAN_POINT ( 'NONE',  ( 1.027846397803542144, 33.74680007765648071, -3.346150245485522312 ) ) ;
#13586=CARTESIAN_POINT ( 'NONE',  ( -2.115076519116362519, 25.12180007765647360, 3.012182706137107147 ) ) ;
#13601=CARTESIAN_POINT ( 'NONE',  ( 2.864755990943265829, 29.49680007765647716, 2.011557305968487697 ) ) ;
#13606=CARTESIAN_POINT ( 'NONE',  ( -3.607379964056363075, 32.25319992234354061, -2.690724712371229899 ) ) ;
#13607=CARTESIAN_POINT ( 'NONE',  ( -2.798362969681409851, 34.75319992234354771, -2.102939460078765421 ) ) ;
#13608=CARTESIAN_POINT ( 'NONE',  ( -0.7188294034286550893, 25.00319992234354771, -2.395093729190349130 ) ) ;
#13610=CARTESIAN_POINT ( 'NONE',  ( -0.05938372350928957516, 28.62180007765647005, -4.731580009072201776 ) ) ;
#13616=CARTESIAN_POINT ( 'NONE',  ( 1.027846397803542144, 36.24680007765648071, -3.346150245485522312 ) ) ;
#13629=CARTESIAN_POINT ( 'NONE',  ( -2.798362969681409851, 32.25319992234354771, -2.102939460078765421 ) ) ;
#13630=CARTESIAN_POINT ( 'NONE',  ( 2.211161402132839182, 15.37819992234354594, -2.942372952327217739 ) ) ;
#13632=CARTESIAN_POINT ( 'NONE',  ( -1.593127413382998459, 30.87180007765647716, -2.091722143975139669 ) ) ;
#13634=CARTESIAN_POINT ( 'NONE',  ( 3.673772985318163098, 28.00319992234354771, -2.599342558261029001 ) ) ;
#13639=CARTESIAN_POINT ( 'NONE',  ( -4.499999999999999112, 40.49680007765648071, 0.05647727720537927543 ) ) ;
#13650=CARTESIAN_POINT ( 'NONE',  ( -2.518350579753611207, 39.37819992234354771, 0.7558219633769609480 ) ) ;
#13652=CARTESIAN_POINT ( 'NONE',  ( 2.211161402132902243, 29.62180007765648071, 2.942372952327172442 ) ) ;
#13653=CARTESIAN_POINT ( 'NONE',  ( 1.027846397803612311, 16.25319992234354416, 3.346150245485499219 ) ) ;
#13660=CARTESIAN_POINT ( 'NONE',  ( 4.518350579753633411, 26.87180007765647716, 1.405661355842698468 ) ) ;
#13667=CARTESIAN_POINT ( 'NONE',  ( -2.055738996568313048, 38.24680007765647360, -1.423772053676023441 ) ) ;
#13669=CARTESIAN_POINT ( 'NONE',  ( -1.027846397803541700, 27.49680007765648071, 3.346150245485522312 ) ) ;
#13671=CARTESIAN_POINT ( 'NONE',  ( -4.000000000000002665, 15.00000000000001066, -0.2096920304738193463 ) ) ;
#13677=CARTESIAN_POINT ( 'NONE',  ( 3.481649420246369697, 24.12180007765648071, -1.193696214020541824 ) ) ;
#13695=CARTESIAN_POINT ( 'NONE',  ( -3.518350579753630747, 35.62180007765648782, -1.080741659609802729 ) ) ;
#13701=CARTESIAN_POINT ( 'NONE',  ( -4.518350579753602325, 36.87819992234354061, 1.405661355842794391 ) ) ;
#13703=CARTESIAN_POINT ( 'NONE',  ( 2.481649420246391902, 30.87819992234354416, 0.8687765177875720335 ) ) ;
#13705=CARTESIAN_POINT ( 'NONE',  ( 3.673772985318219053, 29.49680007765647360, 2.599342558260951730 ) ) ;
#13711=CARTESIAN_POINT ( 'NONE',  ( 2.211161402132902243, 39.62180007765646650, 2.942372952327172442 ) ) ;
#13718=CARTESIAN_POINT ( 'NONE',  ( 3.500000000000000444, 16.74680007765647716, -0.05647727720536935281 ) ) ;
#13722=CARTESIAN_POINT ( 'NONE',  ( 3.500000000000000444, 35.75319992234354771, 0.05647727720529520379 ) ) ;
#13723=CARTESIAN_POINT ( 'NONE',  ( -3.518350579753606322, 19.37819992234354416, 1.080741659609877781 ) ) ;
#13725=CARTESIAN_POINT ( 'NONE',  ( -0.05938372350926768989, 33.62180007765647360, -2.628655560595669183 ) ) ;
#13727=CARTESIAN_POINT ( 'NONE',  ( -4.499999999999999112, 24.50319992234354771, -0.05647727720528529505 ) ) ;
#13732=CARTESIAN_POINT ( 'NONE',  ( 3.518350579753631191, 16.87180007765648071, 1.080741659609802285 ) ) ;
#13748=CARTESIAN_POINT ( 'NONE',  ( 1.989345975306457071, 38.50319992234354771, 1.515154207786300500 ) ) ;
#13751=CARTESIAN_POINT ( 'NONE',  ( -1.027846397803541700, 32.49680007765648071, 3.346150245485522312 ) ) ;
#13753=CARTESIAN_POINT ( 'NONE',  ( 2.115076519116426024, 28.62819992234353705, 3.012182706137062294 ) ) ;
#13758=CARTESIAN_POINT ( 'NONE',  ( 2.829195390882805583, 22.12180007765647716, 3.793023760679204770 ) ) ;
#13764=CARTESIAN_POINT ( 'NONE',  ( -2.500000000000001332, 40.49680007765648071, 0.05647727720535858364 ) ) ;
#13766=CARTESIAN_POINT ( 'NONE',  ( -1.135272562821090014, 38.49680007765647360, -3.311245368580554072 ) ) ;
#13773=CARTESIAN_POINT ( 'NONE',  ( 0.05938372350927906274, 27.37180007765647716, 3.680117784833935701 ) ) ;
#13785=CARTESIAN_POINT ( 'NONE',  ( -3.481649420246369697, 40.37180007765648071, 1.193696214020542490 ) ) ;
#13790=CARTESIAN_POINT ( 'NONE',  ( 3.673772985318163098, 38.00319992234354061, -2.599342558261029001 ) ) ;
#13793=CARTESIAN_POINT ( 'NONE',  ( -1.989345975306457071, 24.75319992234354416, -1.515154207786300944 ) ) ;
#13798=CARTESIAN_POINT ( 'NONE',  ( -3.607379964056306676, 22.74680007765647716, 2.690724712371306282 ) ) ;
#13810=AXIS2_PLACEMENT_3D ( 'NONE', #2928, #11347, #13960 ) ;
#13815=CARTESIAN_POINT ( 'NONE',  ( -2.211161402132839182, 31.62819992234354416, 2.942372952327218627 ) ) ;
#13816=CARTESIAN_POINT ( 'NONE',  ( -0.05938372350920064630, 23.87819992234354416, 3.680117784833935701 ) ) ;
#13819=CARTESIAN_POINT ( 'NONE',  ( 0.05938372350926800214, 29.87180007765648426, 2.628655560595669183 ) ) ;
#13820=CARTESIAN_POINT ( 'NONE',  ( 0.05938372350919016857, 22.62819992234354416, -4.731580009072201776 ) ) ;
#13826=CARTESIAN_POINT ( 'NONE',  ( -2.864755990943265829, 25.74680007765647716, -2.011557305968488141 ) ) ;
#13838=CARTESIAN_POINT ( 'NONE',  ( -0.05938372350921170689, 36.37819992234354771, 2.628655560595669183 ) ) ;
#13840=CARTESIAN_POINT ( 'NONE',  ( 1.027846397803542144, 33.74680007765648071, -3.346150245485522312 ) ) ;
#13841=CARTESIAN_POINT ( 'NONE',  ( -3.500000000000000444, 24.50319992234354416, -0.05647727720529563400 ) ) ;
#13854=DIRECTION ( 'NONE',  ( -1.028113302204112171E-14, 0.1129545544106649313, -0.9936001553129349961 ) ) ;
#13859=CARTESIAN_POINT ( 'NONE',  ( 0.05938372350926800214, 39.87180007765647360, 2.628655560595669183 ) ) ;
#13861=CARTESIAN_POINT ( 'NONE',  ( 3.500000000000000444, 34.24680007765648071, -0.05647727720536935281 ) ) ;
#13864=CARTESIAN_POINT ( 'NONE',  ( -1.296796814808491183, 15.00000000000144240, -3.409573799784564763 ) ) ;
#13869=CARTESIAN_POINT ( 'NONE',  ( 1.027846397803542144, 21.24680007765647716, -3.346150245485522312 ) ) ;
#13881=CARTESIAN_POINT ( 'NONE',  ( -2.115076519116362519, 37.62180007765648071, 3.012182706137107147 ) ) ;
#13886=CARTESIAN_POINT ( 'NONE',  ( -3.673772985318163098, 31.75319992234354771, 2.599342558261029001 ) ) ;
#13888=CARTESIAN_POINT ( 'NONE',  ( -2.518350579753611207, 29.37819992234355126, 0.7558219633769609480 ) ) ;
#13891=CARTESIAN_POINT ( 'NONE',  ( -3.607379964056306676, 27.74680007765648071, 2.690724712371306282 ) ) ;
#13908=CARTESIAN_POINT ( 'NONE',  ( -1.135272562821090014, 15.99680007765647716, -3.311245368580554072 ) ) ;
#13910=CARTESIAN_POINT ( 'NONE',  ( -3.518350579753605434, 31.87819992234354416, 1.080741659609877781 ) ) ;
#13911=CARTESIAN_POINT ( 'NONE',  ( -2.798362969681409851, 17.25319992234354416, -2.102939460078765421 ) ) ;
#13913=CARTESIAN_POINT ( 'NONE',  ( -1.989345975306426206, 27.74680007765648071, 1.515154207786343799 ) ) ;
#13914=CARTESIAN_POINT ( 'NONE',  ( -3.673772985318163098, 29.25319992234354416, 2.599342558261029001 ) ) ;
#13920=CARTESIAN_POINT ( 'NONE',  ( 1.135272562821090458, 19.74680007765648071, 3.311245368580554072 ) ) ;
#13930=CARTESIAN_POINT ( 'NONE',  ( -2.864755990943265829, 15.74680007765647716, -2.011557305968488141 ) ) ;
#13935=CARTESIAN_POINT ( 'NONE',  ( 0.05938372350921204690, 32.62819992234354771, -2.628655560595669183 ) ) ;
#13937=CARTESIAN_POINT ( 'NONE',  ( -1.027846397803541700, 27.49680007765648071, 3.346150245485522312 ) ) ;
#13938=CARTESIAN_POINT ( 'NONE',  ( -1.027846397803611866, 30.00319992234354416, -3.346150245485499219 ) ) ;
#13948=CARTESIAN_POINT ( 'NONE',  ( 0.05938372350921204690, 15.12819992234354771, -2.628655560595669183 ) ) ;
#13950=CARTESIAN_POINT ( 'NONE',  ( 0.05938372350927906967, 39.87180007765648071, 3.680117784833935701 ) ) ;
#13957=CARTESIAN_POINT ( 'NONE',  ( 2.798362969681366330, 31.49680007765647716, -2.102939460078824929 ) ) ;
#13960=DIRECTION ( 'NONE',  ( 0.000000000000000000, -0.000000000000000000, 1.000000000000000000 ) ) ;
#13967=CARTESIAN_POINT ( 'NONE',  ( -3.481649420246369697, 37.87180007765648071, 1.193696214020542490 ) ) ;
#13974=CARTESIAN_POINT ( 'NONE',  ( -4.499999999999999112, 15.49680007765647538, 0.05647727720537927543 ) ) ;
#13977=CARTESIAN_POINT ( 'NONE',  ( -1.497042530366522461, 34.87819992234354771, -2.161531897785030409 ) ) ;
#13980=CARTESIAN_POINT ( 'NONE',  ( 4.518350579753633411, 21.87180007765647360, 1.405661355842698468 ) ) ;
#13982=B_SPLINE_CURVE_WITH_KNOTS ( 'NONE', 3,
 ( #18064, #13671, #16666, #6635, #15271, #15362, #12281, #16848, #5336, #17970, #5239, #2480, #10896, #3945, #9595, #2570, #11074, #13864, #1171, #18155, #2660, #1265, #8294, #6900 ),
 .UNSPECIFIED., .F., .F.,
 ( 4, 2, 2, 2, 2, 2, 2, 2, 2, 2, 2, 4 ),
 ( 0.000000000000000000, 0.0006232196737604741134, 0.001246439347520948227, 0.001869659021281422882, 0.002492878695041897321, 0.003116098368802372193, 0.003739318042562846632, 0.004362537716323321504, 0.004674147553203558507, 0.004829952471643678309, 0.004907854930863738210, 0.004985757390083797244 ),
 .UNSPECIFIED. ) ;
#13995=CARTESIAN_POINT ( 'NONE',  ( 4.499999999999999112, 15.75319992234354416, 0.05647727720528474687 ) ) ;
#13996=CARTESIAN_POINT ( 'NONE',  ( -2.798362969681409851, 22.25319992234354416, -2.102939460078765421 ) ) ;
#13998=CARTESIAN_POINT ( 'NONE',  ( -2.518350579753628526, 28.12180007765647716, -0.7558219633769075463 ) ) ;
#14000=CARTESIAN_POINT ( 'NONE',  ( 3.673772985318163098, 25.50319992234354416, -2.599342558261029001 ) ) ;
#14002=UNCERTAINTY_MEASURE_WITH_UNIT (LENGTH_MEASURE( 1.000000000000000082E-05 ), #2985, 'distance_accuracy_value', 'NONE');
#14006=CARTESIAN_POINT ( 'NONE',  ( 2.864755990943265829, 21.99680007765647716, 2.011557305968487697 ) ) ;
#14017=CARTESIAN_POINT ( 'NONE',  ( 1.027846397803542144, 26.24680007765648071, -3.346150245485522312 ) ) ;
#14022=CARTESIAN_POINT ( 'NONE',  ( -0.7188294034286550893, 37.50319992234354771, -2.395093729190349130 ) ) ;
#14024=CARTESIAN_POINT ( 'NONE',  ( 3.481649420246369697, 31.62180007765647360, -1.193696214020541824 ) ) ;
#14026=CARTESIAN_POINT ( 'NONE',  ( 2.115076519116426024, 26.12819992234354771, 3.012182706137062294 ) ) ;
#14038=CARTESIAN_POINT ( 'NONE',  ( 0.8262555684460829442, 15.25319992234354771, -2.360188852285421302 ) ) ;
#14046=CARTESIAN_POINT ( 'NONE',  ( -3.500000000000000444, 30.49680007765647716, 0.05647727720536892260 ) ) ;
#14056=CARTESIAN_POINT ( 'NONE',  ( -0.05938372350927861171, 36.12180007765648782, -3.680117784833935701 ) ) ;
#14059=CARTESIAN_POINT ( 'NONE',  ( -0.05938372350918959958, 38.87819992234354771, 4.731580009072201776 ) ) ;
#14061=CARTESIAN_POINT ( 'NONE',  ( 2.481649420246391902, 35.87819992234354771, 0.8687765177875720335 ) ) ;
#14064=CARTESIAN_POINT ( 'NONE',  ( 2.829195390882805583, 37.12180007765647360, 3.793023760679204770 ) ) ;
#14074=EDGE_LOOP ( 'NONE', ( #12404, #14378, #12320 ) ) ;
#14084=CARTESIAN_POINT ( 'NONE',  ( -2.829195390882724315, 21.62819992234354416, 3.793023760679264722 ) ) ;
#14085=CARTESIAN_POINT ( 'NONE',  ( -1.027846397803611866, 17.50319992234354416, -3.346150245485499219 ) ) ;
#14088=CARTESIAN_POINT ( 'NONE',  ( 0.05938372350926800214, 34.87180007765648071, 2.628655560595669183 ) ) ;
#14089=CARTESIAN_POINT ( 'NONE',  ( -0.05938372350918959958, 33.87819992234354061, 4.731580009072201776 ) ) ;
#14094=CARTESIAN_POINT ( 'NONE',  ( 3.518350579753631191, 19.37180007765648071, 1.080741659609802285 ) ) ;
#14100=CARTESIAN_POINT ( 'NONE',  ( -1.336863392178478716, 24.99680007765647716, 4.297206761780677731 ) ) ;
#14106=CARTESIAN_POINT ( 'NONE',  ( -3.518350579753630747, 23.12180007765647716, -1.080741659609802729 ) ) ;
#14112=CARTESIAN_POINT ( 'NONE',  ( 1.135272562821020070, 22.75319992234354416, -3.311245368580577164 ) ) ;
#14114=CARTESIAN_POINT ( 'NONE',  ( -3.481649420246369697, 40.37180007765648071, 1.193696214020542490 ) ) ;
#14115=CARTESIAN_POINT ( 'NONE',  ( -2.115076519116425580, 27.37819992234354771, -3.012182706137062738 ) ) ;
#14128=CARTESIAN_POINT ( 'NONE',  ( 2.055738996568281518, 18.00319992234354416, -1.423772053676066518 ) ) ;
#14130=CARTESIAN_POINT ( 'NONE',  ( -2.115076519116362519, 35.12180007765646650, 3.012182706137108035 ) ) ;
#14135=CARTESIAN_POINT ( 'NONE',  ( 1.027846397803542144, 28.74680007765647716, -3.346150245485522312 ) ) ;
#14149=CARTESIAN_POINT ( 'NONE',  ( -2.500000000000001332, 17.99680007765648071, 0.05647727720535858364 ) ) ;
#14156=CARTESIAN_POINT ( 'NONE',  ( 2.481649420246391902, 33.37819992234354771, 0.8687765177875720335 ) ) ;
#14159=CARTESIAN_POINT ( 'NONE',  ( -3.607379964056306676, 30.24680007765647360, 2.690724712371306282 ) ) ;
#14177=CARTESIAN_POINT ( 'NONE',  ( -2.733110507866328476, 17.37819992234354416, -3.862833514489096398 ) ) ;
#14178=CARTESIAN_POINT ( 'NONE',  ( 2.115076519116425580, 26.12819992234354771, 3.012182706137062294 ) ) ;
#14180=CARTESIAN_POINT ( 'NONE',  ( -2.481649420246374138, 37.87180007765647360, 0.8687765177876256573 ) ) ;
#14183=CARTESIAN_POINT ( 'NONE',  ( -2.733110507866328476, 34.87819992234354771, -3.862833514489096398 ) ) ;
#14189=CARTESIAN_POINT ( 'NONE',  ( -2.115076519116362519, 25.12180007765647360, 3.012182706137107147 ) ) ;
#14193=CARTESIAN_POINT ( 'NONE',  ( -3.673772985318219053, 23.24680007765647716, -2.599342558260952174 ) ) ;
#14198=CARTESIAN_POINT ( 'NONE',  ( -2.211161402132902243, 25.87180007765647360, -2.942372952327172886 ) ) ;
#14204=CARTESIAN_POINT ( 'NONE',  ( 2.798362969681409851, 16.00319992234354416, 2.102939460078764977 ) ) ;
#14206=CARTESIAN_POINT ( 'NONE',  ( 0.05938372350926800214, 17.37180007765647716, 2.628655560595669183 ) ) ;
#14209=CARTESIAN_POINT ( 'NONE',  ( -2.115076519116425580, 34.87819992234354771, -3.012182706137062738 ) ) ;
#14221=CARTESIAN_POINT ( 'NONE',  ( -2.987022202050954700, 15.00000000000010125, -0.3375100304031865561 ) ) ;
#14225=CARTESIAN_POINT ( 'NONE',  ( -0.7188294034286550893, 22.50319992234354771, -2.395093729190349130 ) ) ;
#14227=CARTESIAN_POINT ( 'NONE',  ( 1.027846397803542144, 18.74680007765648071, -3.346150245485522312 ) ) ;
#14233=CARTESIAN_POINT ( 'NONE',  ( -1.135272562821090014, 35.99680007765648071, -3.311245368580554072 ) ) ;
#14244=CARTESIAN_POINT ( 'NONE',  ( 2.518350579753628971, 19.37180007765648071, 0.7558219633769073242 ) ) ;
#14246=CARTESIAN_POINT ( 'NONE',  ( 1.027846397803542144, 21.24680007765647716, -3.346150245485522312 ) ) ;
#14250=CARTESIAN_POINT ( 'NONE',  ( -2.481649420246391902, 32.12819992234354771, -0.8687765177875723666 ) ) ;
#14254=CARTESIAN_POINT ( 'NONE',  ( -0.05938372350928957516, 33.62180007765647360, -4.731580009072201776 ) ) ;
#14271=CARTESIAN_POINT ( 'NONE',  ( 0.05938372350919016857, 17.62819992234354416, -4.731580009072201776 ) ) ;
#14272=CARTESIAN_POINT ( 'NONE',  ( 2.115076519116425580, 28.62819992234354061, 3.012182706137062294 ) ) ;
#14273=CARTESIAN_POINT ( 'NONE',  ( 0.7188294034286049072, 36.24680007765647360, -2.395093729190366005 ) ) ;
#14276=CARTESIAN_POINT ( 'NONE',  ( -4.499999999999999112, 34.50319992234354771, -0.05647727720528529505 ) ) ;
#14282=CARTESIAN_POINT ( 'NONE',  ( 3.481649420246369697, 29.12180007765647005, -1.193696214020541824 ) ) ;
#14286=CARTESIAN_POINT ( 'NONE',  ( 3.673772985318219053, 34.49680007765647360, 2.599342558260951730 ) ) ;
#14290=CARTESIAN_POINT ( 'NONE',  ( -2.115076519116362519, 22.62180007765647360, 3.012182706137107147 ) ) ;
#14297=CARTESIAN_POINT ( 'NONE',  ( -2.864755990943222308, 19.25319992234354416, 2.011557305968548093 ) ) ;
#14299=CARTESIAN_POINT ( 'NONE',  ( 3.500000000000000444, 39.24680007765647360, -0.05647727720536935281 ) ) ;
#14301=CARTESIAN_POINT ( 'NONE',  ( 1.027846397803612311, 38.75319992234354061, 3.346150245485499219 ) ) ;
#14305=MANIFOLD_SOLID_BREP ( 'Cavity1', #539 ) ;
#14318=CARTESIAN_POINT ( 'NONE',  ( -1.989345975306457071, 17.25319992234354416, -1.515154207786300944 ) ) ;
#14320=CARTESIAN_POINT ( 'NONE',  ( -1.135272562821090014, 15.99680007765647716, -3.311245368580554072 ) ) ;
#14326=CARTESIAN_POINT ( 'NONE',  ( -3.518350579753630747, 35.62180007765648782, -1.080741659609802729 ) ) ;
#14337=CARTESIAN_POINT ( 'NONE',  ( 2.500000000000001332, 21.74680007765648071, -0.05647727720535888202 ) ) ;
#14339=CARTESIAN_POINT ( 'NONE',  ( 2.798362969681366330, 18.99680007765648071, -2.102939460078824929 ) ) ;
#14343=CARTESIAN_POINT ( 'NONE',  ( 2.500000000000001332, 38.25319992234354771, 0.05647727720530566764 ) ) ;
#14346=CARTESIAN_POINT ( 'NONE',  ( -1.444289557196047014, 33.49680007765648071, -4.262301884875704161 ) ) ;
#14364=CARTESIAN_POINT ( 'NONE',  ( -3.518350579753605434, 39.37819992234354771, 1.080741659609877781 ) ) ;
#14365=CARTESIAN_POINT ( 'NONE',  ( -1.027846397803611866, 25.00319992234354416, -3.346150245485499219 ) ) ;
#14366=CARTESIAN_POINT ( 'NONE',  ( -2.055738996568313048, 35.74680007765648071, -1.423772053676023441 ) ) ;
#14368=CARTESIAN_POINT ( 'NONE',  ( 1.336863392178569754, 31.25319992234354416, 4.297206761780648421 ) ) ;
#14372=CARTESIAN_POINT ( 'NONE',  ( -2.864755990943265829, 33.24680007765648071, -2.011557305968488141 ) ) ;
#14375=CARTESIAN_POINT ( 'NONE',  ( 2.733110507866247652, 28.87180007765647716, -3.862833514489153686 ) ) ;
#14378=ORIENTED_EDGE ( 'NONE', *, *, #5322, .T. ) ;
#14380=CARTESIAN_POINT ( 'NONE',  ( -1.027846397803541700, 19.99680007765648071, 3.346150245485522312 ) ) ;
#14385=CARTESIAN_POINT ( 'NONE',  ( -3.481649420246394122, 17.12819992234354061, -1.193696214020467883 ) ) ;
#14388=CARTESIAN_POINT ( 'NONE',  ( 3.518350579753631191, 39.37180007765646650, 1.080741659609802285 ) ) ;
#14389=CARTESIAN_POINT ( 'NONE',  ( -1.135272562821019626, 34.00319992234354771, 3.311245368580577164 ) ) ;
#14401=CARTESIAN_POINT ( 'NONE',  ( -1.514047762142602060, 14.99999999999999645, -2.869914431049744863 ) ) ;
#14404=CARTESIAN_POINT ( 'NONE',  ( 2.518350579753611207, 23.12819992234354416, -0.7558219633769606149 ) ) ;
#14408=CARTESIAN_POINT ( 'NONE',  ( -3.673772985318163098, 39.25319992234354771, 2.599342558261029001 ) ) ;
#14414=CARTESIAN_POINT ( 'NONE',  ( -2.798362969681365886, 37.74680007765647360, 2.102939460078824929 ) ) ;
#14428=CARTESIAN_POINT ( 'NONE',  ( -2.500000000000001332, 25.49680007765647716, 0.05647727720535858364 ) ) ;
#14430=CARTESIAN_POINT ( 'NONE',  ( -0.05938372350927861865, 21.12180007765647716, -3.680117784833935701 ) ) ;
#14437=CARTESIAN_POINT ( 'NONE',  ( -3.518350579753605434, 16.87819992234353705, 1.080741659609877781 ) ) ;
#14441=CARTESIAN_POINT ( 'NONE',  ( 3.607379964056306676, 33.99680007765647360, -2.690724712371305838 ) ) ;
#14462=CARTESIAN_POINT ( 'NONE',  ( -3.607379964056363075, 29.75319992234354416, -2.690724712371229899 ) ) ;
#14464=CARTESIAN_POINT ( 'NONE',  ( -1.135272562821019626, 26.50319992234354771, 3.311245368580577164 ) ) ;
#14465=CARTESIAN_POINT ( 'NONE',  ( 0.7188294034286049072, 38.74680007765646650, -2.395093729190366005 ) ) ;
#14470=CARTESIAN_POINT ( 'NONE',  ( -3.673772985318163098, 36.75319992234353350, 2.599342558261029001 ) ) ;
#14475=CARTESIAN_POINT ( 'NONE',  ( -1.027846397803541700, 27.49680007765648071, 3.346150245485522312 ) ) ;
#14478=CARTESIAN_POINT ( 'NONE',  ( -3.673772985318219053, 30.74680007765647716, -2.599342558260952174 ) ) ;
#14484=CARTESIAN_POINT ( 'NONE',  ( 2.211161402132902243, 29.62180007765648071, 2.942372952327172442 ) ) ;
#14489=CARTESIAN_POINT ( 'NONE',  ( 3.500000000000000444, 18.25319992234354771, 0.05647727720529520379 ) ) ;
#14492=CARTESIAN_POINT ( 'NONE',  ( 2.798362969681366330, 36.49680007765648071, -2.102939460078824929 ) ) ;
#14494=CARTESIAN_POINT ( 'NONE',  ( -2.115076519116425580, 37.37819992234352640, -3.012182706137062738 ) ) ;
#14510=CARTESIAN_POINT ( 'NONE',  ( 1.593127413382953383, 17.87819992234354416, -2.091722143975172532 ) ) ;
#14516=CARTESIAN_POINT ( 'NONE',  ( -3.500000000000000444, 40.49680007765648071, 0.05647727720536892260 ) ) ;
#14529=CARTESIAN_POINT ( 'NONE',  ( -0.05938372350926768989, 23.62180007765648071, -2.628655560595669183 ) ) ;
#14531=CARTESIAN_POINT ( 'NONE',  ( -2.798362969681365886, 22.74680007765648071, 2.102939460078824929 ) ) ;
#14536=DIRECTION ( 'NONE',  ( 0.000000000000000000, 0.9936001553129349961, 0.1129545544106631688 ) ) ;
#14537=CARTESIAN_POINT ( 'NONE',  ( -2.211161402132839182, 21.62819992234354771, 2.942372952327218627 ) ) ;
#14540=CARTESIAN_POINT ( 'NONE',  ( -3.500000000000000444, 17.99680007765647716, 0.05647727720536892260 ) ) ;
#14555=ADVANCED_FACE ( 'NONE', ( #18035 ), #11090, .T. ) ;
#14560=CARTESIAN_POINT ( 'NONE',  ( 1.336863392178569754, 26.25319992234354416, 4.297206761780648421 ) ) ;
#14561=CARTESIAN_POINT ( 'NONE',  ( -3.481649420246394566, 27.12819992234354771, -1.193696214020467883 ) ) ;
#14562=CARTESIAN_POINT ( 'NONE',  ( 1.497042530366522461, 23.62819992234354416, 2.161531897785029965 ) ) ;
#14565=CARTESIAN_POINT ( 'NONE',  ( 1.336863392178569754, 38.75319992234354061, 4.297206761780648421 ) ) ;
#14569=CARTESIAN_POINT ( 'NONE',  ( 2.115076519116362963, 28.87180007765647716, -3.012182706137107147 ) ) ;
#14572=CARTESIAN_POINT ( 'NONE',  ( -2.829195390882805139, 30.87180007765647716, -3.793023760679206102 ) ) ;
#14575=CARTESIAN_POINT ( 'NONE',  ( -1.135272562821090014, 33.49680007765648071, -3.311245368580554072 ) ) ;
#14581=CARTESIAN_POINT ( 'NONE',  ( -2.798362969681409851, 27.25319992234354771, -2.102939460078765421 ) ) ;
#14584=CARTESIAN_POINT ( 'NONE',  ( -2.500000000000001332, 20.49680007765648071, 0.05647727720535858364 ) ) ;
#14587=CARTESIAN_POINT ( 'NONE',  ( 2.864755990943222308, 35.50319992234354771, -2.011557305968548093 ) ) ;
#14605=CARTESIAN_POINT ( 'NONE',  ( 1.593127413382953383, 27.87819992234355126, -2.091722143975172532 ) ) ;
#14607=CARTESIAN_POINT ( 'NONE',  ( -3.481649420246369697, 17.87180007765648071, 1.193696214020542490 ) ) ;
#14613=CARTESIAN_POINT ( 'NONE',  ( 2.798362969681366330, 38.99680007765647360, -2.102939460078824929 ) ) ;
#14616=CARTESIAN_POINT ( 'NONE',  ( -3.500000000000000444, 39.50319992234354771, -0.05647727720529563400 ) ) ;
#14626=CARTESIAN_POINT ( 'NONE',  ( 2.481649420246374138, 21.62180007765648426, -0.8687765177876252132 ) ) ;
#14629=CARTESIAN_POINT ( 'NONE',  ( 1.135272562821090458, 24.74680007765647716, 3.311245368580554072 ) ) ;
#14633=CARTESIAN_POINT ( 'NONE',  ( -3.481649420246394122, 17.12819992234354061, -1.193696214020467883 ) ) ;
#14636=CARTESIAN_POINT ( 'NONE',  ( -2.798362969681365886, 20.24680007765647716, 2.102939460078824929 ) ) ;
#14656=CARTESIAN_POINT ( 'NONE',  ( -3.673772985318163098, 29.25319992234354416, 2.599342558261029001 ) ) ;
#14657=CARTESIAN_POINT ( 'NONE',  ( -2.211161402132838738, 36.62819992234354061, 2.942372952327218183 ) ) ;
#14658=CARTESIAN_POINT ( 'NONE',  ( 0.05938372350921204690, 17.62819992234354416, -2.628655560595669183 ) ) ;
#14661=CARTESIAN_POINT ( 'NONE',  ( 0.05938372350929014415, 17.37180007765647716, 4.731580009072201776 ) ) ;
#14667=CARTESIAN_POINT ( 'NONE',  ( 1.135272562821090458, 27.24680007765648071, 3.311245368580554072 ) ) ;
#14671=CARTESIAN_POINT ( 'NONE',  ( -1.444289557196047014, 33.49680007765648071, -4.262301884875704161 ) ) ;
#14675=CARTESIAN_POINT ( 'NONE',  ( -2.864755990943265829, 30.74680007765647716, -2.011557305968488141 ) ) ;
#14681=CARTESIAN_POINT ( 'NONE',  ( -2.211161402132839182, 29.12819992234354771, 2.942372952327218627 ) ) ;
#14684=CARTESIAN_POINT ( 'NONE',  ( 2.481649420246374138, 21.62180007765648426, -0.8687765177876252132 ) ) ;
#14686=CARTESIAN_POINT ( 'NONE',  ( 0.05938372350919016857, 20.12819992234354416, -4.731580009072201776 ) ) ;
#14700=CARTESIAN_POINT ( 'NONE',  ( -0.8262555684460826111, 26.50319992234354771, 2.360188852285421302 ) ) ;
#14703=CARTESIAN_POINT ( 'NONE',  ( 2.115076519116362963, 23.87180007765647005, -3.012182706137107147 ) ) ;
#14718=CARTESIAN_POINT ( 'NONE',  ( 0.7188294034286049072, 33.74680007765648071, -2.395093729190366005 ) ) ;
#14720=CARTESIAN_POINT ( 'NONE',  ( -3.500000000000000444, 30.49680007765647716, 0.05647727720536892260 ) ) ;
#14725=CARTESIAN_POINT ( 'NONE',  ( -2.115076519116425580, 17.37819992234354771, -3.012182706137062738 ) ) ;
#14728=CARTESIAN_POINT ( 'NONE',  ( 1.444289557196047680, 39.74680007765648071, 4.262301884875704161 ) ) ;
#14749=CARTESIAN_POINT ( 'NONE',  ( 2.733110507866328920, 23.62819992234354416, 3.862833514489095510 ) ) ;
#14750=CARTESIAN_POINT ( 'NONE',  ( -3.481649420246394566, 32.12819992234354061, -1.193696214020467883 ) ) ;
#14751=CARTESIAN_POINT ( 'NONE',  ( -0.8262555684460826111, 21.50319992234354771, 2.360188852285421302 ) ) ;
#14753=CARTESIAN_POINT ( 'NONE',  ( 3.607379964056306676, 21.49680007765647360, -2.690724712371305838 ) ) ;
#14759=CARTESIAN_POINT ( 'NONE',  ( 2.798362969681366330, 38.99680007765647360, -2.102939460078824929 ) ) ;
#14772=CARTESIAN_POINT ( 'NONE',  ( 2.864755990943222308, 25.50319992234354771, -2.011557305968548093 ) ) ;
#14776=CARTESIAN_POINT ( 'NONE',  ( -0.8262555684461330152, 23.49680007765647716, -2.360188852285403982 ) ) ;
#14777=CARTESIAN_POINT ( 'NONE',  ( 1.336863392178569754, 21.25319992234354771, 4.297206761780648421 ) ) ;
#14781=CARTESIAN_POINT ( 'NONE',  ( -2.733110507866247652, 37.62180007765646650, 3.862833514489154574 ) ) ;
#14794=CARTESIAN_POINT ( 'NONE',  ( 1.593127413382953383, 25.37819992234354416, -2.091722143975172532 ) ) ;
#14797=CARTESIAN_POINT ( 'NONE',  ( -3.518350579753630747, 23.12180007765647716, -1.080741659609802729 ) ) ;
#14813=CARTESIAN_POINT ( 'NONE',  ( 2.481649420246374138, 26.62180007765648426, -0.8687765177876252132 ) ) ;
#14815=CARTESIAN_POINT ( 'NONE',  ( -1.135272562821090014, 25.99680007765648071, -3.311245368580554072 ) ) ;
#14819=CARTESIAN_POINT ( 'NONE',  ( 3.481649420246394122, 15.87819992234354594, 1.193696214020467439 ) ) ;
#14823=CARTESIAN_POINT ( 'NONE',  ( 2.211161402132902243, 19.62180007765647360, 2.942372952327172442 ) ) ;
#14833=ORIENTED_EDGE ( 'NONE', *, *, #12146, .F. ) ;
#14845=CARTESIAN_POINT ( 'NONE',  ( 1.336863392178569754, 28.75319992234354771, 4.297206761780648421 ) ) ;
#14846=CARTESIAN_POINT ( 'NONE',  ( -1.135272562821019626, 36.50319992234354061, 3.311245368580577164 ) ) ;
#14848=CARTESIAN_POINT ( 'NONE',  ( 1.497042530366522461, 16.12819992234354416, 2.161531897785029965 ) ) ;
#14850=CARTESIAN_POINT ( 'NONE',  ( 4.499999999999999112, 16.74680007765647716, -0.05647727720537982360 ) ) ;
#14854=CARTESIAN_POINT ( 'NONE',  ( 1.027846397803542144, 38.74680007765647360, -3.346150245485522312 ) ) ;
#14867=CARTESIAN_POINT ( 'NONE',  ( -3.500000000000000444, 29.50319992234354416, -0.05647727720529563400 ) ) ;
#14871=CARTESIAN_POINT ( 'NONE',  ( 2.500000000000001332, 21.74680007765648071, -0.05647727720535888202 ) ) ;
#14872=CARTESIAN_POINT ( 'NONE',  ( -1.444289557195956863, 19.00319992234354771, 4.262301884875733471 ) ) ;
#14876=CARTESIAN_POINT ( 'NONE',  ( 0.05938372350927906274, 17.37180007765647005, 3.680117784833935701 ) ) ;
#14888=CARTESIAN_POINT ( 'NONE',  ( -0.8262555684460826111, 29.00319992234355482, 2.360188852285421302 ) ) ;
#14891=CARTESIAN_POINT ( 'NONE',  ( 3.500000000000000444, 24.24680007765647716, -0.05647727720536935281 ) ) ;
#14909=CARTESIAN_POINT ( 'NONE',  ( 2.518350579753628971, 26.87180007765648426, 0.7558219633769073242 ) ) ;
#14911=CARTESIAN_POINT ( 'NONE',  ( -2.864755990943265829, 33.24680007765648071, -2.011557305968488141 ) ) ;
#14921=CARTESIAN_POINT ( 'NONE',  ( -2.115076519116362519, 20.12180007765648071, 3.012182706137107147 ) ) ;
#14926=CIRCLE ( 'NONE', #11044, 0.5000000000000026645 ) ;
#14938=CARTESIAN_POINT ( 'NONE',  ( 4.518350579753602325, 35.62819992234354771, -1.405661355842793725 ) ) ;
#14939=CARTESIAN_POINT ( 'NONE',  ( -3.500000000000000444, 34.50319992234354771, -0.05647727720529563400 ) ) ;
#14940=CARTESIAN_POINT ( 'NONE',  ( 0.8262555684460829442, 17.75319992234354061, -2.360188852285421302 ) ) ;
#14943=CARTESIAN_POINT ( 'NONE',  ( -4.499999999999999112, 17.99680007765647005, 0.05647727720537927543 ) ) ;
#14947=CARTESIAN_POINT ( 'NONE',  ( 2.211161402132902243, 34.62180007765648071, 2.942372952327172442 ) ) ;
#14958=CARTESIAN_POINT ( 'NONE',  ( 1.027846397803612311, 23.75319992234354416, 3.346150245485499219 ) ) ;
#14961=CARTESIAN_POINT ( 'NONE',  ( 0.8262555684461332373, 22.24680007765648071, 2.360188852285403982 ) ) ;
#14962=CARTESIAN_POINT ( 'NONE',  ( -2.829195390882724315, 16.62819992234354061, 3.793023760679264722 ) ) ;
#14966=CARTESIAN_POINT ( 'NONE',  ( -3.481649420246369697, 17.87180007765648071, 1.193696214020542490 ) ) ;
#14976=CARTESIAN_POINT ( 'NONE',  ( 2.500000000000001332, 28.25319992234354771, 0.05647727720530566764 ) ) ;
#14978=CARTESIAN_POINT ( 'NONE',  ( 2.115076519116362963, 21.37180007765648071, -3.012182706137107147 ) ) ;
#14982=CARTESIAN_POINT ( 'NONE',  ( 1.336863392178479160, 21.24680007765647716, -4.297206761780677731 ) ) ;
#14989=CARTESIAN_POINT ( 'NONE',  ( 2.518350579753628971, 34.37180007765647360, 0.7558219633769073242 ) ) ;
#14991=CARTESIAN_POINT ( 'NONE',  ( -0.05938372350927861865, 33.62180007765648071, -3.680117784833935701 ) ) ;
#14999=CARTESIAN_POINT ( 'NONE',  ( 2.115076519116362963, 23.87180007765647005, -3.012182706137107147 ) ) ;
#15013=CARTESIAN_POINT ( 'NONE',  ( 3.518350579753631191, 29.37180007765647005, 1.080741659609802285 ) ) ;
#15018=CARTESIAN_POINT ( 'NONE',  ( 1.444289557195957086, 30.25319992234354061, -4.262301884875733471 ) ) ;
#15019=CARTESIAN_POINT ( 'NONE',  ( 3.518350579753606322, 35.62819992234354061, -1.080741659609876892 ) ) ;
#15021=CARTESIAN_POINT ( 'NONE',  ( 1.497042530366522461, 26.12819992234354416, 2.161531897785029965 ) ) ;
#15023=CARTESIAN_POINT ( 'NONE',  ( 4.499999999999999112, 26.74680007765647360, -0.05647727720537982360 ) ) ;
#15039=CARTESIAN_POINT ( 'NONE',  ( 0.05938372350920109732, 32.62819992234354771, -3.680117784833935701 ) ) ;
#15040=CARTESIAN_POINT ( 'NONE',  ( 1.135272562821020070, 15.25319992234354594, -3.311245368580577164 ) ) ;
#15042=CARTESIAN_POINT ( 'NONE',  ( 2.055738996568313048, 29.49680007765648426, 1.423772053676023441 ) ) ;
#15044=CARTESIAN_POINT ( 'NONE',  ( 4.518350579753602325, 15.62819992234354238, -1.405661355842793725 ) ) ;
#15048=CARTESIAN_POINT ( 'NONE',  ( 1.336863392178479160, 38.74680007765646650, -4.297206761780677731 ) ) ;
#15057=CARTESIAN_POINT ( 'NONE',  ( 3.481649420246369697, 16.62180007765648071, -1.193696214020541824 ) ) ;
#15062=CARTESIAN_POINT ( 'NONE',  ( -3.500000000000000444, 14.50319992234354416, -0.05647727720529563400 ) ) ;
#15064=CARTESIAN_POINT ( 'NONE',  ( -2.115076519116362519, 25.12180007765647360, 3.012182706137107147 ) ) ;
#15071=CARTESIAN_POINT ( 'NONE',  ( -3.607379964056306676, 20.24680007765648071, 2.690724712371306282 ) ) ;
#15078=CARTESIAN_POINT ( 'NONE',  ( -1.497042530366477164, 40.12180007765647360, 2.161531897785062384 ) ) ;
#15081=CARTESIAN_POINT ( 'NONE',  ( -2.211161402132901799, 30.87180007765647716, -2.942372952327172886 ) ) ;
#15086=CARTESIAN_POINT ( 'NONE',  ( 3.518350579753631191, 24.37180007765648071, 1.080741659609802285 ) ) ;
#15101=CARTESIAN_POINT ( 'NONE',  ( 2.211161402132902243, 34.62180007765648071, 2.942372952327172442 ) ) ;
#15106=CARTESIAN_POINT ( 'NONE',  ( -1.444289557195956863, 34.00319992234354771, 4.262301884875733471 ) ) ;
#15108=CARTESIAN_POINT ( 'NONE',  ( 2.481649420246391902, 28.37819992234355126, 0.8687765177875720335 ) ) ;
#15110=CARTESIAN_POINT ( 'NONE',  ( 1.336863392178479160, 28.74680007765647360, -4.297206761780677731 ) ) ;
#15113=CARTESIAN_POINT ( 'NONE',  ( 0.05938372350927906274, 34.87180007765645939, 3.680117784833935701 ) ) ;
#15129=CARTESIAN_POINT ( 'NONE',  ( 3.518350579753605434, 33.12819992234354771, -1.080741659609877114 ) ) ;
#15130=CARTESIAN_POINT ( 'NONE',  ( 3.500000000000000444, 18.25319992234354771, 0.05647727720529520379 ) ) ;
#15132=CARTESIAN_POINT ( 'NONE',  ( -2.518350579753628526, 33.12180007765648071, -0.7558219633769075463 ) ) ;
#15134=CARTESIAN_POINT ( 'NONE',  ( -0.05938372350918959958, 28.87819992234354416, 4.731580009072201776 ) ) ;
#15138=CARTESIAN_POINT ( 'NONE',  ( 2.864755990943265829, 16.99680007765647716, 2.011557305968487697 ) ) ;
#15152=CARTESIAN_POINT ( 'NONE',  ( -2.500000000000001332, 37.00319992234354771, -0.05647727720530596601 ) ) ;
#15154=CARTESIAN_POINT ( 'NONE',  ( -1.135272562821090014, 30.99680007765647716, -3.311245368580554072 ) ) ;
#15155=CARTESIAN_POINT ( 'NONE',  ( 2.211161402132839626, 22.87819992234354416, -2.942372952327218183 ) ) ;
#15162=CARTESIAN_POINT ( 'NONE',  ( 4.499999999999999112, 21.74680007765647360, -0.05647727720537982360 ) ) ;
#15171=CARTESIAN_POINT ( 'NONE',  ( 2.518350579753628971, 39.37180007765647360, 0.7558219633769073242 ) ) ;
#15173=CARTESIAN_POINT ( 'NONE',  ( -2.211161402132901799, 35.87180007765648071, -2.942372952327172886 ) ) ;
#15179=CARTESIAN_POINT ( 'NONE',  ( 2.115076519116362963, 26.37180007765648071, -3.012182706137107147 ) ) ;
#15196=CARTESIAN_POINT ( 'NONE',  ( -1.135272562821090014, 38.49680007765647360, -3.311245368580554072 ) ) ;
#15202=CARTESIAN_POINT ( 'NONE',  ( 1.336863392178569754, 36.25319992234354771, 4.297206761780648421 ) ) ;
#15204=CARTESIAN_POINT ( 'NONE',  ( -2.500000000000001332, 24.50319992234354771, -0.05647727720530596601 ) ) ;
#15207=CARTESIAN_POINT ( 'NONE',  ( -4.518350579753632523, 25.62180007765648426, -1.405661355842698468 ) ) ;
#15223=CARTESIAN_POINT ( 'NONE',  ( -1.027846397803611866, 37.50319992234354061, -3.346150245485499219 ) ) ;
#15224=CARTESIAN_POINT ( 'NONE',  ( 2.864755990943222308, 20.50319992234354416, -2.011557305968548093 ) ) ;
#15226=CARTESIAN_POINT ( 'NONE',  ( -2.055738996568313048, 30.74680007765648071, -1.423772053676023441 ) ) ;
#15228=CARTESIAN_POINT ( 'NONE',  ( -3.673772985318163098, 24.25319992234354061, 2.599342558261029001 ) ) ;
#15234=CARTESIAN_POINT ( 'NONE',  ( 2.211161402132902243, 22.12180007765648071, 2.942372952327172442 ) ) ;
#15245=CARTESIAN_POINT ( 'NONE',  ( 0.05938372350927906274, 17.37180007765647005, 3.680117784833935701 ) ) ;
#15251=CARTESIAN_POINT ( 'NONE',  ( -2.518350579753611207, 36.87819992234354061, 0.7558219633769609480 ) ) ;
#15253=CARTESIAN_POINT ( 'NONE',  ( -3.518350579753630747, 30.62180007765647716, -1.080741659609802729 ) ) ;
#15255=CARTESIAN_POINT ( 'NONE',  ( 3.481649420246394122, 23.37819992234353705, 1.193696214020467439 ) ) ;
#15260=CARTESIAN_POINT ( 'NONE',  ( -2.733110507866247652, 22.62180007765647360, 3.862833514489154574 ) ) ;
#15267=CARTESIAN_POINT ( 'NONE',  ( 1.989345975306426206, 36.49680007765648071, -1.515154207786343799 ) ) ;
#15269=CARTESIAN_POINT ( 'NONE',  ( 2.798362969681366330, 38.99680007765647360, -2.102939460078824929 ) ) ;
#15271=CARTESIAN_POINT ( 'NONE',  ( -3.859945489046901823, 15.00000000000001954, -1.030823890046652869 ) ) ;
#15274=CARTESIAN_POINT ( 'NONE',  ( -2.864755990943265829, 28.24680007765648071, -2.011557305968488141 ) ) ;
#15284=CARTESIAN_POINT ( 'NONE',  ( 3.518350579753631191, 39.37180007765646650, 1.080741659609802285 ) ) ;
#15288=CARTESIAN_POINT ( 'NONE',  ( 1.336863392178569754, 33.75319992234354771, 4.297206761780648421 ) ) ;
#15291=CARTESIAN_POINT ( 'NONE',  ( -1.497042530366522461, 24.87819992234354771, -2.161531897785030409 ) ) ;
#15294=CARTESIAN_POINT ( 'NONE',  ( -3.673772985318219053, 25.74680007765648426, -2.599342558260952174 ) ) ;
#15312=CARTESIAN_POINT ( 'NONE',  ( 2.798362969681409851, 36.00319992234354771, 2.102939460078764977 ) ) ;
#15313=CARTESIAN_POINT ( 'NONE',  ( -2.211161402132838738, 21.62819992234354771, 2.942372952327218183 ) ) ;
#15315=CARTESIAN_POINT ( 'NONE',  ( -1.497042530366477164, 30.12180007765648426, 2.161531897785062384 ) ) ;
#15317=CARTESIAN_POINT ( 'NONE',  ( 3.607379964056363075, 28.50319992234354416, 2.690724712371229010 ) ) ;
#15321=CARTESIAN_POINT ( 'NONE',  ( -2.864755990943265829, 20.74680007765647716, -2.011557305968488141 ) ) ;
#15335=CARTESIAN_POINT ( 'NONE',  ( 0.05938372350921204690, 35.12819992234354771, -2.628655560595669183 ) ) ;
#15338=CARTESIAN_POINT ( 'NONE',  ( 2.864755990943265829, 34.49680007765648071, 2.011557305968487697 ) ) ;
#15339=CARTESIAN_POINT ( 'NONE',  ( 2.211161402132839626, 27.87819992234354061, -2.942372952327218183 ) ) ;
#15355=CARTESIAN_POINT ( 'NONE',  ( 1.593127413382998903, 39.62180007765647360, 2.091722143975139669 ) ) ;
#15358=CARTESIAN_POINT ( 'NONE',  ( -2.115076519116362519, 37.62180007765647360, 3.012182706137108035 ) ) ;
#15362=CARTESIAN_POINT ( 'NONE',  ( -3.721472675004220854, 15.00000000000001421, -1.423657464930958128 ) ) ;
#15366=CARTESIAN_POINT ( 'NONE',  ( 2.115076519116362963, 21.37180007765648071, -3.012182706137107147 ) ) ;
#15377=CARTESIAN_POINT ( 'NONE',  ( -1.135272562821090014, 35.99680007765648071, -3.311245368580554072 ) ) ;
#15382=CARTESIAN_POINT ( 'NONE',  ( 4.499999999999999112, 16.74680007765647716, -0.05647727720537982360 ) ) ;
#15383=VECTOR ( 'NONE', #17609, 1000.000000000000000 ) ;
#15385=CARTESIAN_POINT ( 'NONE',  ( 2.500000000000001332, 28.25319992234354771, 0.05647727720530566764 ) ) ;
#15388=CARTESIAN_POINT ( 'NONE',  ( -4.481649420246366589, 22.87180007765647360, 1.518615910253458878 ) ) ;
#15406=CARTESIAN_POINT ( 'NONE',  ( 0.05938372350927906967, 22.37180007765648071, 3.680117784833935701 ) ) ;
#15409=CARTESIAN_POINT ( 'NONE',  ( 3.607379964056363075, 16.00319992234354416, 2.690724712371229010 ) ) ;
#15410=CARTESIAN_POINT ( 'NONE',  ( -2.864755990943222308, 21.75319992234354771, 2.011557305968548093 ) ) ;
#15412=CARTESIAN_POINT ( 'NONE',  ( 2.518350579753628971, 29.37180007765648426, 0.7558219633769073242 ) ) ;
#15413=CARTESIAN_POINT ( 'NONE',  ( 3.673772985318163098, 23.00319992234354416, -2.599342558261029001 ) ) ;
#15418=CARTESIAN_POINT ( 'NONE',  ( -2.864755990943265829, 18.24680007765648071, -2.011557305968488141 ) ) ;
#15427=CARTESIAN_POINT ( 'NONE',  ( -1.135272562821090014, 23.49680007765647716, -3.311245368580554072 ) ) ;
#15432=CARTESIAN_POINT ( 'NONE',  ( 1.497042530366522461, 38.62819992234354771, 2.161531897785029965 ) ) ;
#15434=CARTESIAN_POINT ( 'NONE',  ( -3.481649420246369697, 27.87180007765647360, 1.193696214020542490 ) ) ;
#15435=CARTESIAN_POINT ( 'NONE',  ( 2.864755990943222308, 30.50319992234354416, -2.011557305968548093 ) ) ;
#15447=CARTESIAN_POINT ( 'NONE',  ( 0.7188294034286553114, 16.25319992234354771, 2.395093729190349130 ) ) ;
#15456=CARTESIAN_POINT ( 'NONE',  ( -3.500000000000000444, 32.99680007765648071, 0.05647727720536892260 ) ) ;
#15470=CARTESIAN_POINT ( 'NONE',  ( 2.055738996568313048, 16.99680007765648071, 1.423772053676023441 ) ) ;
#15474=CARTESIAN_POINT ( 'NONE',  ( 4.499999999999999112, 38.25319992234354061, 0.05647727720528474687 ) ) ;
#15477=CARTESIAN_POINT ( 'NONE',  ( 1.497042530366522461, 36.12819992234354771, 2.161531897785029965 ) ) ;
#15481=CARTESIAN_POINT ( 'NONE',  ( 4.499999999999999112, 36.74680007765647360, -0.05647727720537982360 ) ) ;
#15494=CARTESIAN_POINT ( 'NONE',  ( -4.481649420246396787, 19.62819992234354416, -1.518615910253363399 ) ) ;
#15495=CARTESIAN_POINT ( 'NONE',  ( 0.05938372350920110426, 22.62819992234354416, -3.680117784833935701 ) ) ;
#15497=CARTESIAN_POINT ( 'NONE',  ( 2.055738996568313048, 36.99680007765647360, 1.423772053676023441 ) ) ;
#15499=CARTESIAN_POINT ( 'NONE',  ( -3.673772985318163098, 26.75319992234354771, 2.599342558261029001 ) ) ;
#15505=CARTESIAN_POINT ( 'NONE',  ( -0.05938372350927861171, 23.62180007765647005, -3.680117784833935701 ) ) ;
#15512=CARTESIAN_POINT ( 'NONE',  ( 1.135272562821090458, 22.24680007765648071, 3.311245368580554072 ) ) ;
#15517=CARTESIAN_POINT ( 'NONE',  ( -2.864755990943222308, 21.75319992234354771, 2.011557305968548093 ) ) ;
#15519=CARTESIAN_POINT ( 'NONE',  ( -2.115076519116362519, 40.12180007765648071, 3.012182706137107147 ) ) ;
#15520=CARTESIAN_POINT ( 'NONE',  ( -3.500000000000000444, 27.00319992234354771, -0.05647727720529563400 ) ) ;
#15533=CARTESIAN_POINT ( 'NONE',  ( -0.7188294034286550893, 17.50319992234354771, -2.395093729190349130 ) ) ;
#15539=CARTESIAN_POINT ( 'NONE',  ( -2.211161402132902243, 35.87180007765648782, -2.942372952327172886 ) ) ;
#15551=CARTESIAN_POINT ( 'NONE',  ( -2.481649420246374138, 17.87180007765647716, 0.8687765177876256573 ) ) ;
#15556=CARTESIAN_POINT ( 'NONE',  ( 1.593127413382953383, 32.87819992234354771, -2.091722143975172532 ) ) ;
#15560=CARTESIAN_POINT ( 'NONE',  ( 3.673772985318219053, 31.99680007765648071, 2.599342558260951730 ) ) ;
#15573=CARTESIAN_POINT ( 'NONE',  ( 4.499999999999999112, 20.75319992234354416, 0.05647727720528474687 ) ) ;
#15574=CARTESIAN_POINT ( 'NONE',  ( -3.518350579753606322, 26.87819992234354771, 1.080741659609877781 ) ) ;
#15577=CARTESIAN_POINT ( 'NONE',  ( 1.593127413382953383, 15.37819992234354594, -2.091722143975172532 ) ) ;
#15578=CARTESIAN_POINT ( 'NONE',  ( 3.607379964056363075, 33.50319992234354061, 2.690724712371229010 ) ) ;
#15582=CARTESIAN_POINT ( 'NONE',  ( 2.115076519116362963, 21.37180007765648071, -3.012182706137107147 ) ) ;
#15587=CARTESIAN_POINT ( 'NONE',  ( 2.733110507866247652, 26.37180007765647716, -3.862833514489153686 ) ) ;
#15592=CARTESIAN_POINT ( 'NONE',  ( 2.115076519116362963, 21.37180007765648071, -3.012182706137107147 ) ) ;
#15597=CARTESIAN_POINT ( 'NONE',  ( -3.500000000000000444, 17.00319992234354416, -0.05647727720529563400 ) ) ;
#15599=CARTESIAN_POINT ( 'NONE',  ( 3.481649420246369697, 39.12180007765646650, -1.193696214020541824 ) ) ;
#15601=CARTESIAN_POINT ( 'NONE',  ( -2.864755990943222308, 34.25319992234354771, 2.011557305968548093 ) ) ;
#15614=CARTESIAN_POINT ( 'NONE',  ( -1.593127413382952939, 24.12819992234354771, 2.091722143975172532 ) ) ;
#15617=CARTESIAN_POINT ( 'NONE',  ( -2.211161402132902243, 18.37180007765647005, -2.942372952327172886 ) ) ;
#15623=CARTESIAN_POINT ( 'NONE',  ( 2.115076519116362963, 28.87180007765647716, -3.012182706137107147 ) ) ;
#15637=CARTESIAN_POINT ( 'NONE',  ( 1.989345975306426206, 18.99680007765647716, -1.515154207786343799 ) ) ;
#15643=CARTESIAN_POINT ( 'NONE',  ( 0.05938372350921204690, 37.62819992234354771, -2.628655560595669183 ) ) ;
#15646=CARTESIAN_POINT ( 'NONE',  ( 0.05938372350929014415, 32.37180007765647360, 4.731580009072201776 ) ) ;
#15664=CARTESIAN_POINT ( 'NONE',  ( 1.444289557195957086, 20.25319992234354416, -4.262301884875733471 ) ) ;
#15665=CARTESIAN_POINT ( 'NONE',  ( -2.211161402132838738, 31.62819992234354416, 2.942372952327218183 ) ) ;
#15666=CARTESIAN_POINT ( 'NONE',  ( -0.8262555684461330152, 38.49680007765647360, -2.360188852285403982 ) ) ;
#15669=CARTESIAN_POINT ( 'NONE',  ( -4.499999999999999112, 32.00319992234354061, -0.05647727720528529505 ) ) ;
#15677=CARTESIAN_POINT ( 'NONE',  ( 2.798362969681366330, 28.99680007765647716, -2.102939460078824929 ) ) ;
#15682=CARTESIAN_POINT ( 'NONE',  ( 4.518350579753633411, 31.87180007765647716, 1.405661355842698468 ) ) ;
#15686=CARTESIAN_POINT ( 'NONE',  ( 3.518350579753631191, 26.87180007765647360, 1.080741659609802285 ) ) ;
#15690=CARTESIAN_POINT ( 'NONE',  ( 3.481649420246394122, 18.37819992234354771, 1.193696214020467439 ) ) ;
#15692=CARTESIAN_POINT ( 'NONE',  ( -2.864755990943265829, 35.74680007765648071, -2.011557305968488141 ) ) ;
#15694=CARTESIAN_POINT ( 'NONE',  ( 0.05938372350920109732, 37.62819992234352640, -3.680117784833935701 ) ) ;
#15707=CARTESIAN_POINT ( 'NONE',  ( 2.500000000000001332, 18.25319992234354771, 0.05647727720530566764 ) ) ;
#15715=CARTESIAN_POINT ( 'NONE',  ( -2.864755990943265829, 33.24680007765648071, -2.011557305968488141 ) ) ;
#15728=CARTESIAN_POINT ( 'NONE',  ( -2.481649420246374138, 22.87180007765648071, 0.8687765177876256573 ) ) ;
#15730=CARTESIAN_POINT ( 'NONE',  ( -2.864755990943265829, 18.24680007765648071, -2.011557305968488141 ) ) ;
#15734=CARTESIAN_POINT ( 'NONE',  ( 2.518350579753611207, 33.12819992234354771, -0.7558219633769606149 ) ) ;
#15738=CARTESIAN_POINT ( 'NONE',  ( 4.499999999999999112, 31.74680007765647716, -0.05647727720537982360 ) ) ;
#15740=MECHANICAL_DESIGN_GEOMETRIC_PRESENTATION_REPRESENTATION('',(#12185),#1541);
#15756=CARTESIAN_POINT ( 'NONE',  ( 1.336863392178569754, 18.75319992234354416, 4.297206761780648421 ) ) ;
#15757=CARTESIAN_POINT ( 'NONE',  ( -2.211161402132838738, 29.12819992234354416, 2.942372952327218183 ) ) ;
#15758=CARTESIAN_POINT ( 'NONE',  ( -1.497042530366522461, 14.87819992234354594, -2.161531897785030409 ) ) ;
#15760=CARTESIAN_POINT ( 'NONE',  ( -4.481649420246396787, 34.62819992234354771, -1.518615910253363399 ) ) ;
#15766=CARTESIAN_POINT ( 'NONE',  ( 3.481649420246369697, 31.62180007765647360, -1.193696214020541824 ) ) ;
#15769=CARTESIAN_POINT ( 'NONE',  ( -2.733110507866247652, 30.12180007765647716, 3.862833514489154574 ) ) ;
#15773=CARTESIAN_POINT ( 'NONE',  ( 1.135272562821090458, 19.74680007765648071, 3.311245368580554072 ) ) ;
#15781=CARTESIAN_POINT ( 'NONE',  ( -0.05938372350920063936, 21.37819992234353705, 3.680117784833935701 ) ) ;
#15785=CARTESIAN_POINT ( 'NONE',  ( -0.8262555684461330152, 15.99680007765648249, -2.360188852285403982 ) ) ;
#15788=CARTESIAN_POINT ( 'NONE',  ( 0.05938372350920109732, 32.62819992234354771, -3.680117784833935701 ) ) ;
#15801=CARTESIAN_POINT ( 'NONE',  ( -2.238531268403934682, 15.00000000000000355, -2.169313016320178367 ) ) ;
#15803=CARTESIAN_POINT ( 'NONE',  ( -1.593127413382952939, 21.62819992234354416, 2.091722143975172532 ) ) ;
#15807=CARTESIAN_POINT ( 'NONE',  ( -4.518350579753602325, 39.37819992234354771, 1.405661355842794391 ) ) ;
#15812=CARTESIAN_POINT ( 'NONE',  ( 2.115076519116362963, 33.87180007765648071, -3.012182706137107147 ) ) ;
#15824=CARTESIAN_POINT ( 'NONE',  ( 1.497042530366477164, 23.87180007765647716, -2.161531897785062384 ) ) ;
#15826=CARTESIAN_POINT ( 'NONE',  ( 2.115076519116362963, 18.87180007765648071, -3.012182706137107591 ) ) ;
#15830=CARTESIAN_POINT ( 'NONE',  ( -2.864755990943222308, 21.75319992234354771, 2.011557305968548093 ) ) ;
#15833=CARTESIAN_POINT ( 'NONE',  ( -0.05938372350928957516, 36.12180007765646650, -4.731580009072201776 ) ) ;
#15850=CARTESIAN_POINT ( 'NONE',  ( 2.733110507866328920, 28.62819992234354416, 3.862833514489095510 ) ) ;
#15851=CARTESIAN_POINT ( 'NONE',  ( -3.518350579753606322, 29.37819992234354771, 1.080741659609877781 ) ) ;
#15853=CARTESIAN_POINT ( 'NONE',  ( 2.500000000000001332, 39.24680007765647360, -0.05647727720535888202 ) ) ;
#15855=CARTESIAN_POINT ( 'NONE',  ( 1.444289557195957086, 30.25319992234354061, -4.262301884875733471 ) ) ;
#15860=CARTESIAN_POINT ( 'NONE',  ( 3.481649420246369697, 26.62180007765648071, -1.193696214020541824 ) ) ;
#15864=CARTESIAN_POINT ( 'NONE',  ( 1.336863392178479160, 28.74680007765647360, -4.297206761780677731 ) ) ;
#15869=CARTESIAN_POINT ( 'NONE',  ( 1.027846397803542144, 28.74680007765647716, -3.346150245485522312 ) ) ;
#15875=CARTESIAN_POINT ( 'NONE',  ( 2.115076519116426024, 18.62819992234354771, 3.012182706137062294 ) ) ;
#15877=CARTESIAN_POINT ( 'NONE',  ( -1.497042530366477164, 17.62180007765648071, 2.161531897785062384 ) ) ;
#15878=CARTESIAN_POINT ( 'NONE',  ( -3.518350579753605434, 34.37819992234354771, 1.080741659609877781 ) ) ;
#15895=CARTESIAN_POINT ( 'NONE',  ( -2.500000000000001332, 19.50319992234354771, -0.05647727720530596601 ) ) ;
#15902=CARTESIAN_POINT ( 'NONE',  ( -2.115076519116362519, 40.12180007765648071, 3.012182706137107147 ) ) ;
#15915=CARTESIAN_POINT ( 'NONE',  ( 1.497042530366477164, 26.37180007765647716, -2.161531897785062384 ) ) ;
#15917=CARTESIAN_POINT ( 'NONE',  ( -3.518350579753630303, 20.62180007765647360, -1.080741659609802952 ) ) ;
#15924=CARTESIAN_POINT ( 'NONE',  ( -3.481649420246394122, 19.62819992234354416, -1.193696214020467883 ) ) ;
#15927=CARTESIAN_POINT ( 'NONE',  ( -3.481649420246369697, 17.87180007765648071, 1.193696214020542490 ) ) ;
#15947=CARTESIAN_POINT ( 'NONE',  ( -3.607379964056363075, 27.25319992234354771, -2.690724712371229899 ) ) ;
#15948=CARTESIAN_POINT ( 'NONE',  ( 2.211161402132839182, 27.87819992234353705, -2.942372952327217739 ) ) ;
#15949=CARTESIAN_POINT ( 'NONE',  ( 2.481649420246391902, 23.37819992234354771, 0.8687765177875720335 ) ) ;
#15952=CARTESIAN_POINT ( 'NONE',  ( -2.829195390882724315, 36.62819992234354771, 3.793023760679264722 ) ) ;
#15954=AXIS2_PLACEMENT_3D ( 'NONE', #8191, #13854, #1161 ) ;
#15958=CARTESIAN_POINT ( 'NONE',  ( -2.211161402132902243, 33.37180007765648071, -2.942372952327172886 ) ) ;
#15962=CARTESIAN_POINT ( 'NONE',  ( -0.05938372350928957516, 28.62180007765647005, -4.731580009072201776 ) ) ;
#15968=CARTESIAN_POINT ( 'NONE',  ( -3.481649420246369697, 32.87180007765645939, 1.193696214020542490 ) ) ;
#15973=CARTESIAN_POINT ( 'NONE',  ( 3.518350579753605434, 28.12819992234354416, -1.080741659609877114 ) ) ;
#15976=CARTESIAN_POINT ( 'NONE',  ( 0.8262555684461332373, 24.74680007765647716, 2.360188852285403982 ) ) ;
#15977=CARTESIAN_POINT ( 'NONE',  ( 2.211161402132839626, 32.87819992234354771, -2.942372952327218183 ) ) ;
#15995=CARTESIAN_POINT ( 'NONE',  ( 2.055738996568281518, 25.50319992234354416, -1.423772053676066518 ) ) ;
#15997=CARTESIAN_POINT ( 'NONE',  ( -2.115076519116362519, 17.62180007765647716, 3.012182706137107147 ) ) ;
#16012=CARTESIAN_POINT ( 'NONE',  ( -0.05938372350926768989, 18.62180007765648071, -2.628655560595669183 ) ) ;
#16014=CARTESIAN_POINT ( 'NONE',  ( -3.481649420246370141, 22.87180007765647716, 1.193696214020542268 ) ) ;
#16021=CARTESIAN_POINT ( 'NONE',  ( -1.135272562821019626, 19.00319992234354771, 3.311245368580577164 ) ) ;
#16025=CARTESIAN_POINT ( 'NONE',  ( -4.481649420246366589, 40.37180007765647360, 1.518615910253458878 ) ) ;
#16045=CARTESIAN_POINT ( 'NONE',  ( 4.499999999999999112, 28.25319992234354416, 0.05647727720528474687 ) ) ;
#16046=CARTESIAN_POINT ( 'NONE',  ( 2.864755990943222308, 38.00319992234354061, -2.011557305968548093 ) ) ;
#16047=CARTESIAN_POINT ( 'NONE',  ( -0.8262555684460826111, 16.50319992234354416, 2.360188852285421302 ) ) ;
#16048=EDGE_LOOP ( 'NONE', ( #4043, #16622, #14833 ) ) ;
#16050=CARTESIAN_POINT ( 'NONE',  ( -0.05938372350928957516, 16.12180007765647716, -4.731580009072201776 ) ) ;
#16054=CARTESIAN_POINT ( 'NONE',  ( 2.798362969681366330, 31.49680007765647716, -2.102939460078824929 ) ) ;
#16057=CARTESIAN_POINT ( 'NONE',  ( -3.673772985318219053, 33.24680007765647360, -2.599342558260952174 ) ) ;
#16061=CARTESIAN_POINT ( 'NONE',  ( 2.211161402132902243, 32.12180007765647360, 2.942372952327172442 ) ) ;
#16066=CARTESIAN_POINT ( 'NONE',  ( -3.518350579753605434, 26.87819992234354416, 1.080741659609877781 ) ) ;
#16069=CARTESIAN_POINT ( 'NONE',  ( -2.055738996568313048, 18.24680007765647716, -1.423772053676023441 ) ) ;
#16071=CARTESIAN_POINT ( 'NONE',  ( 4.518350579753602325, 18.12819992234354416, -1.405661355842793725 ) ) ;
#16089=CARTESIAN_POINT ( 'NONE',  ( 2.518350579753611207, 25.62819992234354416, -0.7558219633769606149 ) ) ;
#16093=CARTESIAN_POINT ( 'NONE',  ( -3.518350579753630747, 20.62180007765646650, -1.080741659609802729 ) ) ;
#16109=CARTESIAN_POINT ( 'NONE',  ( 1.593127413382998903, 27.12180007765647716, 2.091722143975139669 ) ) ;
#16111=CARTESIAN_POINT ( 'NONE',  ( 3.518350579753631191, 26.87180007765647716, 1.080741659609802729 ) ) ;
#16115=CARTESIAN_POINT ( 'NONE',  ( 2.211161402132839626, 20.37819992234354416, -2.942372952327218183 ) ) ;
#16118=CARTESIAN_POINT ( 'NONE',  ( 2.829195390882805583, 39.62180007765647360, 3.793023760679204770 ) ) ;
#16140=CARTESIAN_POINT ( 'NONE',  ( 2.829195390882724759, 25.37819992234354416, -3.793023760679264278 ) ) ;
#16142=CARTESIAN_POINT ( 'NONE',  ( -0.7188294034286550893, 20.00319992234354771, -2.395093729190349130 ) ) ;
#16144=CARTESIAN_POINT ( 'NONE',  ( -0.05938372350928957516, 21.12180007765647360, -4.731580009072201776 ) ) ;
#16147=CARTESIAN_POINT ( 'NONE',  ( -2.864755990943265829, 35.74680007765648071, -2.011557305968488141 ) ) ;
#16158=CARTESIAN_POINT ( 'NONE',  ( -1.135272562821019626, 24.00319992234354416, 3.311245368580577164 ) ) ;
#16161=CARTESIAN_POINT ( 'NONE',  ( 0.7188294034286049072, 21.24680007765648426, -2.395093729190366005 ) ) ;
#16162=CARTESIAN_POINT ( 'NONE',  ( 3.607379964056363075, 21.00319992234354416, 2.690724712371229010 ) ) ;
#16175=CARTESIAN_POINT ( 'NONE',  ( -0.8262555684460826111, 31.50319992234354416, 2.360188852285421302 ) ) ;
#16177=CARTESIAN_POINT ( 'NONE',  ( 3.500000000000000444, 26.74680007765648071, -0.05647727720536935281 ) ) ;
#16195=CARTESIAN_POINT ( 'NONE',  ( -1.989345975306426206, 32.74680007765648071, 1.515154207786343799 ) ) ;
#16197=CARTESIAN_POINT ( 'NONE',  ( -3.481649420246370141, 27.87180007765647716, 1.193696214020542268 ) ) ;
#16201=CARTESIAN_POINT ( 'NONE',  ( -1.027846397803611866, 17.50319992234354416, -3.346150245485499219 ) ) ;
#16205=CARTESIAN_POINT ( 'NONE',  ( -0.05938372350927861171, 18.62180007765647005, -3.680117784833935701 ) ) ;
#16224=CARTESIAN_POINT ( 'NONE',  ( 2.829195390882724759, 27.87819992234354416, -3.793023760679264278 ) ) ;
#16225=CARTESIAN_POINT ( 'NONE',  ( -2.864755990943222308, 34.25319992234354771, 2.011557305968548093 ) ) ;
#16226=CARTESIAN_POINT ( 'NONE',  ( -1.989345975306457071, 19.75319992234354771, -1.515154207786300944 ) ) ;
#16228=CARTESIAN_POINT ( 'NONE',  ( -4.499999999999999112, 20.49680007765647716, 0.05647727720537927543 ) ) ;
#16236=CARTESIAN_POINT ( 'NONE',  ( -3.481649420246369697, 37.87180007765648071, 1.193696214020542490 ) ) ;
#16248=CARTESIAN_POINT ( 'NONE',  ( 2.115076519116426024, 31.12819992234354061, 3.012182706137062294 ) ) ;
#16249=CARTESIAN_POINT ( 'NONE',  ( 2.798362969681409851, 16.00319992234354416, 2.102939460078764977 ) ) ;
#16252=CARTESIAN_POINT ( 'NONE',  ( -1.593127413382998459, 20.87180007765648426, -2.091722143975139669 ) ) ;
#16254=CARTESIAN_POINT ( 'NONE',  ( -3.607379964056363075, 14.75319992234354416, -2.690724712371229899 ) ) ;
#16260=CARTESIAN_POINT ( 'NONE',  ( -2.864755990943265829, 15.74680007765647716, -2.011557305968488141 ) ) ;
#16272=CARTESIAN_POINT ( 'NONE',  ( 0.05938372350921204690, 25.12819992234354416, -2.628655560595669183 ) ) ;
#16274=CARTESIAN_POINT ( 'NONE',  ( 2.211161402132902243, 19.62180007765647360, 2.942372952327172442 ) ) ;
#16289=DIRECTION ( 'NONE',  ( 1.028113302204111856E-14, -0.1129545544106654864, 0.9936001553129347741 ) ) ;
#16290=CARTESIAN_POINT ( 'NONE',  ( -2.500000000000001332, 30.49680007765648071, 0.05647727720535858364 ) ) ;
#16292=CARTESIAN_POINT ( 'NONE',  ( -3.500000000000000444, 32.99680007765648071, 0.05647727720536892260 ) ) ;
#16294=PRODUCT_CONTEXT ( 'NONE', #7947, 'mechanical' ) ;
#16299=CARTESIAN_POINT ( 'NONE',  ( -0.05938372350927861171, 16.12180007765647716, -3.680117784833935701 ) ) ;
#16317=CARTESIAN_POINT ( 'NONE',  ( 4.518350579753602325, 30.62819992234354416, -1.405661355842793725 ) ) ;
#16318=CARTESIAN_POINT ( 'NONE',  ( -3.518350579753606322, 34.37819992234354771, 1.080741659609877781 ) ) ;
#16319=CARTESIAN_POINT ( 'NONE',  ( 0.8262555684460829442, 20.25319992234354771, -2.360188852285421302 ) ) ;
#16321=CARTESIAN_POINT ( 'NONE',  ( -1.444289557196047014, 18.49680007765647360, -4.262301884875704161 ) ) ;
#16327=CARTESIAN_POINT ( 'NONE',  ( -0.05938372350927861171, 38.62180007765648071, -3.680117784833935701 ) ) ;
#16337=CARTESIAN_POINT ( 'NONE',  ( 3.481649420246394122, 23.37819992234353705, 1.193696214020467439 ) ) ;
#16340=CARTESIAN_POINT ( 'NONE',  ( -1.593127413382998459, 25.87180007765647716, -2.091722143975139669 ) ) ;
#16341=CARTESIAN_POINT ( 'NONE',  ( -1.135272562821019626, 39.00319992234354061, 3.311245368580577164 ) ) ;
#16346=CARTESIAN_POINT ( 'NONE',  ( -2.798362969681365886, 17.74680007765647716, 2.102939460078824929 ) ) ;
#16363=CARTESIAN_POINT ( 'NONE',  ( -0.7188294034286550893, 27.50319992234354771, -2.395093729190349130 ) ) ;
#16366=CARTESIAN_POINT ( 'NONE',  ( 3.481649420246369697, 26.62180007765648071, -1.193696214020541824 ) ) ;
#16375=CARTESIAN_POINT ( 'NONE',  ( 1.444289557196047680, 19.74680007765647716, 4.262301884875704161 ) ) ;
#16382=CARTESIAN_POINT ( 'NONE',  ( -1.593127413382998459, 33.37180007765648071, -2.091722143975139669 ) ) ;
#16384=CARTESIAN_POINT ( 'NONE',  ( -0.05938372350927861865, 28.62180007765647716, -3.680117784833935701 ) ) ;
#16391=CARTESIAN_POINT ( 'NONE',  ( 2.798362969681366330, 21.49680007765647716, -2.102939460078824929 ) ) ;
#16405=CARTESIAN_POINT ( 'NONE',  ( -1.135272562821090014, 30.99680007765647716, -3.311245368580554072 ) ) ;
#16410=CARTESIAN_POINT ( 'NONE',  ( 4.481649420246397675, 35.87819992234354771, 1.518615910253363177 ) ) ;
#16411=CARTESIAN_POINT ( 'NONE',  ( 3.500000000000000444, 33.25319992234354771, 0.05647727720529520379 ) ) ;
#16412=CARTESIAN_POINT ( 'NONE',  ( 2.481649420246391902, 25.87819992234355126, 0.8687765177875720335 ) ) ;
#16415=CARTESIAN_POINT ( 'NONE',  ( 3.607379964056306676, 26.49680007765647716, -2.690724712371305838 ) ) ;
#16420=CARTESIAN_POINT ( 'NONE',  ( -3.518350579753630747, 38.12180007765648071, -1.080741659609802729 ) ) ;
#16434=CARTESIAN_POINT ( 'NONE',  ( -3.500000000000000444, 37.00319992234354061, -0.05647727720529563400 ) ) ;
#16438=CARTESIAN_POINT ( 'NONE',  ( 2.481649420246374138, 29.12180007765648426, -0.8687765177876252132 ) ) ;
#16439=CARTESIAN_POINT ( 'NONE',  ( 3.607379964056363075, 16.00319992234354416, 2.690724712371229010 ) ) ;
#16443=CARTESIAN_POINT ( 'NONE',  ( -2.829195390882805139, 38.37180007765647360, -3.793023760679206102 ) ) ;
#16448=ORIENTED_EDGE ( 'NONE', *, *, #4562, .T. ) ;
#16453=CARTESIAN_POINT ( 'NONE',  ( 2.518350579753611207, 33.12819992234354771, -0.7558219633769606149 ) ) ;
#16455=CARTESIAN_POINT ( 'NONE',  ( -1.027846397803541700, 19.99680007765648071, 3.346150245485522312 ) ) ;
#16462=CARTESIAN_POINT ( 'NONE',  ( -2.829195390882805139, 25.87180007765647716, -3.793023760679206102 ) ) ;
#16470=CARTESIAN_POINT ( 'NONE',  ( 0.05938372350926800214, 29.87180007765648426, 2.628655560595669183 ) ) ;
#16473=CARTESIAN_POINT ( 'NONE',  ( -2.115076519116362519, 30.12180007765647716, 3.012182706137108035 ) ) ;
#16481=CARTESIAN_POINT ( 'NONE',  ( 2.864755990943265829, 26.99680007765648071, 2.011557305968487697 ) ) ;
#16495=CARTESIAN_POINT ( 'NONE',  ( 2.115076519116362963, 31.37180007765647716, -3.012182706137107147 ) ) ;
#16500=CARTESIAN_POINT ( 'NONE',  ( 3.607379964056363075, 31.00319992234354771, 2.690724712371229010 ) ) ;
#16503=CARTESIAN_POINT ( 'NONE',  ( 0.7188294034286553114, 31.25319992234354416, 2.395093729190349130 ) ) ;
#16505=CARTESIAN_POINT ( 'NONE',  ( -4.499999999999999112, 25.49680007765647716, 0.05647727720537927543 ) ) ;
#16509=CARTESIAN_POINT ( 'NONE',  ( 3.481649420246369697, 39.12180007765646650, -1.193696214020541824 ) ) ;
#16522=CARTESIAN_POINT ( 'NONE',  ( 2.798362969681409851, 38.50319992234354061, 2.102939460078764977 ) ) ;
#16525=CARTESIAN_POINT ( 'NONE',  ( -2.481649420246374138, 32.87180007765648071, 0.8687765177876256573 ) ) ;
#16527=CARTESIAN_POINT ( 'NONE',  ( 4.518350579753602325, 28.12819992234354416, -1.405661355842793725 ) ) ;
#16533=CARTESIAN_POINT ( 'NONE',  ( -4.481649420246366589, 40.37180007765647360, 1.518615910253458878 ) ) ;
#16545=CARTESIAN_POINT ( 'NONE',  ( -2.798362969681365886, 17.74680007765647716, 2.102939460078824929 ) ) ;
#16550=CARTESIAN_POINT ( 'NONE',  ( 2.500000000000001332, 38.25319992234354771, 0.05647727720530566764 ) ) ;
#16552=CARTESIAN_POINT ( 'NONE',  ( 0.05938372350927906274, 29.87180007765648071, 3.680117784833935701 ) ) ;
#16553=CARTESIAN_POINT ( 'NONE',  ( 2.864755990943222308, 28.00319992234354416, -2.011557305968548093 ) ) ;
#16561=CARTESIAN_POINT ( 'NONE',  ( -4.481649420246366589, 25.37180007765648426, 1.518615910253458878 ) ) ;
#16568=CARTESIAN_POINT ( 'NONE',  ( 1.989345975306426206, 38.99680007765648071, -1.515154207786343799 ) ) ;
#16570=CARTESIAN_POINT ( 'NONE',  ( 3.481649420246370141, 39.12180007765646650, -1.193696214020541602 ) ) ;
#16577=CARTESIAN_POINT ( 'NONE',  ( -1.027846397803541700, 24.99680007765647716, 3.346150245485522312 ) ) ;
#16590=CARTESIAN_POINT ( 'NONE',  ( -2.055738996568313048, 18.24680007765647716, -1.423772053676023441 ) ) ;
#16596=CARTESIAN_POINT ( 'NONE',  ( 0.05938372350919016857, 37.62819992234354771, -4.731580009072201776 ) ) ;
#16600=CARTESIAN_POINT ( 'NONE',  ( -0.05938372350921170689, 28.87819992234354416, 2.628655560595669183 ) ) ;
#16604=CARTESIAN_POINT ( 'NONE',  ( 2.829195390882805583, 22.12180007765647716, 3.793023760679204770 ) ) ;
#16622=ORIENTED_EDGE ( 'NONE', *, *, #10080, .F. ) ;
#16623=CARTESIAN_POINT ( 'NONE',  ( -1.135272562821019626, 36.50319992234354061, 3.311245368580577164 ) ) ;
#16624=CARTESIAN_POINT ( 'NONE',  ( 2.798362969681409851, 23.50319992234354416, 2.102939460078764977 ) ) ;
#16626=CARTESIAN_POINT ( 'NONE',  ( -0.7188294034286043521, 29.99680007765648071, 2.395093729190366005 ) ) ;
#16628=CARTESIAN_POINT ( 'NONE',  ( -1.444289557195956863, 24.00319992234354416, 4.262301884875733471 ) ) ;
#16633=CARTESIAN_POINT ( 'NONE',  ( 4.481649420246366589, 36.62180007765647360, -1.518615910253458212 ) ) ;
#16642=CARTESIAN_POINT ( 'NONE',  ( -0.05938372350927861171, 16.12180007765647716, -3.680117784833935701 ) ) ;
#16647=CARTESIAN_POINT ( 'NONE',  ( 2.055738996568281518, 33.00319992234354771, -1.423772053676066518 ) ) ;
#16649=CARTESIAN_POINT ( 'NONE',  ( -1.135272562821090014, 33.49680007765648071, -3.311245368580554072 ) ) ;
#16650=CARTESIAN_POINT ( 'NONE',  ( 1.027846397803612311, 23.75319992234354416, 3.346150245485499219 ) ) ;
#16655=CARTESIAN_POINT ( 'NONE',  ( -2.829195390882805139, 20.87180007765647716, -3.793023760679206102 ) ) ;
#16661=CARTESIAN_POINT ( 'NONE',  ( 0.7188294034286049072, 38.74680007765646650, -2.395093729190366005 ) ) ;
#16664=CARTESIAN_POINT ( 'NONE',  ( -3.500000000000000444, 37.99680007765647360, 0.05647727720536892260 ) ) ;
#16666=CARTESIAN_POINT ( 'NONE',  ( -3.982427978483248587, 15.00000000000000355, -0.4169694339699933638 ) ) ;
#16669=CARTESIAN_POINT ( 'NONE',  ( -3.500000000000000444, 27.99680007765648071, 0.05647727720536892260 ) ) ;
#16682=CARTESIAN_POINT ( 'NONE',  ( 2.798362969681366330, 38.99680007765647360, -2.102939460078824929 ) ) ;
#16685=CARTESIAN_POINT ( 'NONE',  ( -2.829195390882724315, 31.62819992234354416, 3.793023760679264722 ) ) ;
#16687=CARTESIAN_POINT ( 'NONE',  ( -2.055738996568281518, 31.75319992234354771, 1.423772053676066962 ) ) ;
#16690=CARTESIAN_POINT ( 'NONE',  ( 1.444289557196047680, 27.24680007765647716, 4.262301884875704161 ) ) ;
#16707=CARTESIAN_POINT ( 'NONE',  ( -3.481649420246370141, 17.87180007765647716, 1.193696214020542268 ) ) ;
#16712=CARTESIAN_POINT ( 'NONE',  ( -2.211161402132839182, 34.12819992234355482, 2.942372952327218627 ) ) ;
#16713=CARTESIAN_POINT ( 'NONE',  ( -3.481649420246394566, 19.62819992234354416, -1.193696214020467883 ) ) ;
#16715=CARTESIAN_POINT ( 'NONE',  ( -1.497042530366477164, 32.62180007765647360, 2.161531897785062384 ) ) ;
#16717=CARTESIAN_POINT ( 'NONE',  ( -2.733110507866328476, 27.37819992234355126, -3.862833514489096398 ) ) ;
#16723=CARTESIAN_POINT ( 'NONE',  ( 1.135272562821090458, 24.74680007765647716, 3.311245368580554072 ) ) ;
#16736=CARTESIAN_POINT ( 'NONE',  ( 0.8262555684460829442, 32.75319992234354061, -2.360188852285421302 ) ) ;
#16738=CARTESIAN_POINT ( 'NONE',  ( 3.518350579753631191, 29.37180007765647005, 1.080741659609802285 ) ) ;
#16740=CARTESIAN_POINT ( 'NONE',  ( -0.05938372350920063936, 28.87819992234353705, 3.680117784833935701 ) ) ;
#16753=CARTESIAN_POINT ( 'NONE',  ( -1.989345975306426206, 35.24680007765648071, 1.515154207786343799 ) ) ;
#16755=CARTESIAN_POINT ( 'NONE',  ( 2.798362969681366330, 36.49680007765648071, -2.102939460078824929 ) ) ;
#16761=CARTESIAN_POINT ( 'NONE',  ( -2.864755990943265829, 23.24680007765647716, -2.011557305968488141 ) ) ;
#16773=CARTESIAN_POINT ( 'NONE',  ( 0.05938372350926800214, 17.37180007765647716, 2.628655560595669183 ) ) ;
#16776=CARTESIAN_POINT ( 'NONE',  ( 3.607379964056363075, 38.50319992234354771, 2.690724712371229010 ) ) ;
#16779=CARTESIAN_POINT ( 'NONE',  ( 0.8262555684460829442, 25.25319992234354771, -2.360188852285421302 ) ) ;
#16783=CARTESIAN_POINT ( 'NONE',  ( -4.481649420246366589, 27.87180007765647716, 1.518615910253458878 ) ) ;
#16800=CARTESIAN_POINT ( 'NONE',  ( 3.518350579753631191, 16.87180007765647360, 1.080741659609802729 ) ) ;
#16802=CARTESIAN_POINT ( 'NONE',  ( 0.05938372350920109732, 35.12819992234354771, -3.680117784833935701 ) ) ;
#16803=CARTESIAN_POINT ( 'NONE',  ( -2.211161402132838738, 19.12819992234354061, 2.942372952327218183 ) ) ;
#16805=CARTESIAN_POINT ( 'NONE',  ( 0.8262555684461332373, 27.24680007765648426, 2.360188852285403982 ) ) ;
#16806=CARTESIAN_POINT ( 'NONE',  ( 4.518350579753602325, 25.62819992234354416, -1.405661355842793725 ) ) ;
#16812=CARTESIAN_POINT ( 'NONE',  ( 2.864755990943265829, 19.49680007765648071, 2.011557305968487697 ) ) ;
#16820=CARTESIAN_POINT ( 'NONE',  ( -2.211161402132902243, 18.37180007765647005, -2.942372952327172886 ) ) ;
#16827=CARTESIAN_POINT ( 'NONE',  ( -2.055738996568281518, 39.25319992234354771, 1.423772053676066962 ) ) ;
#16831=CARTESIAN_POINT ( 'NONE',  ( 0.05938372350927906274, 34.87180007765645939, 3.680117784833935701 ) ) ;
#16833=CARTESIAN_POINT ( 'NONE',  ( 3.518350579753605434, 28.12819992234354416, -1.080741659609877114 ) ) ;
#16844=CARTESIAN_POINT ( 'NONE',  ( 1.497042530366477164, 38.87180007765646650, -2.161531897785062384 ) ) ;
#16846=CARTESIAN_POINT ( 'NONE',  ( 2.864755990943265829, 34.49680007765648071, 2.011557305968487697 ) ) ;
#16848=CARTESIAN_POINT ( 'NONE',  ( -3.432133564730650122, 14.99999999999999822, -1.977182347542568941 ) ) ;
#16853=CARTESIAN_POINT ( 'NONE',  ( -2.115076519116362519, 32.62180007765646650, 3.012182706137107147 ) ) ;
#16865=CARTESIAN_POINT ( 'NONE',  ( 2.115076519116362963, 36.37180007765648782, -3.012182706137107147 ) ) ;
#16868=CARTESIAN_POINT ( 'NONE',  ( 2.829195390882805583, 17.12180007765647716, 3.793023760679204770 ) ) ;
#16870=CARTESIAN_POINT ( 'NONE',  ( 0.05938372350921204690, 35.12819992234354771, -2.628655560595669183 ) ) ;
#16875=CARTESIAN_POINT ( 'NONE',  ( -4.518350579753632523, 33.12180007765647360, -1.405661355842698468 ) ) ;
#16882=CIRCLE ( 'NONE', #12116, 0.5000000000000026645 ) ;
#16892=SURFACE_STYLE_USAGE ( .BOTH. , #11203 ) ;
#16893=CARTESIAN_POINT ( 'NONE',  ( 4.518350579753602325, 20.62819992234354416, -1.405661355842793725 ) ) ;
#16894=CARTESIAN_POINT ( 'NONE',  ( 3.481649420246395010, 18.37819992234354771, 1.193696214020467439 ) ) ;
#16897=CARTESIAN_POINT ( 'NONE',  ( 2.481649420246374138, 34.12180007765647360, -0.8687765177876252132 ) ) ;
#16898=CARTESIAN_POINT ( 'NONE',  ( -4.518350579753602325, 26.87819992234354416, 1.405661355842794391 ) ) ;
#16903=CARTESIAN_POINT ( 'NONE',  ( -3.500000000000000444, 22.99680007765647716, 0.05647727720536892260 ) ) ;
#16911=CARTESIAN_POINT ( 'NONE',  ( -3.481649420246369697, 25.37180007765648071, 1.193696214020542490 ) ) ;
#16918=CARTESIAN_POINT ( 'NONE',  ( -3.500000000000000444, 19.50319992234354416, -0.05647727720529563400 ) ) ;
#16920=CARTESIAN_POINT ( 'NONE',  ( -1.027846397803541700, 34.99680007765648071, 3.346150245485522312 ) ) ;
#16922=CARTESIAN_POINT ( 'NONE',  ( -1.027846397803611866, 27.50319992234354771, -3.346150245485499219 ) ) ;
#16933=CARTESIAN_POINT ( 'NONE',  ( -3.000000000000001332, 15.00000000000000355, 3.048632113068340848E-14 ) ) ;
#16937=CARTESIAN_POINT ( 'NONE',  ( -0.05938372350926768989, 38.62180007765647360, -2.628655560595669183 ) ) ;
#16939=CARTESIAN_POINT ( 'NONE',  ( -3.500000000000000444, 35.49680007765648071, 0.05647727720536892260 ) ) ;
#16940=AXIS2_PLACEMENT_3D ( 'NONE', #9024, #13557, #6428 ) ;
#16944=CARTESIAN_POINT ( 'NONE',  ( 3.500000000000000444, 34.24680007765648071, -0.05647727720536935281 ) ) ;
#16948=COLOUR_RGB ( '',0.8941176470588234615, 0.8941176470588234615, 0.8941176470588234615 ) ;
#16955=CARTESIAN_POINT ( 'NONE',  ( -1.989345975306426206, 17.74680007765647716, 1.515154207786343799 ) ) ;
#16962=CARTESIAN_POINT ( 'NONE',  ( -0.7188294034286550893, 37.50319992234354771, -2.395093729190349130 ) ) ;
#16966=CARTESIAN_POINT ( 'NONE',  ( -3.673772985318219053, 35.74680007765646650, -2.599342558260952174 ) ) ;
#16982=CARTESIAN_POINT ( 'NONE',  ( 4.481649420246397675, 15.87819992234354061, 1.518615910253363177 ) ) ;
#16983=CARTESIAN_POINT ( 'NONE',  ( 3.481649420246395010, 28.37819992234354416, 1.193696214020467439 ) ) ;
#16985=CARTESIAN_POINT ( 'NONE',  ( -2.500000000000001332, 40.49680007765648071, 0.05647727720535858364 ) ) ;
#16987=CARTESIAN_POINT ( 'NONE',  ( 4.481649420246397675, 33.37819992234354771, 1.518615910253363177 ) ) ;
#16993=CARTESIAN_POINT ( 'NONE',  ( -3.481649420246369697, 25.37180007765648071, 1.193696214020542490 ) ) ;
#16998=CARTESIAN_POINT ( 'NONE',  ( 1.336863392178479160, 26.24680007765647716, -4.297206761780677731 ) ) ;
#17005=CARTESIAN_POINT ( 'NONE',  ( 2.211161402132902243, 22.12180007765648071, 2.942372952327172442 ) ) ;
#17011=CARTESIAN_POINT ( 'NONE',  ( 3.500000000000000444, 15.75319992234354416, 0.05647727720529520379 ) ) ;
#17013=CARTESIAN_POINT ( 'NONE',  ( 0.05938372350927906274, 37.37180007765645939, 3.680117784833935701 ) ) ;
#17014=CARTESIAN_POINT ( 'NONE',  ( 3.500000000000000444, 38.25319992234354061, 0.05647727720529520379 ) ) ;
#17024=CARTESIAN_POINT ( 'NONE',  ( -2.607440925699020084, 15.00000000000000533, -1.613633664971267700 ) ) ;
#17027=CARTESIAN_POINT ( 'NONE',  ( 2.481649420246391902, 23.37819992234354771, 0.8687765177875720335 ) ) ;
#17035=CARTESIAN_POINT ( 'NONE',  ( -1.135272562821090014, 28.49680007765648071, -3.311245368580554072 ) ) ;
#17044=CARTESIAN_POINT ( 'NONE',  ( 1.593127413382998903, 22.12180007765648071, 2.091722143975139669 ) ) ;
#17050=CARTESIAN_POINT ( 'NONE',  ( -2.481649420246391902, 34.62819992234354771, -0.8687765177875723666 ) ) ;
#17054=CARTESIAN_POINT ( 'NONE',  ( -2.829195390882805139, 33.37180007765647360, -3.793023760679206102 ) ) ;
#17067=CARTESIAN_POINT ( 'NONE',  ( -2.829195390882724315, 19.12819992234354416, 3.793023760679264722 ) ) ;
#17068=CARTESIAN_POINT ( 'NONE',  ( 3.518350579753606322, 30.62819992234354061, -1.080741659609876892 ) ) ;
#17071=CARTESIAN_POINT ( 'NONE',  ( -2.500000000000001332, 35.49680007765647360, 0.05647727720535858364 ) ) ;
#17073=CARTESIAN_POINT ( 'NONE',  ( -1.336863392178569088, 37.50319992234353350, -4.297206761780648421 ) ) ;
#17079=CARTESIAN_POINT ( 'NONE',  ( 1.027846397803542144, 21.24680007765647716, -3.346150245485522312 ) ) ;
#17083=CARTESIAN_POINT ( 'NONE',  ( -2.829195390882805139, 33.37180007765647360, -3.793023760679206102 ) ) ;
#17087=CARTESIAN_POINT ( 'NONE',  ( -2.798362969681365886, 22.74680007765648071, 2.102939460078824929 ) ) ;
#17093=CARTESIAN_POINT ( 'NONE',  ( -2.115076519116425580, 22.37819992234353350, -3.012182706137062738 ) ) ;
#17095=CARTESIAN_POINT ( 'NONE',  ( 2.115076519116362963, 38.87180007765645939, -3.012182706137107147 ) ) ;
#17097=CARTESIAN_POINT ( 'NONE',  ( -3.481649420246394122, 37.12819992234354771, -1.193696214020467883 ) ) ;
#17111=CARTESIAN_POINT ( 'NONE',  ( -0.8262555684460826111, 21.50319992234354771, 2.360188852285421302 ) ) ;
#17113=CARTESIAN_POINT ( 'NONE',  ( 2.798362969681366330, 18.99680007765648071, -2.102939460078824929 ) ) ;
#17118=CARTESIAN_POINT ( 'NONE',  ( 1.135272562821090458, 32.24680007765648071, 3.311245368580554072 ) ) ;
#17132=CARTESIAN_POINT ( 'NONE',  ( -0.8262555684461330152, 25.99680007765648071, -2.360188852285403982 ) ) ;
#17135=CARTESIAN_POINT ( 'NONE',  ( 1.135272562821090458, 22.24680007765648071, 3.311245368580554072 ) ) ;
#17138=CARTESIAN_POINT ( 'NONE',  ( 0.7188294034286553114, 38.75319992234354061, 2.395093729190349130 ) ) ;
#17141=CARTESIAN_POINT ( 'NONE',  ( -1.336863392178478716, 37.49680007765647360, 4.297206761780677731 ) ) ;
#17163=CARTESIAN_POINT ( 'NONE',  ( -4.499999999999999112, 17.00319992234354416, -0.05647727720528529505 ) ) ;
#17164=CARTESIAN_POINT ( 'NONE',  ( -3.500000000000000444, 32.00319992234354771, -0.05647727720529563400 ) ) ;
#17165=CARTESIAN_POINT ( 'NONE',  ( 2.500000000000001332, 34.24680007765648071, -0.05647727720535888202 ) ) ;
#17167=CARTESIAN_POINT ( 'NONE',  ( -1.336863392178569088, 32.50319992234354771, -4.297206761780648421 ) ) ;
#17174=CARTESIAN_POINT ( 'NONE',  ( -0.05938372350927861171, 31.12180007765647005, -3.680117784833935701 ) ) ;
#17180=CARTESIAN_POINT ( 'NONE',  ( -1.336863392178478716, 34.99680007765647360, 4.297206761780677731 ) ) ;
#17182=EDGE_LOOP ( 'NONE', ( #8037, #17492, #900, #12883, #360 ) ) ;
#17184=CARTESIAN_POINT ( 'NONE',  ( 2.115076519116362963, 26.37180007765648071, -3.012182706137107147 ) ) ;
#17189=CARTESIAN_POINT ( 'NONE',  ( -3.481649420246394122, 19.62819992234354416, -1.193696214020467883 ) ) ;
#17192=CARTESIAN_POINT ( 'NONE',  ( -3.518350579753630747, 35.62180007765648782, -1.080741659609802729 ) ) ;
#17194=CARTESIAN_POINT ( 'NONE',  ( 2.798362969681409851, 36.00319992234354771, 2.102939460078764977 ) ) ;
#17208=CARTESIAN_POINT ( 'NONE',  ( 1.989345975306457071, 21.00319992234354771, 1.515154207786300500 ) ) ;
#17211=CARTESIAN_POINT ( 'NONE',  ( 2.733110507866247652, 18.87180007765647716, -3.862833514489153686 ) ) ;
#17217=CARTESIAN_POINT ( 'NONE',  ( 3.481649420246369697, 31.62180007765647360, -1.193696214020541824 ) ) ;
#17229=CARTESIAN_POINT ( 'NONE',  ( -2.500000000000001332, 20.49680007765648071, 0.05647727720535858364 ) ) ;
#17231=CARTESIAN_POINT ( 'NONE',  ( -2.798362969681365886, 25.24680007765647716, 2.102939460078824929 ) ) ;
#17235=CARTESIAN_POINT ( 'NONE',  ( 2.500000000000001332, 35.75319992234354061, 0.05647727720530566764 ) ) ;
#17238=CARTESIAN_POINT ( 'NONE',  ( 4.481649420246366589, 31.62180007765647716, -1.518615910253458212 ) ) ;
#17258=CARTESIAN_POINT ( 'NONE',  ( 4.518350579753602325, 18.12819992234354416, -1.405661355842793725 ) ) ;
#17259=CARTESIAN_POINT ( 'NONE',  ( -3.481649420246394566, 29.62819992234354061, -1.193696214020467883 ) ) ;
#17260=CARTESIAN_POINT ( 'NONE',  ( -1.593127413382998459, 38.37180007765647360, -2.091722143975139669 ) ) ;
#17263=CARTESIAN_POINT ( 'NONE',  ( -1.444289557195956863, 36.50319992234354061, 4.262301884875733471 ) ) ;
#17269=CARTESIAN_POINT ( 'NONE',  ( -0.05938372350927861171, 33.62180007765648071, -3.680117784833935701 ) ) ;
#17272=CARTESIAN_POINT ( 'NONE',  ( -3.607379964056306676, 27.74680007765648071, 2.690724712371306282 ) ) ;
#17276=CARTESIAN_POINT ( 'NONE',  ( 2.798362969681366330, 28.99680007765647716, -2.102939460078824929 ) ) ;
#17285=CARTESIAN_POINT ( 'NONE',  ( 2.211161402132839626, 22.87819992234354416, -2.942372952327218183 ) ) ;
#17288=CARTESIAN_POINT ( 'NONE',  ( -2.211161402132902243, 35.87180007765648782, -2.942372952327172886 ) ) ;
#17291=CARTESIAN_POINT ( 'NONE',  ( -3.500000000000000444, 37.00319992234354061, -0.05647727720529563400 ) ) ;
#17304=CARTESIAN_POINT ( 'NONE',  ( -1.055125536766255978, 15.00000000000066436, -3.294876966330904544 ) ) ;
#17307=CARTESIAN_POINT ( 'NONE',  ( 1.989345975306457071, 23.50319992234355126, 1.515154207786300500 ) ) ;
#17313=CARTESIAN_POINT ( 'NONE',  ( -2.211161402132902243, 38.37180007765648071, -2.942372952327172886 ) ) ;
#17317=PLANE ( 'NONE',  #11647 ) ;
#17325=CARTESIAN_POINT ( 'NONE',  ( -1.989345975306426206, 22.74680007765647716, 1.515154207786343799 ) ) ;
#17328=CARTESIAN_POINT ( 'NONE',  ( -1.135272562821090014, 20.99680007765647716, -3.311245368580554072 ) ) ;
#17332=CARTESIAN_POINT ( 'NONE',  ( 2.864755990943222308, 18.00319992234354771, -2.011557305968548093 ) ) ;
#17336=CARTESIAN_POINT ( 'NONE',  ( 2.798362969681366330, 16.49680007765647716, -2.102939460078824929 ) ) ;
#17354=CARTESIAN_POINT ( 'NONE',  ( -1.336863392178569088, 30.00319992234354416, -4.297206761780648421 ) ) ;
#17355=CARTESIAN_POINT ( 'NONE',  ( -0.05938372350920064630, 28.87819992234354061, 3.680117784833935701 ) ) ;
#17356=CARTESIAN_POINT ( 'NONE',  ( 2.055738996568281518, 23.00319992234354771, -1.423772053676066518 ) ) ;
#17358=CARTESIAN_POINT ( 'NONE',  ( 1.444289557195957086, 35.25319992234354771, -4.262301884875733471 ) ) ;
#17363=CARTESIAN_POINT ( 'NONE',  ( -2.864755990943265829, 28.24680007765648071, -2.011557305968488141 ) ) ;
#17367=CARTESIAN_POINT ( 'NONE',  ( 3.607379964056306676, 33.99680007765647360, -2.690724712371305838 ) ) ;
#17370=CARTESIAN_POINT ( 'NONE',  ( -2.211161402132902243, 30.87180007765647716, -2.942372952327172886 ) ) ;
#17375=CARTESIAN_POINT ( 'NONE',  ( -3.518350579753605434, 29.37819992234354416, 1.080741659609877781 ) ) ;
#17378=CARTESIAN_POINT ( 'NONE',  ( 2.864755990943265829, 36.99680007765648071, 2.011557305968487697 ) ) ;
#17379=CARTESIAN_POINT ( 'NONE',  ( 2.864755990943222308, 38.00319992234354061, -2.011557305968548093 ) ) ;
#17397=CARTESIAN_POINT ( 'NONE',  ( -1.989345975306457071, 19.75319992234354771, -1.515154207786300944 ) ) ;
#17405=CARTESIAN_POINT ( 'NONE',  ( 3.481649420246369697, 39.12180007765646650, -1.193696214020541824 ) ) ;
#17409=DIRECTION ( 'NONE',  ( 0.000000000000000000, -0.9936001553129346631, -0.1129545544106654864 ) ) ;
#17417=CARTESIAN_POINT ( 'NONE',  ( -1.989345975306426206, 20.24680007765648071, 1.515154207786343799 ) ) ;
#17419=CARTESIAN_POINT ( 'NONE',  ( -3.500000000000000444, 17.99680007765647716, 0.05647727720536892260 ) ) ;
#17425=CARTESIAN_POINT ( 'NONE',  ( -1.135272562821019626, 16.50319992234354416, 3.311245368580577164 ) ) ;
#17428=CARTESIAN_POINT ( 'NONE',  ( 1.027846397803542144, 18.74680007765648071, -3.346150245485522312 ) ) ;
#17447=CARTESIAN_POINT ( 'NONE',  ( 3.607379964056363075, 26.00319992234354771, 2.690724712371229010 ) ) ;
#17448=CARTESIAN_POINT ( 'NONE',  ( 3.500000000000000444, 35.75319992234354771, 0.05647727720529520379 ) ) ;
#17449=CARTESIAN_POINT ( 'NONE',  ( 2.500000000000001332, 18.25319992234354771, 0.05647727720530566764 ) ) ;
#17452=CARTESIAN_POINT ( 'NONE',  ( -1.444289557195956863, 39.00319992234354061, 4.262301884875733471 ) ) ;
#17457=CARTESIAN_POINT ( 'NONE',  ( -2.211161402132902243, 28.37180007765647716, -2.942372952327172886 ) ) ;
#17460=CARTESIAN_POINT ( 'NONE',  ( -2.733110507866247652, 32.62180007765647360, 3.862833514489154574 ) ) ;
#17465=CARTESIAN_POINT ( 'NONE',  ( -2.798362969681365886, 32.74680007765648071, 2.102939460078824929 ) ) ;
#17471=CARTESIAN_POINT ( 'NONE',  ( 1.027846397803612311, 26.25319992234354771, 3.346150245485499219 ) ) ;
#17474=CARTESIAN_POINT ( 'NONE',  ( -0.8262555684461330152, 20.99680007765648071, -2.360188852285403982 ) ) ;
#17475=CARTESIAN_POINT ( 'NONE',  ( -2.829195390882724315, 19.12819992234354416, 3.793023760679264722 ) ) ;
#17492=ORIENTED_EDGE ( 'NONE', *, *, #5322, .F. ) ;
#17494=CARTESIAN_POINT ( 'NONE',  ( 2.481649420246391902, 25.87819992234355126, 0.8687765177875720335 ) ) ;
#17497=CARTESIAN_POINT ( 'NONE',  ( -0.05938372350927861171, 21.12180007765648071, -3.680117784833935701 ) ) ;
#17502=CARTESIAN_POINT ( 'NONE',  ( -1.027846397803541700, 37.49680007765647360, 3.346150245485522312 ) ) ;
#17515=CARTESIAN_POINT ( 'NONE',  ( 2.500000000000001332, 29.24680007765648071, -0.05647727720535888202 ) ) ;
#17517=CARTESIAN_POINT ( 'NONE',  ( 1.027846397803542144, 18.74680007765648071, -3.346150245485522312 ) ) ;
#17523=CARTESIAN_POINT ( 'NONE',  ( -3.500000000000000444, 17.00319992234354416, -0.05647727720529563400 ) ) ;
#17527=CARTESIAN_POINT ( 'NONE',  ( -1.027846397803541700, 19.99680007765648071, 3.346150245485522312 ) ) ;
#17544=CARTESIAN_POINT ( 'NONE',  ( 0.05938372350919016857, 25.12819992234354416, -4.731580009072201776 ) ) ;
#17546=CARTESIAN_POINT ( 'NONE',  ( 1.027846397803612311, 33.75319992234354771, 3.346150245485499219 ) ) ;
#17547=CARTESIAN_POINT ( 'NONE',  ( 1.497042530366522461, 18.62819992234354771, 2.161531897785029965 ) ) ;
#17550=CARTESIAN_POINT ( 'NONE',  ( -3.607379964056306676, 20.24680007765648071, 2.690724712371306282 ) ) ;
#17554=CARTESIAN_POINT ( 'NONE',  ( -1.027846397803541700, 34.99680007765648071, 3.346150245485522312 ) ) ;
#17564=CARTESIAN_POINT ( 'NONE',  ( -1.135272562821019626, 29.00319992234354416, 3.311245368580577164 ) ) ;
#17567=CARTESIAN_POINT ( 'NONE',  ( 0.05938372350926800214, 19.87180007765648426, 2.628655560595669183 ) ) ;
#17570=CARTESIAN_POINT ( 'NONE',  ( -3.607379964056363075, 19.75319992234354416, -2.690724712371229899 ) ) ;
#17591=CARTESIAN_POINT ( 'NONE',  ( -1.593127413382952939, 31.62819992234354416, 2.091722143975172532 ) ) ;
#17594=CARTESIAN_POINT ( 'NONE',  ( -2.211161402132902243, 25.87180007765647360, -2.942372952327172886 ) ) ;
#17609=DIRECTION ( 'NONE',  ( -1.000000000000000000, 0.000000000000000000, 1.053778523157998394E-14 ) ) ;
#17610=CARTESIAN_POINT ( 'NONE',  ( 1.989345975306426206, 28.99680007765648071, -1.515154207786343799 ) ) ;
#17612=CARTESIAN_POINT ( 'NONE',  ( 1.027846397803542144, 28.74680007765647716, -3.346150245485522312 ) ) ;
#17617=CARTESIAN_POINT ( 'NONE',  ( -1.135272562821019626, 21.50319992234354416, 3.311245368580577164 ) ) ;
#17620=CARTESIAN_POINT ( 'NONE',  ( -2.211161402132902243, 15.87180007765647716, -2.942372952327172886 ) ) ;
#17641=CARTESIAN_POINT ( 'NONE',  ( -4.499999999999999112, 27.00319992234355126, -0.05647727720528529505 ) ) ;
#17642=CARTESIAN_POINT ( 'NONE',  ( -0.05938372350920064630, 38.87819992234354061, 3.680117784833935701 ) ) ;
#17643=CARTESIAN_POINT ( 'NONE',  ( 2.055738996568281518, 18.00319992234354416, -1.423772053676066518 ) ) ;
#17645=CARTESIAN_POINT ( 'NONE',  ( 3.607379964056363075, 38.50319992234354771, 2.690724712371229010 ) ) ;
#17649=CARTESIAN_POINT ( 'NONE',  ( -1.135272562821090014, 35.99680007765648071, -3.311245368580554072 ) ) ;
#17660=CARTESIAN_POINT ( 'NONE',  ( 3.500000000000000444, 25.75319992234354771, 0.05647727720529520379 ) ) ;
#17661=CARTESIAN_POINT ( 'NONE',  ( 3.481649420246395010, 15.87819992234354416, 1.193696214020467439 ) ) ;
#17663=CARTESIAN_POINT ( 'NONE',  ( -1.989345975306426206, 25.24680007765648071, 1.515154207786343799 ) ) ;
#17664=CARTESIAN_POINT ( 'NONE',  ( -3.518350579753605434, 39.37819992234354771, 1.080741659609877781 ) ) ;
#17668=CARTESIAN_POINT ( 'NONE',  ( 4.518350579753633411, 39.37180007765647360, 1.405661355842698468 ) ) ;
#17679=CARTESIAN_POINT ( 'NONE',  ( 2.481649420246391902, 30.87819992234354416, 0.8687765177875720335 ) ) ;
#17681=CARTESIAN_POINT ( 'NONE',  ( 1.135272562821090458, 22.24680007765648071, 3.311245368580554072 ) ) ;
#17694=CARTESIAN_POINT ( 'NONE',  ( -3.500000000000000000, 15.00000000000000355, 3.564992268403899267E-14 ) ) ;
#17695=CARTESIAN_POINT ( 'NONE',  ( 1.593127413382998903, 32.12180007765648071, 2.091722143975139669 ) ) ;
#17698=CARTESIAN_POINT ( 'NONE',  ( -1.027846397803541700, 29.99680007765648071, 3.346150245485522312 ) ) ;
#17705=CARTESIAN_POINT ( 'NONE',  ( 2.798362969681366330, 18.99680007765648071, -2.102939460078824929 ) ) ;
#17723=CARTESIAN_POINT ( 'NONE',  ( 1.444289557195957086, 27.75319992234354416, -4.262301884875733471 ) ) ;
#17724=CARTESIAN_POINT ( 'NONE',  ( -3.518350579753606322, 39.37819992234354771, 1.080741659609877781 ) ) ;
#17725=CARTESIAN_POINT ( 'NONE',  ( -1.497042530366522461, 22.37819992234354416, -2.161531897785030409 ) ) ;
#17727=CARTESIAN_POINT ( 'NONE',  ( 1.444289557196047680, 17.24680007765648071, 4.262301884875704161 ) ) ;
#17735=CARTESIAN_POINT ( 'NONE',  ( -2.864755990943265829, 38.24680007765647360, -2.011557305968488141 ) ) ;
#17749=CARTESIAN_POINT ( 'NONE',  ( -2.798362969681409851, 29.75319992234354416, -2.102939460078765421 ) ) ;
#17753=CARTESIAN_POINT ( 'NONE',  ( 0.8262555684461332373, 19.74680007765648071, 2.360188852285403982 ) ) ;
#17755=CARTESIAN_POINT ( 'NONE',  ( 4.499999999999999112, 20.75319992234354416, 0.05647727720528474687 ) ) ;
#17759=CARTESIAN_POINT ( 'NONE',  ( 3.481649420246369697, 16.62180007765648071, -1.193696214020541824 ) ) ;
#17772=CARTESIAN_POINT ( 'NONE',  ( -1.593127413382952939, 29.12819992234354416, 2.091722143975172532 ) ) ;
#17775=CARTESIAN_POINT ( 'NONE',  ( 0.05938372350927906274, 19.87180007765648426, 3.680117784833935701 ) ) ;
#17789=CARTESIAN_POINT ( 'NONE',  ( -2.481649420246374138, 32.87180007765648071, 0.8687765177876256573 ) ) ;
#17792=CARTESIAN_POINT ( 'NONE',  ( 2.864755990943265829, 29.49680007765647716, 2.011557305968487697 ) ) ;
#17799=CARTESIAN_POINT ( 'NONE',  ( -2.211161402132902243, 23.37180007765647716, -2.942372952327172886 ) ) ;
#17812=CARTESIAN_POINT ( 'NONE',  ( 0.05938372350927906274, 34.87180007765645939, 3.680117784833935701 ) ) ;
#17816=CARTESIAN_POINT ( 'NONE',  ( -1.336863392178569088, 32.50319992234354771, -4.297206761780648421 ) ) ;
#17817=CARTESIAN_POINT ( 'NONE',  ( -2.798362969681409851, 37.25319992234354061, -2.102939460078765421 ) ) ;
#17818=CARTESIAN_POINT ( 'NONE',  ( -0.05938372350921170689, 26.37819992234355126, 2.628655560595669183 ) ) ;
#17820=CARTESIAN_POINT ( 'NONE',  ( -3.673772985318219053, 18.24680007765647716, -2.599342558260952174 ) ) ;
#17824=CARTESIAN_POINT ( 'NONE',  ( -1.027846397803541700, 37.49680007765647360, 3.346150245485522312 ) ) ;
#17835=CARTESIAN_POINT ( 'NONE',  ( -2.115076519116425580, 37.37819992234352640, -3.012182706137062738 ) ) ;
#17836=CARTESIAN_POINT ( 'NONE',  ( -1.041744090737314776, 15.00160208984915755, -3.341881251993961133 ) ) ;
#17838=CARTESIAN_POINT ( 'NONE',  ( 2.055738996568313048, 24.49680007765648426, 1.423772053676023441 ) ) ;
#17840=CARTESIAN_POINT ( 'NONE',  ( -2.864755990943222308, 39.25319992234354771, 2.011557305968548093 ) ) ;
#17844=CARTESIAN_POINT ( 'NONE',  ( 2.115076519116362963, 16.37180007765647716, -3.012182706137107147 ) ) ;
#17858=CARTESIAN_POINT ( 'NONE',  ( -2.518350579753611207, 34.37819992234354771, 0.7558219633769609480 ) ) ;
#17861=CARTESIAN_POINT ( 'NONE',  ( -1.027846397803541700, 22.49680007765648071, 3.346150245485522312 ) ) ;
#17867=CARTESIAN_POINT ( 'NONE',  ( -4.499999999999999112, 25.49680007765647716, 0.05647727720537927543 ) ) ;
#17874=CARTESIAN_POINT ( 'NONE',  ( 2.481649420246374138, 31.62180007765648426, -0.8687765177876252132 ) ) ;
#17876=CARTESIAN_POINT ( 'NONE',  ( 3.500000000000000444, 29.24680007765647716, -0.05647727720536935281 ) ) ;
#17882=ADVANCED_FACE ( 'NONE', ( #3118 ), #239, .T. ) ;
#17883=CARTESIAN_POINT ( 'NONE',  ( -1.027846397803541700, 22.49680007765648071, 3.346150245485522312 ) ) ;
#17894=CARTESIAN_POINT ( 'NONE',  ( 3.481649420246369697, 31.62180007765647360, -1.193696214020541824 ) ) ;
#17900=CARTESIAN_POINT ( 'NONE',  ( 3.673772985318163098, 30.50319992234354416, -2.599342558261029001 ) ) ;
#17902=CARTESIAN_POINT ( 'NONE',  ( 0.8262555684460829442, 30.25319992234354771, -2.360188852285421302 ) ) ;
#17906=CARTESIAN_POINT ( 'NONE',  ( 1.336863392178479160, 23.74680007765647716, -4.297206761780677731 ) ) ;
#17911=CARTESIAN_POINT ( 'NONE',  ( -2.115076519116362519, 35.12180007765645939, 3.012182706137107147 ) ) ;
#17919=CARTESIAN_POINT ( 'NONE',  ( 2.211161402132902243, 17.12180007765647360, 2.942372952327172442 ) ) ;
#17922=CARTESIAN_POINT ( 'NONE',  ( -3.481649420246394122, 34.62819992234354771, -1.193696214020467883 ) ) ;
#17926=CARTESIAN_POINT ( 'NONE',  ( 0.8262555684461332373, 32.24680007765648071, 2.360188852285403982 ) ) ;
#17927=CARTESIAN_POINT ( 'NONE',  ( -2.733110507866328476, 22.37819992234354416, -3.862833514489096398 ) ) ;
#17932=CARTESIAN_POINT ( 'NONE',  ( -2.211161402132902243, 15.87180007765647716, -2.942372952327172886 ) ) ;
#17940=CARTESIAN_POINT ( 'NONE',  ( 3.518350579753631191, 19.37180007765648071, 1.080741659609802285 ) ) ;
#17944=CARTESIAN_POINT ( 'NONE',  ( 1.989345975306457071, 36.00319992234354771, 1.515154207786300500 ) ) ;
#17947=CARTESIAN_POINT ( 'NONE',  ( -2.864755990943265829, 28.24680007765648071, -2.011557305968488141 ) ) ;
#17948=CARTESIAN_POINT ( 'NONE',  ( -0.05938372350920063936, 16.37819992234354416, 3.680117784833935701 ) ) ;
#17955=CARTESIAN_POINT ( 'NONE',  ( -3.607379964056306676, 22.74680007765647716, 2.690724712371306282 ) ) ;
#17965=CARTESIAN_POINT ( 'NONE',  ( 2.518350579753628971, 36.87180007765648071, 0.7558219633769073242 ) ) ;
#17967=CARTESIAN_POINT ( 'NONE',  ( -1.027846397803541700, 37.49680007765647360, 3.346150245485522312 ) ) ;
#17970=CARTESIAN_POINT ( 'NONE',  ( -3.052806949544935478, 15.00000000000000888, -2.471371977836584133 ) ) ;
#17975=CARTESIAN_POINT ( 'NONE',  ( -2.211161402132902243, 20.87180007765647716, -2.942372952327172886 ) ) ;
#17987=CARTESIAN_POINT ( 'NONE',  ( -2.500000000000001332, 15.49680007765647893, 0.05647727720535858364 ) ) ;
#17992=CARTESIAN_POINT ( 'NONE',  ( -3.607379964056363075, 34.75319992234354771, -2.690724712371229899 ) ) ;
#17995=CARTESIAN_POINT ( 'NONE',  ( -0.8262555684460826111, 29.00319992234355482, 2.360188852285421302 ) ) ;
#17998=CARTESIAN_POINT ( 'NONE',  ( -3.607379964056306676, 25.24680007765648071, 2.690724712371306282 ) ) ;
#18013=CARTESIAN_POINT ( 'NONE',  ( -2.864755990943222308, 36.75319992234354061, 2.011557305968548093 ) ) ;
#18014=CARTESIAN_POINT ( 'NONE',  ( -3.500000000000000444, 19.50319992234354416, -0.05647727720529563400 ) ) ;
#18016=CARTESIAN_POINT ( 'NONE',  ( 0.7188294034286049072, 31.24680007765648071, -2.395093729190366005 ) ) ;
#18018=CARTESIAN_POINT ( 'NONE',  ( 2.829195390882724759, 22.87819992234354416, -3.793023760679264278 ) ) ;
#18023=CARTESIAN_POINT ( 'NONE',  ( -4.499999999999999112, 35.49680007765647360, 0.05647727720537927543 ) ) ;
#18035=FACE_OUTER_BOUND ( 'NONE', #13071, .T. ) ;
#18040=CARTESIAN_POINT ( 'NONE',  ( 2.055738996568281518, 35.50319992234354771, -1.423772053676066518 ) ) ;
#18042=CARTESIAN_POINT ( 'NONE',  ( 1.027846397803542144, 28.74680007765647716, -3.346150245485522312 ) ) ;
#18043=CARTESIAN_POINT ( 'NONE',  ( -3.481649420246394122, 29.62819992234353350, -1.193696214020467883 ) ) ;
#18051=CARTESIAN_POINT ( 'NONE',  ( -4.499999999999999112, 20.49680007765647716, 0.05647727720537927543 ) ) ;
#18059=CARTESIAN_POINT ( 'NONE',  ( -1.497042530366477164, 37.62180007765646650, 2.161531897785062384 ) ) ;
#18061=CARTESIAN_POINT ( 'NONE',  ( -2.798362969681365886, 40.24680007765648071, 2.102939460078824929 ) ) ;
#18064=CARTESIAN_POINT ( 'NONE',  ( -4.000000000000000000, 15.00000000000000355, 4.083367561434192880E-14 ) ) ;
#18067=CARTESIAN_POINT ( 'NONE',  ( 2.211161402132902243, 24.62180007765647716, 2.942372952327172442 ) ) ;
#18080=CARTESIAN_POINT ( 'NONE',  ( -1.027846397803541700, 39.99680007765648071, 3.346150245485522312 ) ) ;
#18085=CARTESIAN_POINT ( 'NONE',  ( -2.733110507866328476, 34.87819992234354771, -3.862833514489096398 ) ) ;
#18090=CARTESIAN_POINT ( 'NONE',  ( -0.05938372350921170689, 31.37819992234354061, 2.628655560595669183 ) ) ;
#18093=CARTESIAN_POINT ( 'NONE',  ( 3.673772985318219053, 21.99680007765647716, 2.599342558260951730 ) ) ;
#18110=CARTESIAN_POINT ( 'NONE',  ( 1.135272562821020070, 32.75319992234354771, -3.311245368580577164 ) ) ;
#18111=CARTESIAN_POINT ( 'NONE',  ( -2.115076519116425580, 19.87819992234354416, -3.012182706137063182 ) ) ;
#18113=CARTESIAN_POINT ( 'NONE',  ( 2.481649420246374138, 26.62180007765648426, -0.8687765177876252132 ) ) ;
#18115=CARTESIAN_POINT ( 'NONE',  ( -4.481649420246396787, 22.12819992234354416, -1.518615910253363399 ) ) ;
#18121=CARTESIAN_POINT ( 'NONE',  ( -0.05938372350927861171, 21.12180007765648071, -3.680117784833935701 ) ) ;
#18130=CARTESIAN_POINT ( 'NONE',  ( 1.027846397803542144, 18.74680007765648071, -3.346150245485522312 ) ) ;
#18136=CARTESIAN_POINT ( 'NONE',  ( -0.05938372350921170689, 38.87819992234354771, 2.628655560595669183 ) ) ;
#18138=CARTESIAN_POINT ( 'NONE',  ( 0.05938372350927906274, 32.37180007765647360, 3.680117784833935701 ) ) ;
#18140=CARTESIAN_POINT ( 'NONE',  ( 2.211161402132839626, 25.37819992234353705, -2.942372952327218183 ) ) ;
#18152=CARTESIAN_POINT ( 'NONE',  ( 2.055738996568313048, 39.49680007765648071, 1.423772053676023441 ) ) ;
#18154=CARTESIAN_POINT ( 'NONE',  ( -2.211161402132901799, 38.37180007765647360, -2.942372952327172886 ) ) ;
#18155=CARTESIAN_POINT ( 'NONE',  ( -1.165965068879164734, 15.00000000000001421, -3.401582918303170278 ) ) ;
#18160=CARTESIAN_POINT ( 'NONE',  ( 0.05938372350927906274, 24.87180007765647005, 3.680117784833935701 ) ) ;
#18173=CARTESIAN_POINT ( 'NONE',  ( -0.05938372350926768989, 16.12180007765648071, -2.628655560595669183 ) ) ;
#18176=CARTESIAN_POINT ( 'NONE',  ( -4.481649420246366589, 17.87180007765647360, 1.518615910253458878 ) ) ;
#18178=CARTESIAN_POINT ( 'NONE',  ( 0.8262555684460829442, 27.75319992234355126, -2.360188852285421302 ) ) ;
#18181=CARTESIAN_POINT ( 'NONE',  ( 1.444289557196047680, 22.24680007765647716, 4.262301884875704161 ) ) ;
#18204=CARTESIAN_POINT ( 'NONE',  ( 3.481649420246394122, 38.37819992234354771, 1.193696214020467439 ) ) ;
#18205=CARTESIAN_POINT ( 'NONE',  ( 1.027846397803612311, 16.25319992234354416, 3.346150245485499219 ) ) ;
#18207=CARTESIAN_POINT ( 'NONE',  ( 2.518350579753628971, 26.87180007765648426, 0.7558219633769073242 ) ) ;
#18208=CARTESIAN_POINT ( 'NONE',  ( -4.499999999999999112, 29.50319992234354061, -0.05647727720528529505 ) ) ;
#18212=CARTESIAN_POINT ( 'NONE',  ( 0.05938372350927906274, 22.37180007765648071, 3.680117784833935701 ) ) ;
#18224=CARTESIAN_POINT ( 'NONE',  ( 0.7188294034286553114, 38.75319992234354061, 2.395093729190349130 ) ) ;
#18226=CARTESIAN_POINT ( 'NONE',  ( -0.05938372350927861171, 28.62180007765648071, -3.680117784833935701 ) ) ;
#18228=CARTESIAN_POINT ( 'NONE',  ( -1.135272562821019626, 26.50319992234354771, 3.311245368580577164 ) ) ;
#18238=CARTESIAN_POINT ( 'NONE',  ( 2.500000000000001332, 15.75319992234354594, 0.05647727720530566764 ) ) ;
#18240=CARTESIAN_POINT ( 'NONE',  ( 1.135272562821090458, 34.74680007765648071, 3.311245368580554072 ) ) ;
#18247=CARTESIAN_POINT ( 'NONE',  ( 3.518350579753631191, 29.37180007765647005, 1.080741659609802285 ) ) ;
#18259=CARTESIAN_POINT ( 'NONE',  ( -2.798362969681365886, 40.24680007765648071, 2.102939460078824929 ) ) ;
#18262=CARTESIAN_POINT ( 'NONE',  ( 2.733110507866247652, 16.37180007765647716, -3.862833514489153686 ) ) ;
#18265=CARTESIAN_POINT ( 'NONE',  ( 1.989345975306457071, 33.50319992234354061, 1.515154207786300500 ) ) ;
#18268=CARTESIAN_POINT ( 'NONE',  ( -2.829195390882805139, 23.37180007765647716, -3.793023760679206102 ) ) ;
#18283=CARTESIAN_POINT ( 'NONE',  ( -4.518350579753602325, 19.37819992234354061, 1.405661355842794391 ) ) ;
#18284=CARTESIAN_POINT ( 'NONE',  ( -3.500000000000000444, 22.00319992234354416, -0.05647727720529563400 ) ) ;
#18286=CARTESIAN_POINT ( 'NONE',  ( 2.518350579753611207, 15.62819992234354594, -0.7558219633769606149 ) ) ;
#18288=CARTESIAN_POINT ( 'NONE',  ( 2.733110507866328920, 23.62819992234354416, 3.862833514489095510 ) ) ;
#18296=CARTESIAN_POINT ( 'NONE',  ( -1.135272562821090014, 20.99680007765647716, -3.311245368580554072 ) ) ;
#18305=CARTESIAN_POINT ( 'NONE',  ( -2.864755990943265829, 25.74680007765647716, -2.011557305968488141 ) ) ;
#18312=CARTESIAN_POINT ( 'NONE',  ( 1.027846397803612311, 18.75319992234354771, 3.346150245485499219 ) ) ;
#18315=CARTESIAN_POINT ( 'NONE',  ( -1.135272562821090014, 28.49680007765648071, -3.311245368580554072 ) ) ;
#18316=CARTESIAN_POINT ( 'NONE',  ( 1.135272562821020070, 25.25319992234354416, -3.311245368580577164 ) ) ;
#18331=CARTESIAN_POINT ( 'NONE',  ( -2.500000000000001332, 37.99680007765646650, 0.05647727720535858364 ) ) ;
#18333=CARTESIAN_POINT ( 'NONE',  ( 3.518350579753631191, 36.87180007765647360, 1.080741659609802729 ) ) ;
#18339=CARTESIAN_POINT ( 'NONE',  ( -3.518350579753630747, 33.12180007765646650, -1.080741659609802729 ) ) ;
#18351=CARTESIAN_POINT ( 'NONE',  ( -1.593127413382998459, 15.87180007765648071, -2.091722143975139669 ) ) ;
#18356=CARTESIAN_POINT ( 'NONE',  ( -0.8262555684460826111, 34.00319992234354771, 2.360188852285421302 ) ) ;
#18361=CARTESIAN_POINT ( 'NONE',  ( -2.733110507866247652, 35.12180007765647360, 3.862833514489154574 ) ) ;
#18369=CARTESIAN_POINT ( 'NONE',  ( -0.05938372350926768989, 38.62180007765647360, -2.628655560595669183 ) ) ;
#18404=COLOUR_RGB('Grey',0.48,0.52,0.57);
#18405=FILL_AREA_STYLE_COLOUR('',#18404);
#18406=FILL_AREA_STYLE('',(#18405));
#18407=SURFACE_STYLE_FILL_AREA(#18406);
#18408=SURFACE_SIDE_STYLE('',(#18407));
#18409=SURFACE_STYLE_USAGE(.BOTH.,#18408);
#18410=PRESENTATION_STYLE_ASSIGNMENT((#18409));
ENDSEC;
END-ISO-10303-21;
